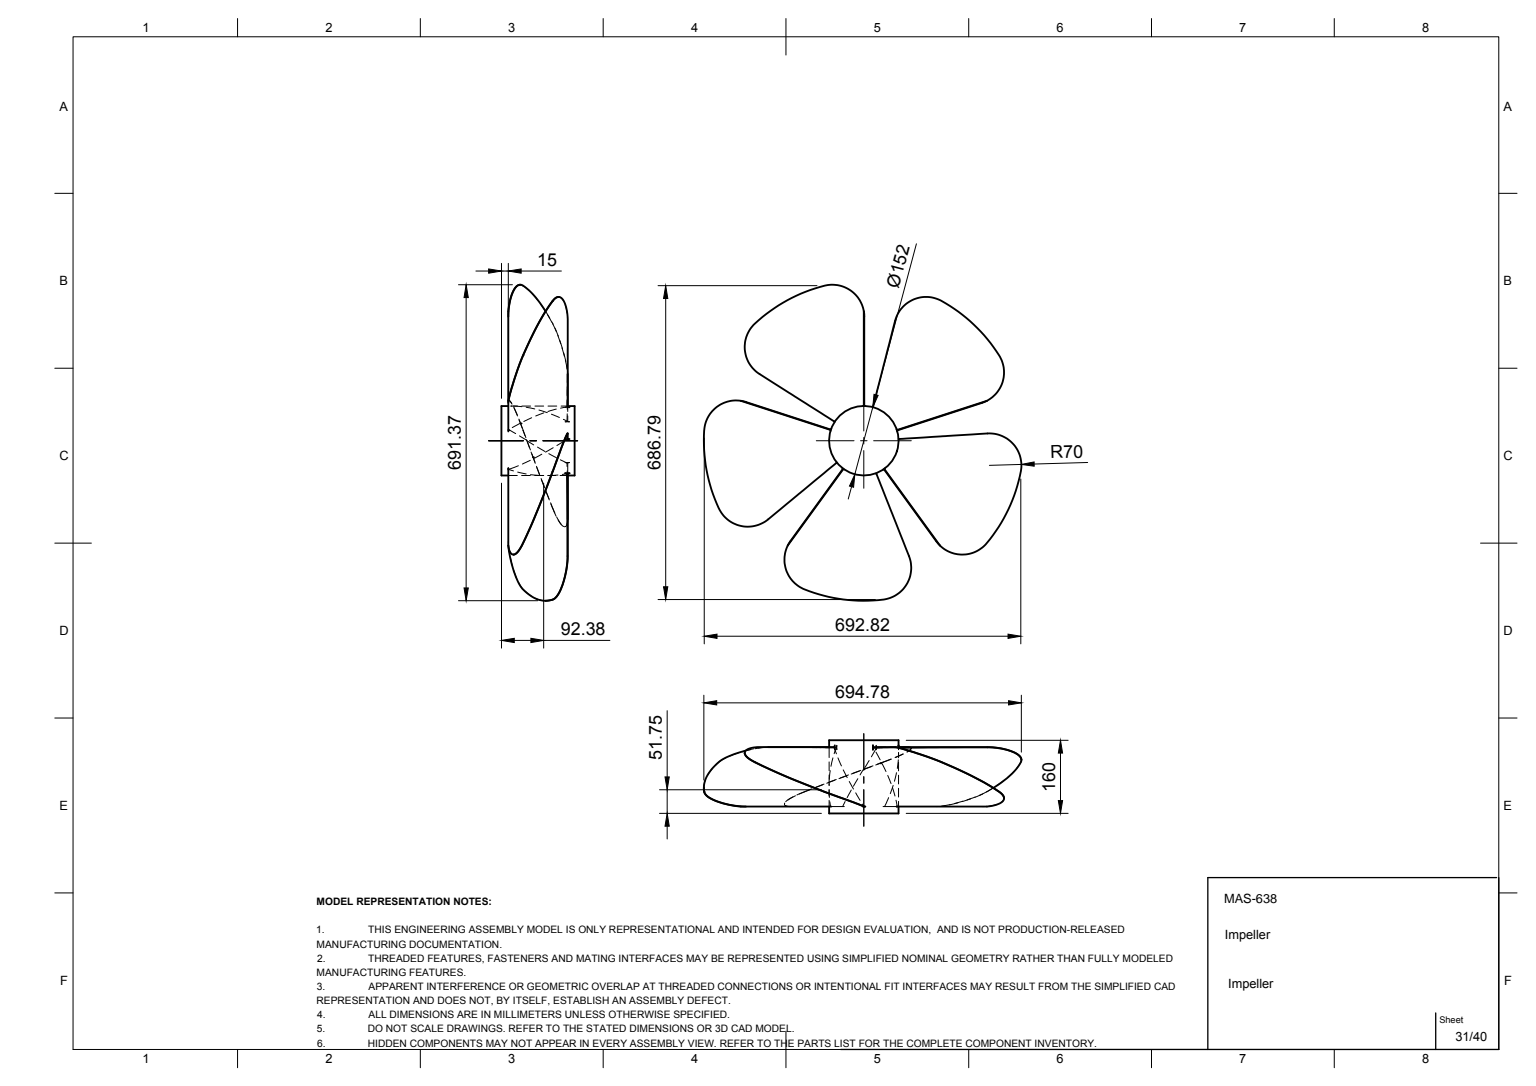
ISO-10303-21;
HEADER;
FILE_DESCRIPTION((''),'2;1');
FILE_NAME('Impeller.step','2026-10-09T12:00:21-07:00',(''),(''),'','','');
FILE_SCHEMA (('AUTOMOTIVE_DESIGN { 1 0 10303 214 3 1 1 }'));
ENDSEC;
DATA;
#10=MECHANICAL_DESIGN_GEOMETRIC_PRESENTATION_REPRESENTATION('',(#428),#10334);
#11=(
BOUNDED_CURVE()
B_SPLINE_CURVE(2,(#6661,#6662,#6663,#6664,#6665,#6666,#6667,#6668,#6669,
#6670,#6671,#6672,#6673,#6674,#6675),.UNSPECIFIED.,.F.,.F.)
B_SPLINE_CURVE_WITH_KNOTS((3,2,2,2,2,2,2,3),(0.24767599272402,0.275737101138962,
0.367649468185283,0.459561835231604,0.551474202277924,0.643386569324245,
0.735298936370566,0.744991303101576),.UNSPECIFIED.)
CURVE()
GEOMETRIC_REPRESENTATION_ITEM()
RATIONAL_B_SPLINE_CURVE((0.999547382800022,0.999674234156792,1.,0.998932974802372,
1.,0.998932974802372,1.,0.998932974802372,1.,0.998932974802372,1.,0.998932974802372,
1.,0.999887479782547,0.999798690587312))
REPRESENTATION_ITEM('')
) ;
#12=(
BOUNDED_CURVE()
B_SPLINE_CURVE(2,(#6842,#6843,#6844,#6845,#6846,#6847,#6848,#6849,#6850,
#6851,#6852,#6853,#6854,#6855,#6856),.UNSPECIFIED.,.F.,.F.)
B_SPLINE_CURVE_WITH_KNOTS((3,2,2,2,2,2,2,3),(0.0400825883740044,0.0441176470588235,
0.0588235294117647,0.0735294117647059,0.0882352941176471,0.102941176470588,
0.117647058823529,0.119652613204452),.UNSPECIFIED.)
CURVE()
GEOMETRIC_REPRESENTATION_ITEM()
RATIONAL_B_SPLINE_CURVE((0.999575116080077,0.999707225368239,1.,0.998932974802372,
1.,0.998932974802372,1.,0.998932974802372,1.,0.998932974802372,1.,0.998932974802372,
1.,0.999854481559943,0.999748654059601))
REPRESENTATION_ITEM('')
) ;
#13=(
BOUNDED_CURVE()
B_SPLINE_CURVE(2,(#7299,#7300,#7301,#7302,#7303,#7304,#7305,#7306,#7307,
#7308,#7309,#7310,#7311,#7312,#7313),.UNSPECIFIED.,.F.,.F.)
B_SPLINE_CURVE_WITH_KNOTS((3,2,2,2,2,2,2,3),(0.24767599272402,0.275737101138962,
0.367649468185283,0.459561835231604,0.551474202277924,0.643386569324245,
0.735298936370566,0.744991303101576),.UNSPECIFIED.)
CURVE()
GEOMETRIC_REPRESENTATION_ITEM()
RATIONAL_B_SPLINE_CURVE((0.999547382800022,0.999674234156792,1.,0.998932974802372,
1.,0.998932974802372,1.,0.998932974802372,1.,0.998932974802372,1.,0.998932974802372,
1.,0.999887479782547,0.999798690587312))
REPRESENTATION_ITEM('')
) ;
#14=(
BOUNDED_CURVE()
B_SPLINE_CURVE(2,(#7480,#7481,#7482,#7483,#7484,#7485,#7486,#7487,#7488,
#7489,#7490,#7491,#7492,#7493,#7494),.UNSPECIFIED.,.F.,.F.)
B_SPLINE_CURVE_WITH_KNOTS((3,2,2,2,2,2,2,3),(0.0400825883740044,0.0441176470588235,
0.0588235294117647,0.0735294117647059,0.0882352941176471,0.102941176470588,
0.117647058823529,0.119652613204452),.UNSPECIFIED.)
CURVE()
GEOMETRIC_REPRESENTATION_ITEM()
RATIONAL_B_SPLINE_CURVE((0.999575116080077,0.999707225368239,1.,0.998932974802372,
1.,0.998932974802372,1.,0.998932974802372,1.,0.998932974802372,1.,0.998932974802372,
1.,0.999854481559943,0.999748654059601))
REPRESENTATION_ITEM('')
) ;
#15=(
BOUNDED_CURVE()
B_SPLINE_CURVE(2,(#7937,#7938,#7939,#7940,#7941,#7942,#7943,#7944,#7945,
#7946,#7947,#7948,#7949,#7950,#7951),.UNSPECIFIED.,.F.,.F.)
B_SPLINE_CURVE_WITH_KNOTS((3,2,2,2,2,2,2,3),(0.24767599272402,0.275737101138962,
0.367649468185283,0.459561835231604,0.551474202277924,0.643386569324245,
0.735298936370566,0.744991303101576),.UNSPECIFIED.)
CURVE()
GEOMETRIC_REPRESENTATION_ITEM()
RATIONAL_B_SPLINE_CURVE((0.999547382800022,0.999674234156792,1.,0.998932974802372,
1.,0.998932974802372,1.,0.998932974802372,1.,0.998932974802372,1.,0.998932974802372,
1.,0.999887479782547,0.999798690587312))
REPRESENTATION_ITEM('')
) ;
#16=(
BOUNDED_CURVE()
B_SPLINE_CURVE(2,(#8118,#8119,#8120,#8121,#8122,#8123,#8124,#8125,#8126,
#8127,#8128,#8129,#8130,#8131,#8132),.UNSPECIFIED.,.F.,.F.)
B_SPLINE_CURVE_WITH_KNOTS((3,2,2,2,2,2,2,3),(0.0400825883740044,0.0441176470588235,
0.0588235294117647,0.0735294117647059,0.0882352941176471,0.102941176470588,
0.117647058823529,0.119652613204452),.UNSPECIFIED.)
CURVE()
GEOMETRIC_REPRESENTATION_ITEM()
RATIONAL_B_SPLINE_CURVE((0.999575116080077,0.999707225368239,1.,0.998932974802372,
1.,0.998932974802372,1.,0.998932974802372,1.,0.998932974802372,1.,0.998932974802372,
1.,0.999854481559943,0.999748654059601))
REPRESENTATION_ITEM('')
) ;
#17=(
BOUNDED_CURVE()
B_SPLINE_CURVE(2,(#8574,#8575,#8576,#8577,#8578,#8579,#8580,#8581,#8582,
#8583,#8584,#8585,#8586,#8587,#8588),.UNSPECIFIED.,.F.,.F.)
B_SPLINE_CURVE_WITH_KNOTS((3,2,2,2,2,2,2,3),(0.24767599272402,0.275737101138962,
0.367649468185283,0.459561835231603,0.551474202277924,0.643386569324245,
0.735298936370566,0.744991303101576),.UNSPECIFIED.)
CURVE()
GEOMETRIC_REPRESENTATION_ITEM()
RATIONAL_B_SPLINE_CURVE((0.999547382800022,0.999674234156792,1.,0.998932974802372,
1.,0.998932974802372,1.,0.998932974802372,1.,0.998932974802372,1.,0.998932974802372,
1.,0.999887479782547,0.999798690587312))
REPRESENTATION_ITEM('')
) ;
#18=(
BOUNDED_CURVE()
B_SPLINE_CURVE(2,(#8755,#8756,#8757,#8758,#8759,#8760,#8761,#8762,#8763,
#8764,#8765,#8766,#8767,#8768,#8769),.UNSPECIFIED.,.F.,.F.)
B_SPLINE_CURVE_WITH_KNOTS((3,2,2,2,2,2,2,3),(0.0400825883740044,0.0441176470588235,
0.0588235294117647,0.0735294117647059,0.0882352941176471,0.102941176470588,
0.117647058823529,0.119652613204452),.UNSPECIFIED.)
CURVE()
GEOMETRIC_REPRESENTATION_ITEM()
RATIONAL_B_SPLINE_CURVE((0.999575116080077,0.999707225368239,1.,0.998932974802372,
1.,0.998932974802372,1.,0.998932974802372,1.,0.998932974802372,1.,0.998932974802372,
1.,0.999854481559943,0.999748654059601))
REPRESENTATION_ITEM('')
) ;
#19=(
BOUNDED_CURVE()
B_SPLINE_CURVE(2,(#9211,#9212,#9213,#9214,#9215,#9216,#9217,#9218,#9219,
#9220,#9221,#9222,#9223,#9224,#9225),.UNSPECIFIED.,.F.,.F.)
B_SPLINE_CURVE_WITH_KNOTS((3,2,2,2,2,2,2,3),(0.24767599272402,0.275737101138962,
0.367649468185283,0.459561835231604,0.551474202277924,0.643386569324245,
0.735298936370566,0.744991303101576),.UNSPECIFIED.)
CURVE()
GEOMETRIC_REPRESENTATION_ITEM()
RATIONAL_B_SPLINE_CURVE((0.999547382800022,0.999674234156792,1.,0.998932974802372,
1.,0.998932974802372,1.,0.998932974802372,1.,0.998932974802372,1.,0.998932974802372,
1.,0.999887479782547,0.999798690587312))
REPRESENTATION_ITEM('')
) ;
#20=(
BOUNDED_CURVE()
B_SPLINE_CURVE(2,(#9392,#9393,#9394,#9395,#9396,#9397,#9398,#9399,#9400,
#9401,#9402,#9403,#9404,#9405,#9406),.UNSPECIFIED.,.F.,.F.)
B_SPLINE_CURVE_WITH_KNOTS((3,2,2,2,2,2,2,3),(0.0400825883740044,0.0441176470588235,
0.0588235294117647,0.0735294117647059,0.0882352941176471,0.102941176470588,
0.117647058823529,0.119652613204452),.UNSPECIFIED.)
CURVE()
GEOMETRIC_REPRESENTATION_ITEM()
RATIONAL_B_SPLINE_CURVE((0.999575116080077,0.999707225368239,1.,0.998932974802372,
1.,0.998932974802372,1.,0.998932974802372,1.,0.998932974802372,1.,0.998932974802372,
1.,0.999854481559943,0.999748654059601))
REPRESENTATION_ITEM('')
) ;
#21=ELLIPSE('',#4098,37.7772650531372,35.8772408571367) ;
#22=ELLIPSE('',#4099,37.8497403828003,36.0198777791808) ;
#23=ELLIPSE('',#4107,36.8921420435166,34.215760038751) ;
#24=ELLIPSE('',#4108,36.1551251123153,32.8675469297647) ;
#25=ELLIPSE('',#4116,37.0958421669686,34.5946418749128) ;
#26=ELLIPSE('',#4117,37.8806839269163,36.0787426019938) ;
#27=ELLIPSE('',#4124,37.6579384286729,35.6509558139733) ;
#28=ELLIPSE('',#4125,37.3365253827658,35.0500856310496) ;
#29=ELLIPSE('',#4132,38.4895046711754,37.2427567220046) ;
#30=ELLIPSE('',#4133,37.7160972861981,35.7660825268951) ;
#31=(
BOUNDED_SURFACE()
B_SPLINE_SURFACE(1,2,((#6503,#6504,#6505,#6506,#6507,#6508,#6509,#6510,
#6511,#6512,#6513,#6514,#6515,#6516,#6517,#6518,#6519,#6520,#6521,#6522,
#6523,#6524,#6525),(#6526,#6527,#6528,#6529,#6530,#6531,#6532,#6533,#6534,
#6535,#6536,#6537,#6538,#6539,#6540,#6541,#6542,#6543,#6544,#6545,#6546,
#6547,#6548)),.UNSPECIFIED.,.F.,.F.,.F.)
B_SPLINE_SURFACE_WITH_KNOTS((2,2),(3,2,2,2,2,2,2,2,2,2,2,3),(0.,1.),(-1.033109709591E-7,
0.0147058823529412,0.0294117647058824,0.0441176470588235,0.0588235294117647,
0.0735294117647059,0.0882352941176471,0.102941176470588,0.117647058823529,
0.132352941176471,0.147058823529412,0.159998951452637),.UNSPECIFIED.)
GEOMETRIC_REPRESENTATION_ITEM()
RATIONAL_B_SPLINE_SURFACE(((1.00000001499212,0.998932967306364,1.,0.998932974802372,
1.,0.998932974802372,1.,0.998932974802372,1.,0.998932974802372,1.,0.998932974802372,
1.,0.998932974802372,1.,0.998932974802372,1.,0.998932974802372,1.,0.998932974802372,
1.,0.999061093906287,0.999774528647208),(1.00000001499212,0.998932967306364,
1.,0.998932974802372,1.,0.998932974802372,1.,0.998932974802372,1.,0.998932974802372,
1.,0.998932974802372,1.,0.998932974802372,1.,0.998932974802372,1.,0.998932974802372,
1.,0.998932974802372,1.,0.999061093906287,0.999774528647208)))
REPRESENTATION_ITEM('')
SURFACE()
) ;
#32=(
BOUNDED_SURFACE()
B_SPLINE_SURFACE(1,2,((#6692,#6693,#6694,#6695,#6696,#6697,#6698,#6699,
#6700,#6701,#6702,#6703,#6704,#6705,#6706,#6707,#6708,#6709,#6710,#6711,
#6712,#6713,#6714),(#6715,#6716,#6717,#6718,#6719,#6720,#6721,#6722,#6723,
#6724,#6725,#6726,#6727,#6728,#6729,#6730,#6731,#6732,#6733,#6734,#6735,
#6736,#6737)),.UNSPECIFIED.,.F.,.F.,.F.)
B_SPLINE_SURFACE_WITH_KNOTS((2,2),(3,2,2,2,2,2,2,2,2,2,2,3),(-2.12079707674176E-9,
1.),(-4.92610673029739E-10,0.0147058823529412,0.0294117647058824,0.0441176470588235,
0.0588235294117647,0.0735294117647059,0.0882352941176471,0.102941176470588,
0.117647058823529,0.132352941176471,0.147058823529412,0.159999479208712),
 .UNSPECIFIED.)
GEOMETRIC_REPRESENTATION_ITEM()
RATIONAL_B_SPLINE_SURFACE(((1.00000000007149,0.99893297476663,1.,0.998932974802372,
1.,0.998932974802372,1.,0.998932974802372,1.,0.998932974802372,1.,0.998932974802372,
1.,0.998932974802372,1.,0.998932974802372,1.,0.998932974802372,1.,0.998932974802372,
1.,0.999061055613513,0.999774586844051),(1.00000000007149,0.99893297476663,
1.,0.998932974802372,1.,0.998932974802372,1.,0.998932974802372,1.,0.998932974802372,
1.,0.998932974802372,1.,0.998932974802372,1.,0.998932974802372,1.,0.998932974802372,
1.,0.998932974802372,1.,0.999061055613513,0.999774586844051)))
REPRESENTATION_ITEM('')
SURFACE()
) ;
#33=(
BOUNDED_SURFACE()
B_SPLINE_SURFACE(3,2,((#6905,#6906,#6907),(#6908,#6909,#6910),(#6911,#6912,
#6913),(#6914,#6915,#6916),(#6917,#6918,#6919),(#6920,#6921,#6922),(#6923,
#6924,#6925),(#6926,#6927,#6928),(#6929,#6930,#6931),(#6932,#6933,#6934),
(#6935,#6936,#6937),(#6938,#6939,#6940),(#6941,#6942,#6943),(#6944,#6945,
#6946),(#6947,#6948,#6949),(#6950,#6951,#6952),(#6953,#6954,#6955),(#6956,
#6957,#6958),(#6959,#6960,#6961),(#6962,#6963,#6964),(#6965,#6966,#6967),
(#6968,#6969,#6970),(#6971,#6972,#6973),(#6974,#6975,#6976),(#6977,#6978,
#6979),(#6980,#6981,#6982),(#6983,#6984,#6985),(#6986,#6987,#6988),(#6989,
#6990,#6991),(#6992,#6993,#6994),(#6995,#6996,#6997),(#6998,#6999,#7000)),
 .UNSPECIFIED.,.F.,.F.,.F.)
B_SPLINE_SURFACE_WITH_KNOTS((4,2,2,2,2,2,2,2,2,2,2,2,2,2,2,4),(3,3),(0.0363322941033848,
0.0552795959345893,0.0647532468501916,0.0742268977657938,0.0837005486813961,
0.0931741995969984,0.102647850512601,0.112121501428203,0.121595152343805,
0.131068803259407,0.14054245417501,0.150016105090612,0.159489756006214,
0.168963406921816,0.178437057837419,0.187910708753021),(0.,1.),
 .UNSPECIFIED.)
GEOMETRIC_REPRESENTATION_ITEM()
RATIONAL_B_SPLINE_SURFACE(((1.,0.713723577868364,1.),(1.,0.713722445293404,
1.),(1.,0.713725662281373,1.),(1.,0.713724573699931,1.),(1.,0.71372208949302,
1.),(1.,0.713725723145716,1.),(1.,0.713725237219869,1.),(1.,0.713719633392001,
1.),(1.,0.713725477091233,1.),(1.,0.713724228403321,1.),(1.,0.713722641415878,
1.),(1.,0.713725747691194,1.),(1.,0.713724999814938,1.),(1.,0.713718882742839,
1.),(1.,0.713725607158444,1.),(1.,0.713723850204247,1.),(1.,0.713723140250565,
1.),(1.,0.713725729945787,1.),(1.,0.713724718679381,1.),(1.,0.713718072353828,
1.),(1.,0.713725695695606,1.),(1.,0.713723420086558,1.),(1.,0.713723588770072,
1.),(1.,0.71372566780113,1.),(1.,0.713718399163855,1.),(1.,0.713724843902384,
1.),(1.,0.713725741663279,1.),(1.,0.71372293985685,1.),(1.,0.713724004994082,
1.),(1.,0.713725560151496,1.),(1.,0.713723126093937,1.),(1.,0.713721352883454,
1.)))
REPRESENTATION_ITEM('')
SURFACE()
) ;
#34=(
BOUNDED_SURFACE()
B_SPLINE_SURFACE(3,2,((#7001,#7002,#7003),(#7004,#7005,#7006),(#7007,#7008,
#7009),(#7010,#7011,#7012),(#7013,#7014,#7015),(#7016,#7017,#7018),(#7019,
#7020,#7021),(#7022,#7023,#7024),(#7025,#7026,#7027),(#7028,#7029,#7030),
(#7031,#7032,#7033),(#7034,#7035,#7036),(#7037,#7038,#7039),(#7040,#7041,
#7042),(#7043,#7044,#7045),(#7046,#7047,#7048),(#7049,#7050,#7051),(#7052,
#7053,#7054),(#7055,#7056,#7057),(#7058,#7059,#7060),(#7061,#7062,#7063),
(#7064,#7065,#7066),(#7067,#7068,#7069),(#7070,#7071,#7072),(#7073,#7074,
#7075),(#7076,#7077,#7078),(#7079,#7080,#7081),(#7082,#7083,#7084),(#7085,
#7086,#7087),(#7088,#7089,#7090),(#7091,#7092,#7093),(#7094,#7095,#7096),
(#7097,#7098,#7099),(#7100,#7101,#7102),(#7103,#7104,#7105),(#7106,#7107,
#7108)),.UNSPECIFIED.,.F.,.F.,.F.)
B_SPLINE_SURFACE_WITH_KNOTS((4,2,2,2,2,2,2,2,2,2,2,2,2,2,2,2,2,4),(3,3),
(0.110192674671804,0.119968567976379,0.129744461280954,0.139520354585529,
0.149296247890104,0.159072141194679,0.168848034499254,0.178623927803829,
0.183511874456117,0.188399821108404,0.198175714412979,0.207951607717554,
0.217727501022129,0.227503394326704,0.23727928763128,0.247055180935855,
0.25683107424043,0.266606967545005),(0.,1.),.UNSPECIFIED.)
GEOMETRIC_REPRESENTATION_ITEM()
RATIONAL_B_SPLINE_SURFACE(((1.,0.717557917014249,1.),(1.,0.717557424551413,
1.),(1.,0.717562701205404,1.),(1.,0.717561702803317,1.),(1.,0.717559005659748,
1.),(1.,0.717563327413176,1.),(1.,0.71756229100789,1.),(1.,0.717553816681041,
1.),(1.,0.717563248342644,1.),(1.,0.717560128438615,1.),(1.,0.717560865936392,
1.),(1.,0.717563079897794,1.),(1.,0.717555152418623,1.),(1.,0.717562714682237,
1.),(1.,0.717563278057682,1.),(1.,0.717559267705998,1.),(1.,0.717558273919951,
1.),(1.,0.717561484503512,1.),(1.,0.717562276054518,1.),(1.,0.717562227727252,
1.),(1.,0.717558058641825,1.),(1.,0.717563288924202,1.),(1.,0.717562675856868,
1.),(1.,0.717554973696268,1.),(1.,0.717563128955385,1.),(1.,0.717560719068534,
1.),(1.,0.717560347129028,1.),(1.,0.717563217875631,1.),(1.,0.717554301335648,
1.),(1.,0.717562479166741,1.),(1.,0.717563325990987,1.),(1.,0.717558566722815,
1.),(1.,0.717561980919154,1.),(1.,0.717562507369476,1.),(1.,0.717555378743213,
1.),(1.,0.717566078456111,1.)))
REPRESENTATION_ITEM('')
SURFACE()
) ;
#35=(
BOUNDED_SURFACE()
B_SPLINE_SURFACE(1,2,((#7141,#7142,#7143,#7144,#7145,#7146,#7147,#7148,
#7149,#7150,#7151,#7152,#7153,#7154,#7155,#7156,#7157,#7158,#7159,#7160,
#7161,#7162,#7163),(#7164,#7165,#7166,#7167,#7168,#7169,#7170,#7171,#7172,
#7173,#7174,#7175,#7176,#7177,#7178,#7179,#7180,#7181,#7182,#7183,#7184,
#7185,#7186)),.UNSPECIFIED.,.F.,.F.,.F.)
B_SPLINE_SURFACE_WITH_KNOTS((2,2),(3,2,2,2,2,2,2,2,2,2,2,3),(0.,1.),(-1.03310890689824E-7,
0.0147058823529412,0.0294117647058824,0.0441176470588235,0.0588235294117647,
0.0735294117647059,0.0882352941176471,0.102941176470588,0.117647058823529,
0.132352941176471,0.147058823529412,0.159998951452637),.UNSPECIFIED.)
GEOMETRIC_REPRESENTATION_ITEM()
RATIONAL_B_SPLINE_SURFACE(((1.00000001499211,0.99893296730637,1.,0.998932974802372,
1.,0.998932974802372,1.,0.998932974802372,1.,0.998932974802372,1.,0.998932974802372,
1.,0.998932974802372,1.,0.998932974802372,1.,0.998932974802372,1.,0.998932974802372,
1.,0.999061093906287,0.999774528647208),(1.00000001499211,0.99893296730637,
1.,0.998932974802372,1.,0.998932974802372,1.,0.998932974802372,1.,0.998932974802372,
1.,0.998932974802372,1.,0.998932974802372,1.,0.998932974802372,1.,0.998932974802372,
1.,0.998932974802372,1.,0.999061093906287,0.999774528647208)))
REPRESENTATION_ITEM('')
SURFACE()
) ;
#36=(
BOUNDED_SURFACE()
B_SPLINE_SURFACE(1,2,((#7330,#7331,#7332,#7333,#7334,#7335,#7336,#7337,
#7338,#7339,#7340,#7341,#7342,#7343,#7344,#7345,#7346,#7347,#7348,#7349,
#7350,#7351,#7352),(#7353,#7354,#7355,#7356,#7357,#7358,#7359,#7360,#7361,
#7362,#7363,#7364,#7365,#7366,#7367,#7368,#7369,#7370,#7371,#7372,#7373,
#7374,#7375)),.UNSPECIFIED.,.F.,.F.,.F.)
B_SPLINE_SURFACE_WITH_KNOTS((2,2),(3,2,2,2,2,2,2,2,2,2,2,3),(-2.12079713977352E-9,
1.),(-4.92610737156842E-10,0.0147058823529412,0.0294117647058824,0.0441176470588235,
0.0588235294117647,0.0735294117647059,0.0882352941176471,0.102941176470588,
0.117647058823529,0.132352941176471,0.147058823529412,0.159999479208712),
 .UNSPECIFIED.)
GEOMETRIC_REPRESENTATION_ITEM()
RATIONAL_B_SPLINE_SURFACE(((1.00000000007149,0.99893297476663,1.,0.998932974802372,
1.,0.998932974802372,1.,0.998932974802372,1.,0.998932974802372,1.,0.998932974802372,
1.,0.998932974802372,1.,0.998932974802372,1.,0.998932974802372,1.,0.998932974802372,
1.,0.999061055613513,0.999774586844051),(1.00000000007149,0.99893297476663,
1.,0.998932974802372,1.,0.998932974802372,1.,0.998932974802372,1.,0.998932974802372,
1.,0.998932974802372,1.,0.998932974802372,1.,0.998932974802372,1.,0.998932974802372,
1.,0.998932974802372,1.,0.999061055613513,0.999774586844051)))
REPRESENTATION_ITEM('')
SURFACE()
) ;
#37=(
BOUNDED_SURFACE()
B_SPLINE_SURFACE(3,2,((#7542,#7543,#7544),(#7545,#7546,#7547),(#7548,#7549,
#7550),(#7551,#7552,#7553),(#7554,#7555,#7556),(#7557,#7558,#7559),(#7560,
#7561,#7562),(#7563,#7564,#7565),(#7566,#7567,#7568),(#7569,#7570,#7571),
(#7572,#7573,#7574),(#7575,#7576,#7577),(#7578,#7579,#7580),(#7581,#7582,
#7583),(#7584,#7585,#7586),(#7587,#7588,#7589),(#7590,#7591,#7592),(#7593,
#7594,#7595),(#7596,#7597,#7598),(#7599,#7600,#7601),(#7602,#7603,#7604),
(#7605,#7606,#7607),(#7608,#7609,#7610),(#7611,#7612,#7613),(#7614,#7615,
#7616),(#7617,#7618,#7619),(#7620,#7621,#7622),(#7623,#7624,#7625),(#7626,
#7627,#7628),(#7629,#7630,#7631),(#7632,#7633,#7634),(#7635,#7636,#7637)),
 .UNSPECIFIED.,.F.,.F.,.F.)
B_SPLINE_SURFACE_WITH_KNOTS((4,2,2,2,2,2,2,2,2,2,2,2,2,2,2,4),(3,3),(0.0363322941033848,
0.0552795959345893,0.0647532468501916,0.0742268977657939,0.0837005486813961,
0.0931741995969984,0.102647850512601,0.112121501428203,0.121595152343805,
0.131068803259407,0.14054245417501,0.150016105090612,0.159489756006214,
0.168963406921816,0.178437057837419,0.187910708753021),(0.,1.),
 .UNSPECIFIED.)
GEOMETRIC_REPRESENTATION_ITEM()
RATIONAL_B_SPLINE_SURFACE(((1.,0.713723577868379,1.),(1.,0.71372244527551,
1.),(1.,0.713725662305176,1.),(1.,0.713724573687971,1.),(1.,0.713722089554594,
1.),(1.,0.713725723084203,1.),(1.,0.713725237316385,1.),(1.,0.71371963329541,
1.),(1.,0.713725477094868,1.),(1.,0.713724228399586,1.),(1.,0.713722641372577,
1.),(1.,0.713725747734493,1.),(1.,0.713724999822108,1.),(1.,0.713718882735633,
1.),(1.,0.713725607168583,1.),(1.,0.713723850194029,1.),(1.,0.713723140179135,
1.),(1.,0.713725730017236,1.),(1.,0.713724718641669,1.),(1.,0.713718072391505,
1.),(1.,0.713725695688412,1.),(1.,0.713723420093739,1.),(1.,0.713723588714817,
1.),(1.,0.71372566785642,1.),(1.,0.713718399180568,1.),(1.,0.713724843885739,
1.),(1.,0.713725741676244,1.),(1.,0.713722939843865,1.),(1.,0.71372400500128,
1.),(1.,0.71372556014432,1.),(1.,0.713723126099315,1.),(1.,0.713721352883477,
1.)))
REPRESENTATION_ITEM('')
SURFACE()
) ;
#38=(
BOUNDED_SURFACE()
B_SPLINE_SURFACE(3,2,((#7638,#7639,#7640),(#7641,#7642,#7643),(#7644,#7645,
#7646),(#7647,#7648,#7649),(#7650,#7651,#7652),(#7653,#7654,#7655),(#7656,
#7657,#7658),(#7659,#7660,#7661),(#7662,#7663,#7664),(#7665,#7666,#7667),
(#7668,#7669,#7670),(#7671,#7672,#7673),(#7674,#7675,#7676),(#7677,#7678,
#7679),(#7680,#7681,#7682),(#7683,#7684,#7685),(#7686,#7687,#7688),(#7689,
#7690,#7691),(#7692,#7693,#7694),(#7695,#7696,#7697),(#7698,#7699,#7700),
(#7701,#7702,#7703),(#7704,#7705,#7706),(#7707,#7708,#7709),(#7710,#7711,
#7712),(#7713,#7714,#7715),(#7716,#7717,#7718),(#7719,#7720,#7721),(#7722,
#7723,#7724),(#7725,#7726,#7727),(#7728,#7729,#7730),(#7731,#7732,#7733),
(#7734,#7735,#7736),(#7737,#7738,#7739),(#7740,#7741,#7742),(#7743,#7744,
#7745)),.UNSPECIFIED.,.F.,.F.,.F.)
B_SPLINE_SURFACE_WITH_KNOTS((4,2,2,2,2,2,2,2,2,2,2,2,2,2,2,2,2,4),(3,3),
(0.110192674671804,0.119968567976379,0.129744461280954,0.139520354585529,
0.149296247890104,0.159072141194679,0.168848034499254,0.178623927803829,
0.183511874456117,0.188399821108404,0.198175714412979,0.207951607717554,
0.21772750102213,0.227503394326705,0.23727928763128,0.247055180935855,0.25683107424043,
0.266606967545005),(0.,1.),.UNSPECIFIED.)
GEOMETRIC_REPRESENTATION_ITEM()
RATIONAL_B_SPLINE_SURFACE(((1.,0.717557917014237,1.),(1.,0.717557424537029,
1.),(1.,0.717562701224584,1.),(1.,0.717561702784131,1.),(1.,0.717559005677598,
1.),(1.,0.717563327395298,1.),(1.,0.71756229102355,1.),(1.,0.717553816665384,
1.),(1.,0.717563248345556,1.),(1.,0.717560128435701,1.),(1.,0.717560865922022,
1.),(1.,0.717563079912224,1.),(1.,0.717555152410577,1.),(1.,0.717562714690268,
1.),(1.,0.71756327807233,1.),(1.,0.717559267698649,1.),(1.,0.71755827388903,
1.),(1.,0.717561484534412,1.),(1.,0.717562276061397,1.),(1.,0.717562227713511,
1.),(1.,0.717558058653909,1.),(1.,0.717563288912114,1.),(1.,0.717562675824823,
1.),(1.,0.717554973728334,1.),(1.,0.717563128966192,1.),(1.,0.717560719057696,
1.),(1.,0.717560347146644,1.),(1.,0.71756321785806,1.),(1.,0.717554301337103,
1.),(1.,0.717562479165266,1.),(1.,0.717563326012811,1.),(1.,0.717558566701041,
1.),(1.,0.717561980953627,1.),(1.,0.717562507334971,1.),(1.,0.717555378769111,
1.),(1.,0.717566078456109,1.)))
REPRESENTATION_ITEM('')
SURFACE()
) ;
#39=(
BOUNDED_SURFACE()
B_SPLINE_SURFACE(1,2,((#7779,#7780,#7781,#7782,#7783,#7784,#7785,#7786,
#7787,#7788,#7789,#7790,#7791,#7792,#7793,#7794,#7795,#7796,#7797,#7798,
#7799,#7800,#7801),(#7802,#7803,#7804,#7805,#7806,#7807,#7808,#7809,#7810,
#7811,#7812,#7813,#7814,#7815,#7816,#7817,#7818,#7819,#7820,#7821,#7822,
#7823,#7824)),.UNSPECIFIED.,.F.,.F.,.F.)
B_SPLINE_SURFACE_WITH_KNOTS((2,2),(3,2,2,2,2,2,2,2,2,2,2,3),(0.,1.),(-1.03311088010868E-7,
0.0147058823529412,0.0294117647058824,0.0441176470588235,0.0588235294117647,
0.0735294117647059,0.0882352941176471,0.102941176470588,0.117647058823529,
0.132352941176471,0.147058823529412,0.159998951452637),.UNSPECIFIED.)
GEOMETRIC_REPRESENTATION_ITEM()
RATIONAL_B_SPLINE_SURFACE(((1.00000001499214,0.998932967306356,1.,0.998932974802372,
1.,0.998932974802372,1.,0.998932974802372,1.,0.998932974802372,1.,0.998932974802372,
1.,0.998932974802372,1.,0.998932974802372,1.,0.998932974802372,1.,0.998932974802372,
1.,0.999061093906287,0.999774528647208),(1.00000001499214,0.998932967306356,
1.,0.998932974802372,1.,0.998932974802372,1.,0.998932974802372,1.,0.998932974802372,
1.,0.998932974802372,1.,0.998932974802372,1.,0.998932974802372,1.,0.998932974802372,
1.,0.998932974802372,1.,0.999061093906287,0.999774528647208)))
REPRESENTATION_ITEM('')
SURFACE()
) ;
#40=(
BOUNDED_SURFACE()
B_SPLINE_SURFACE(1,2,((#7968,#7969,#7970,#7971,#7972,#7973,#7974,#7975,
#7976,#7977,#7978,#7979,#7980,#7981,#7982,#7983,#7984,#7985,#7986,#7987,
#7988,#7989,#7990),(#7991,#7992,#7993,#7994,#7995,#7996,#7997,#7998,#7999,
#8000,#8001,#8002,#8003,#8004,#8005,#8006,#8007,#8008,#8009,#8010,#8011,
#8012,#8013)),.UNSPECIFIED.,.F.,.F.,.F.)
B_SPLINE_SURFACE_WITH_KNOTS((2,2),(3,2,2,2,2,2,2,2,2,2,2,3),(-2.12079722094204E-9,
1.),(-4.92610683626735E-10,0.0147058823529412,0.0294117647058824,0.0441176470588235,
0.0588235294117647,0.0735294117647059,0.0882352941176471,0.102941176470588,
0.117647058823529,0.132352941176471,0.147058823529412,0.159999479208712),
 .UNSPECIFIED.)
GEOMETRIC_REPRESENTATION_ITEM()
RATIONAL_B_SPLINE_SURFACE(((1.00000000007149,0.99893297476663,1.,0.998932974802373,
1.,0.998932974802373,1.,0.998932974802373,1.,0.998932974802373,1.,0.998932974802373,
1.,0.998932974802373,1.,0.998932974802373,1.,0.998932974802373,1.,0.998932974802373,
1.,0.999061055613513,0.999774586844051),(1.00000000007149,0.99893297476663,
1.,0.998932974802372,1.,0.998932974802372,1.,0.998932974802372,1.,0.998932974802372,
1.,0.998932974802372,1.,0.998932974802372,1.,0.998932974802372,1.,0.998932974802372,
1.,0.998932974802372,1.,0.999061055613513,0.999774586844051)))
REPRESENTATION_ITEM('')
SURFACE()
) ;
#41=(
BOUNDED_SURFACE()
B_SPLINE_SURFACE(3,2,((#8180,#8181,#8182),(#8183,#8184,#8185),(#8186,#8187,
#8188),(#8189,#8190,#8191),(#8192,#8193,#8194),(#8195,#8196,#8197),(#8198,
#8199,#8200),(#8201,#8202,#8203),(#8204,#8205,#8206),(#8207,#8208,#8209),
(#8210,#8211,#8212),(#8213,#8214,#8215),(#8216,#8217,#8218),(#8219,#8220,
#8221),(#8222,#8223,#8224),(#8225,#8226,#8227),(#8228,#8229,#8230),(#8231,
#8232,#8233),(#8234,#8235,#8236),(#8237,#8238,#8239),(#8240,#8241,#8242),
(#8243,#8244,#8245),(#8246,#8247,#8248),(#8249,#8250,#8251),(#8252,#8253,
#8254),(#8255,#8256,#8257),(#8258,#8259,#8260),(#8261,#8262,#8263),(#8264,
#8265,#8266),(#8267,#8268,#8269),(#8270,#8271,#8272),(#8273,#8274,#8275)),
 .UNSPECIFIED.,.F.,.F.,.F.)
B_SPLINE_SURFACE_WITH_KNOTS((4,2,2,2,2,2,2,2,2,2,2,2,2,2,2,4),(3,3),(0.0363322941033848,
0.0552795959345893,0.0647532468501916,0.0742268977657939,0.0837005486813961,
0.0931741995969984,0.102647850512601,0.112121501428203,0.121595152343805,
0.131068803259407,0.14054245417501,0.150016105090612,0.159489756006214,
0.168963406921816,0.178437057837419,0.187910708753021),(0.,1.),
 .UNSPECIFIED.)
GEOMETRIC_REPRESENTATION_ITEM()
RATIONAL_B_SPLINE_SURFACE(((1.,0.713723577868358,1.),(1.,0.713722445286561,
1.),(1.,0.713725662290464,1.),(1.,0.713724573695348,1.),(1.,0.713722089511115,
1.),(1.,0.713725723127692,1.),(1.,0.713725237333952,1.),(1.,0.713719633277867,
1.),(1.,0.713725477122433,1.),(1.,0.713724228372051,1.),(1.,0.713722641353114,
1.),(1.,0.713725747753947,1.),(1.,0.713724999842608,1.),(1.,0.713718882715111,
1.),(1.,0.713725607168934,1.),(1.,0.713723850193677,1.),(1.,0.713723140210728,
1.),(1.,0.71372572998564,1.),(1.,0.713724718629055,1.),(1.,0.713718072404138,
1.),(1.,0.713725695723828,1.),(1.,0.713723420058332,1.),(1.,0.713723588633586,
1.),(1.,0.713725667937673,1.),(1.,0.713718399179848,1.),(1.,0.713724843886423,
1.),(1.,0.713725741689566,1.),(1.,0.713722939830535,1.),(1.,0.713724005000408,
1.),(1.,0.713725560145201,1.),(1.,0.71372312609865,1.),(1.,0.713721352883471,
1.)))
REPRESENTATION_ITEM('')
SURFACE()
) ;
#42=(
BOUNDED_SURFACE()
B_SPLINE_SURFACE(3,2,((#8276,#8277,#8278),(#8279,#8280,#8281),(#8282,#8283,
#8284),(#8285,#8286,#8287),(#8288,#8289,#8290),(#8291,#8292,#8293),(#8294,
#8295,#8296),(#8297,#8298,#8299),(#8300,#8301,#8302),(#8303,#8304,#8305),
(#8306,#8307,#8308),(#8309,#8310,#8311),(#8312,#8313,#8314),(#8315,#8316,
#8317),(#8318,#8319,#8320),(#8321,#8322,#8323),(#8324,#8325,#8326),(#8327,
#8328,#8329),(#8330,#8331,#8332),(#8333,#8334,#8335),(#8336,#8337,#8338),
(#8339,#8340,#8341),(#8342,#8343,#8344),(#8345,#8346,#8347),(#8348,#8349,
#8350),(#8351,#8352,#8353),(#8354,#8355,#8356),(#8357,#8358,#8359),(#8360,
#8361,#8362),(#8363,#8364,#8365),(#8366,#8367,#8368),(#8369,#8370,#8371),
(#8372,#8373,#8374),(#8375,#8376,#8377),(#8378,#8379,#8380),(#8381,#8382,
#8383)),.UNSPECIFIED.,.F.,.F.,.F.)
B_SPLINE_SURFACE_WITH_KNOTS((4,2,2,2,2,2,2,2,2,2,2,2,2,2,2,2,2,4),(3,3),
(0.110192674671804,0.119968567976379,0.129744461280954,0.139520354585529,
0.149296247890104,0.159072141194679,0.168848034499254,0.178623927803829,
0.183511874456117,0.188399821108404,0.198175714412979,0.207951607717554,
0.21772750102213,0.227503394326705,0.23727928763128,0.247055180935855,0.25683107424043,
0.266606967545005),(0.,1.),.UNSPECIFIED.)
GEOMETRIC_REPRESENTATION_ITEM()
RATIONAL_B_SPLINE_SURFACE(((1.,0.717557917014254,1.),(1.,0.717557424547014,
1.),(1.,0.717562701211253,1.),(1.,0.717561702797474,1.),(1.,0.717559005695462,
1.),(1.,0.717563327377434,1.),(1.,0.71756229099605,1.),(1.,0.717553816692872,
1.),(1.,0.71756324839199,1.),(1.,0.717560128389276,1.),(1.,0.717560865954089,
1.),(1.,0.717563079880128,1.),(1.,0.717555152412765,1.),(1.,0.717562714688071,
1.),(1.,0.717563278030574,1.),(1.,0.717559267719585,1.),(1.,0.717558273903889,
1.),(1.,0.717561484519553,1.),(1.,0.717562276060567,1.),(1.,0.717562227715156,
1.),(1.,0.717558058640351,1.),(1.,0.717563288925658,1.),(1.,0.717562675824091,
1.),(1.,0.717554973729067,1.),(1.,0.717563128925084,1.),(1.,0.717560719098766,
1.),(1.,0.717560347141852,1.),(1.,0.717563217862797,1.),(1.,0.71755430134791,
1.),(1.,0.717562479154465,1.),(1.,0.717563326066472,1.),(1.,0.717558566647358,
1.),(1.,0.717561980967755,1.),(1.,0.717562507320847,1.),(1.,0.717555378779752,
1.),(1.,0.7175660784561,1.)))
REPRESENTATION_ITEM('')
SURFACE()
) ;
#43=(
BOUNDED_SURFACE()
B_SPLINE_SURFACE(1,2,((#8416,#8417,#8418,#8419,#8420,#8421,#8422,#8423,
#8424,#8425,#8426,#8427,#8428,#8429,#8430,#8431,#8432,#8433,#8434,#8435,
#8436,#8437,#8438),(#8439,#8440,#8441,#8442,#8443,#8444,#8445,#8446,#8447,
#8448,#8449,#8450,#8451,#8452,#8453,#8454,#8455,#8456,#8457,#8458,#8459,
#8460,#8461)),.UNSPECIFIED.,.F.,.F.,.F.)
B_SPLINE_SURFACE_WITH_KNOTS((2,2),(3,2,2,2,2,2,2,2,2,2,2,3),(0.,1.),(-1.03311007440564E-7,
0.0147058823529412,0.0294117647058824,0.0441176470588235,0.0588235294117647,
0.0735294117647059,0.0882352941176471,0.102941176470588,0.117647058823529,
0.132352941176471,0.147058823529412,0.159998951452637),.UNSPECIFIED.)
GEOMETRIC_REPRESENTATION_ITEM()
RATIONAL_B_SPLINE_SURFACE(((1.00000001499213,0.998932967306362,1.,0.998932974802372,
1.,0.998932974802372,1.,0.998932974802372,1.,0.998932974802372,1.,0.998932974802372,
1.,0.998932974802372,1.,0.998932974802372,1.,0.998932974802372,1.,0.998932974802372,
1.,0.999061093906287,0.999774528647208),(1.00000001499213,0.998932967306362,
1.,0.998932974802372,1.,0.998932974802372,1.,0.998932974802372,1.,0.998932974802372,
1.,0.998932974802372,1.,0.998932974802372,1.,0.998932974802372,1.,0.998932974802372,
1.,0.998932974802372,1.,0.999061093906287,0.999774528647208)))
REPRESENTATION_ITEM('')
SURFACE()
) ;
#44=(
BOUNDED_SURFACE()
B_SPLINE_SURFACE(1,2,((#8605,#8606,#8607,#8608,#8609,#8610,#8611,#8612,
#8613,#8614,#8615,#8616,#8617,#8618,#8619,#8620,#8621,#8622,#8623,#8624,
#8625,#8626,#8627),(#8628,#8629,#8630,#8631,#8632,#8633,#8634,#8635,#8636,
#8637,#8638,#8639,#8640,#8641,#8642,#8643,#8644,#8645,#8646,#8647,#8648,
#8649,#8650)),.UNSPECIFIED.,.F.,.F.,.F.)
B_SPLINE_SURFACE_WITH_KNOTS((2,2),(3,2,2,2,2,2,2,2,2,2,2,3),(-2.12079720203126E-9,
1.),(-4.92610607495987E-10,0.0147058823529412,0.0294117647058824,0.0441176470588235,
0.0588235294117647,0.0735294117647059,0.0882352941176471,0.102941176470588,
0.117647058823529,0.132352941176471,0.147058823529412,0.159999479208712),
 .UNSPECIFIED.)
GEOMETRIC_REPRESENTATION_ITEM()
RATIONAL_B_SPLINE_SURFACE(((1.00000000007148,0.998932974766629,1.,0.998932974802372,
1.,0.998932974802372,1.,0.998932974802372,1.,0.998932974802372,1.,0.998932974802372,
1.,0.998932974802372,1.,0.998932974802372,1.,0.998932974802372,1.,0.998932974802372,
1.,0.999061055613513,0.999774586844051),(1.00000000007149,0.99893297476663,
1.,0.998932974802372,1.,0.998932974802372,1.,0.998932974802372,1.,0.998932974802372,
1.,0.998932974802372,1.,0.998932974802372,1.,0.998932974802372,1.,0.998932974802372,
1.,0.998932974802372,1.,0.999061055613513,0.999774586844051)))
REPRESENTATION_ITEM('')
SURFACE()
) ;
#45=(
BOUNDED_SURFACE()
B_SPLINE_SURFACE(3,2,((#8817,#8818,#8819),(#8820,#8821,#8822),(#8823,#8824,
#8825),(#8826,#8827,#8828),(#8829,#8830,#8831),(#8832,#8833,#8834),(#8835,
#8836,#8837),(#8838,#8839,#8840),(#8841,#8842,#8843),(#8844,#8845,#8846),
(#8847,#8848,#8849),(#8850,#8851,#8852),(#8853,#8854,#8855),(#8856,#8857,
#8858),(#8859,#8860,#8861),(#8862,#8863,#8864),(#8865,#8866,#8867),(#8868,
#8869,#8870),(#8871,#8872,#8873),(#8874,#8875,#8876),(#8877,#8878,#8879),
(#8880,#8881,#8882),(#8883,#8884,#8885),(#8886,#8887,#8888),(#8889,#8890,
#8891),(#8892,#8893,#8894),(#8895,#8896,#8897),(#8898,#8899,#8900),(#8901,
#8902,#8903),(#8904,#8905,#8906),(#8907,#8908,#8909),(#8910,#8911,#8912)),
 .UNSPECIFIED.,.F.,.F.,.F.)
B_SPLINE_SURFACE_WITH_KNOTS((4,2,2,2,2,2,2,2,2,2,2,2,2,2,2,4),(3,3),(0.0363322941033848,
0.0552795959345893,0.0647532468501916,0.0742268977657938,0.0837005486813961,
0.0931741995969983,0.102647850512601,0.112121501428203,0.121595152343805,
0.131068803259407,0.14054245417501,0.150016105090612,0.159489756006214,
0.168963406921816,0.178437057837419,0.187910708753021),(0.,1.),
 .UNSPECIFIED.)
GEOMETRIC_REPRESENTATION_ITEM()
RATIONAL_B_SPLINE_SURFACE(((1.,0.713723577868383,1.),(1.,0.713722445236779,
1.),(1.,0.713725662356741,1.),(1.,0.713724573662225,1.),(1.,0.713722089533019,
1.),(1.,0.713725723105761,1.),(1.,0.713725237328151,1.),(1.,0.713719633283652,
1.),(1.,0.713725477073128,1.),(1.,0.713724228421365,1.),(1.,0.713722641394657,
1.),(1.,0.713725747712396,1.),(1.,0.713724999816327,1.),(1.,0.713718882741423,
1.),(1.,0.713725607146823,1.),(1.,0.713723850215792,1.),(1.,0.713723140163847,
1.),(1.,0.71372573003249,1.),(1.,0.713724718644484,1.),(1.,0.71371807238871,
1.),(1.,0.713725695693675,1.),(1.,0.713723420088484,1.),(1.,0.713723588715348,
1.),(1.,0.713725667855899,1.),(1.,0.713718399201785,1.),(1.,0.713724843864469,
1.),(1.,0.71372574166801,1.),(1.,0.713722939852113,1.),(1.,0.71372400503284,
1.),(1.,0.713725560112773,1.),(1.,0.713723126123005,1.),(1.,0.713721352883481,
1.)))
REPRESENTATION_ITEM('')
SURFACE()
) ;
#46=(
BOUNDED_SURFACE()
B_SPLINE_SURFACE(3,2,((#8913,#8914,#8915),(#8916,#8917,#8918),(#8919,#8920,
#8921),(#8922,#8923,#8924),(#8925,#8926,#8927),(#8928,#8929,#8930),(#8931,
#8932,#8933),(#8934,#8935,#8936),(#8937,#8938,#8939),(#8940,#8941,#8942),
(#8943,#8944,#8945),(#8946,#8947,#8948),(#8949,#8950,#8951),(#8952,#8953,
#8954),(#8955,#8956,#8957),(#8958,#8959,#8960),(#8961,#8962,#8963),(#8964,
#8965,#8966),(#8967,#8968,#8969),(#8970,#8971,#8972),(#8973,#8974,#8975),
(#8976,#8977,#8978),(#8979,#8980,#8981),(#8982,#8983,#8984),(#8985,#8986,
#8987),(#8988,#8989,#8990),(#8991,#8992,#8993),(#8994,#8995,#8996),(#8997,
#8998,#8999),(#9000,#9001,#9002),(#9003,#9004,#9005),(#9006,#9007,#9008),
(#9009,#9010,#9011),(#9012,#9013,#9014),(#9015,#9016,#9017),(#9018,#9019,
#9020)),.UNSPECIFIED.,.F.,.F.,.F.)
B_SPLINE_SURFACE_WITH_KNOTS((4,2,2,2,2,2,2,2,2,2,2,2,2,2,2,2,2,4),(3,3),
(0.110192674671804,0.119968567976379,0.129744461280954,0.139520354585529,
0.149296247890104,0.159072141194679,0.168848034499254,0.178623927803829,
0.183511874456117,0.188399821108404,0.198175714412979,0.207951607717554,
0.217727501022129,0.227503394326704,0.23727928763128,0.247055180935855,
0.25683107424043,0.266606967545005),(0.,1.00023388176495),.UNSPECIFIED.)
GEOMETRIC_REPRESENTATION_ITEM()
RATIONAL_B_SPLINE_SURFACE(((1.,0.717491858961397,1.00013214700528),(1.,
0.717491366381689,1.00013214723569),(1.,0.717496644273678,1.00013214476688),
(1.,0.717495645633698,1.00013214523401),(1.,0.717492947926026,1.0001321464959),
(1.,0.717497270561146,1.00013214447393),(1.,0.717496233954528,1.00013214495881),
(1.,0.717487757692677,1.0001321489237),(1.,0.717497191556528,1.00013214451089),
(1.,0.717494070883108,1.00013214597062),(1.,0.717494808582735,1.00013214562555),
(1.,0.71749702304298,1.0001321445897),(1.,0.717489093728662,1.00013214829875),
(1.,0.717496657741948,1.00013214476058),(1.,0.717497221266918,1.00013214449699),
(1.,0.71749320996491,1.00013214637333),(1.,0.717492215950634,1.00013214683829),
(1.,0.71749542728491,1.00013214533615),(1.,0.717496219027939,1.0001321449658),
(1.,0.717496170669021,1.00013214498842),(1.,0.717492000648466,1.000132146939),
(1.,0.717497232101359,1.00013214449192),(1.,0.717496618895965,1.00013214477875),
(1.,0.717488914976109,1.00013214838237),(1.,0.717497072114508,1.00013214456675),
(1.,0.717494661677973,1.00013214569427),(1.,0.717494289673323,1.00013214586828),
(1.,0.717497161033782,1.00013214452516),(1.,0.717488242471211,1.00013214869694),
(1.,0.717496422146812,1.00013214487079),(1.,0.717497269224653,1.00013214447455),
(1.,0.7174925088005,1.00013214670131),(1.,0.7174959238285,1.00013214510388),
(1.,0.717496450378461,1.00013214485758),(1.,0.717489320105511,1.00013214819286),
(1.,0.717500022312063,1.00013214318676)))
REPRESENTATION_ITEM('')
SURFACE()
) ;
#47=(
BOUNDED_SURFACE()
B_SPLINE_SURFACE(1,2,((#9053,#9054,#9055,#9056,#9057,#9058,#9059,#9060,
#9061,#9062,#9063,#9064,#9065,#9066,#9067,#9068,#9069,#9070,#9071,#9072,
#9073,#9074,#9075),(#9076,#9077,#9078,#9079,#9080,#9081,#9082,#9083,#9084,
#9085,#9086,#9087,#9088,#9089,#9090,#9091,#9092,#9093,#9094,#9095,#9096,
#9097,#9098)),.UNSPECIFIED.,.F.,.F.,.F.)
B_SPLINE_SURFACE_WITH_KNOTS((2,2),(3,2,2,2,2,2,2,2,2,2,2,3),(0.,1.),(-1.0331090323905E-7,
0.0147058823529412,0.0294117647058824,0.0441176470588235,0.0588235294117647,
0.0735294117647059,0.0882352941176471,0.102941176470588,0.117647058823529,
0.132352941176471,0.147058823529412,0.159998951452637),.UNSPECIFIED.)
GEOMETRIC_REPRESENTATION_ITEM()
RATIONAL_B_SPLINE_SURFACE(((1.00000001499211,0.998932967306369,1.,0.998932974802372,
1.,0.998932974802372,1.,0.998932974802372,1.,0.998932974802372,1.,0.998932974802372,
1.,0.998932974802372,1.,0.998932974802372,1.,0.998932974802372,1.,0.998932974802372,
1.,0.999061093906287,0.999774528647208),(1.00000001499211,0.998932967306369,
1.,0.998932974802372,1.,0.998932974802372,1.,0.998932974802372,1.,0.998932974802372,
1.,0.998932974802372,1.,0.998932974802372,1.,0.998932974802372,1.,0.998932974802372,
1.,0.998932974802372,1.,0.999061093906287,0.999774528647208)))
REPRESENTATION_ITEM('')
SURFACE()
) ;
#48=(
BOUNDED_SURFACE()
B_SPLINE_SURFACE(1,2,((#9242,#9243,#9244,#9245,#9246,#9247,#9248,#9249,
#9250,#9251,#9252,#9253,#9254,#9255,#9256,#9257,#9258,#9259,#9260,#9261,
#9262,#9263,#9264),(#9265,#9266,#9267,#9268,#9269,#9270,#9271,#9272,#9273,
#9274,#9275,#9276,#9277,#9278,#9279,#9280,#9281,#9282,#9283,#9284,#9285,
#9286,#9287)),.UNSPECIFIED.,.F.,.F.,.F.)
B_SPLINE_SURFACE_WITH_KNOTS((2,2),(3,2,2,2,2,2,2,2,2,2,2,3),(-2.12079799133641E-9,
1.),(-4.92610666765903E-10,0.0147058823529412,0.0294117647058824,0.0441176470588235,
0.0588235294117647,0.0735294117647059,0.0882352941176471,0.102941176470588,
0.117647058823529,0.132352941176471,0.147058823529412,0.159999479208712),
 .UNSPECIFIED.)
GEOMETRIC_REPRESENTATION_ITEM()
RATIONAL_B_SPLINE_SURFACE(((1.00000000007149,0.99893297476663,1.,0.998932974802372,
1.,0.998932974802372,1.,0.998932974802372,1.,0.998932974802372,1.,0.998932974802372,
1.,0.998932974802372,1.,0.998932974802372,1.,0.998932974802372,1.,0.998932974802372,
1.,0.999061055613513,0.999774586844051),(1.00000000007149,0.99893297476663,
1.,0.998932974802372,1.,0.998932974802372,1.,0.998932974802372,1.,0.998932974802372,
1.,0.998932974802372,1.,0.998932974802372,1.,0.998932974802372,1.,0.998932974802372,
1.,0.998932974802372,1.,0.999061055613513,0.999774586844051)))
REPRESENTATION_ITEM('')
SURFACE()
) ;
#49=(
BOUNDED_SURFACE()
B_SPLINE_SURFACE(3,2,((#9454,#9455,#9456),(#9457,#9458,#9459),(#9460,#9461,
#9462),(#9463,#9464,#9465),(#9466,#9467,#9468),(#9469,#9470,#9471),(#9472,
#9473,#9474),(#9475,#9476,#9477),(#9478,#9479,#9480),(#9481,#9482,#9483),
(#9484,#9485,#9486),(#9487,#9488,#9489),(#9490,#9491,#9492),(#9493,#9494,
#9495),(#9496,#9497,#9498),(#9499,#9500,#9501),(#9502,#9503,#9504),(#9505,
#9506,#9507),(#9508,#9509,#9510),(#9511,#9512,#9513),(#9514,#9515,#9516),
(#9517,#9518,#9519),(#9520,#9521,#9522),(#9523,#9524,#9525),(#9526,#9527,
#9528),(#9529,#9530,#9531),(#9532,#9533,#9534),(#9535,#9536,#9537),(#9538,
#9539,#9540),(#9541,#9542,#9543),(#9544,#9545,#9546),(#9547,#9548,#9549)),
 .UNSPECIFIED.,.F.,.F.,.F.)
B_SPLINE_SURFACE_WITH_KNOTS((4,2,2,2,2,2,2,2,2,2,2,2,2,2,2,4),(3,3),(0.0363322941033848,
0.0552795959345893,0.0647532468501916,0.0742268977657939,0.0837005486813961,
0.0931741995969984,0.102647850512601,0.112121501428203,0.121595152343805,
0.131068803259407,0.14054245417501,0.150016105090612,0.159489756006214,
0.168963406921816,0.178437057837419,0.187910708753021),(0.,1.),
 .UNSPECIFIED.)
GEOMETRIC_REPRESENTATION_ITEM()
RATIONAL_B_SPLINE_SURFACE(((1.,0.713723577868383,1.),(1.,0.71372244524152,
1.),(1.,0.71372566235043,1.),(1.,0.713724573665381,1.),(1.,0.713722089517223,
1.),(1.,0.713725723121526,1.),(1.,0.713725237291428,1.),(1.,0.71371963332031,
1.),(1.,0.713725477049126,1.),(1.,0.713724228445444,1.),(1.,0.713722641365561,
1.),(1.,0.713725747741501,1.),(1.,0.713724999819642,1.),(1.,0.713718882738076,
1.),(1.,0.71372560714099,1.),(1.,0.713723850221543,1.),(1.,0.713723140170877,
1.),(1.,0.713725730025478,1.),(1.,0.713724718581176,1.),(1.,0.713718072451985,
1.),(1.,0.713725695588659,1.),(1.,0.713723420193482,1.),(1.,0.713723588743928,
1.),(1.,0.713725667827276,1.),(1.,0.713718399166187,1.),(1.,0.71372484390015,
1.),(1.,0.71372574176479,1.),(1.,0.713722939755319,1.),(1.,0.713724005027918,
1.),(1.,0.713725560117667,1.),(1.,0.713723126119328,1.),(1.,0.713721352883472,
1.)))
REPRESENTATION_ITEM('')
SURFACE()
) ;
#50=(
BOUNDED_SURFACE()
B_SPLINE_SURFACE(3,2,((#9550,#9551,#9552),(#9553,#9554,#9555),(#9556,#9557,
#9558),(#9559,#9560,#9561),(#9562,#9563,#9564),(#9565,#9566,#9567),(#9568,
#9569,#9570),(#9571,#9572,#9573),(#9574,#9575,#9576),(#9577,#9578,#9579),
(#9580,#9581,#9582),(#9583,#9584,#9585),(#9586,#9587,#9588),(#9589,#9590,
#9591),(#9592,#9593,#9594),(#9595,#9596,#9597),(#9598,#9599,#9600),(#9601,
#9602,#9603),(#9604,#9605,#9606),(#9607,#9608,#9609),(#9610,#9611,#9612),
(#9613,#9614,#9615),(#9616,#9617,#9618),(#9619,#9620,#9621),(#9622,#9623,
#9624),(#9625,#9626,#9627),(#9628,#9629,#9630),(#9631,#9632,#9633),(#9634,
#9635,#9636),(#9637,#9638,#9639),(#9640,#9641,#9642),(#9643,#9644,#9645),
(#9646,#9647,#9648),(#9649,#9650,#9651),(#9652,#9653,#9654),(#9655,#9656,
#9657)),.UNSPECIFIED.,.F.,.F.,.F.)
B_SPLINE_SURFACE_WITH_KNOTS((4,2,2,2,2,2,2,2,2,2,2,2,2,2,2,2,2,4),(3,3),
(0.110192674671804,0.119968567976379,0.129744461280954,0.139520354585529,
0.149296247890104,0.159072141194679,0.168848034499254,0.178623927803829,
0.183511874456117,0.188399821108404,0.198175714412979,0.207951607717554,
0.217727501022129,0.227503394326705,0.23727928763128,0.247055180935855,
0.25683107424043,0.266606967545005),(0.,1.),.UNSPECIFIED.)
GEOMETRIC_REPRESENTATION_ITEM()
RATIONAL_B_SPLINE_SURFACE(((1.,0.717557917014258,1.),(1.,0.717557424560011,
1.),(1.,0.717562701193914,1.),(1.,0.717561702814847,1.),(1.,0.71755900564737,
1.),(1.,0.717563327425588,1.),(1.,0.717562291025758,1.),(1.,0.717553816663223,
1.),(1.,0.717563248329896,1.),(1.,0.717560128451358,1.),(1.,0.717560865886123,
1.),(1.,0.717563079948143,1.),(1.,0.717555152391406,1.),(1.,0.717562714709462,
1.),(1.,0.717563278031631,1.),(1.,0.717559267718992,1.),(1.,0.71755827387268,
1.),(1.,0.717561484550715,1.),(1.,0.717562276065883,1.),(1.,0.717562227704526,
1.),(1.,0.71755805869716,1.),(1.,0.71756328886893,1.),(1.,0.717562675764556,
1.),(1.,0.717554973788595,1.),(1.,0.717563128952974,1.),(1.,0.717560719070892,
1.),(1.,0.717560347081223,1.),(1.,0.717563217923494,1.),(1.,0.71755430141606,
1.),(1.,0.717562479086372,1.),(1.,0.717563326002921,1.),(1.,0.717558566710936,
1.),(1.,0.71756198091345,1.),(1.,0.717562507375146,1.),(1.,0.717555378738943,
1.),(1.,0.717566078456158,1.)))
REPRESENTATION_ITEM('')
SURFACE()
) ;
#51=B_SPLINE_CURVE_WITH_KNOTS('',3,(#5793,#5794,#5795,#5796),
 .UNSPECIFIED.,.F.,.F.,(4,4),(0.149240959230156,0.155663525084362),
 .UNSPECIFIED.) ;
#52=B_SPLINE_CURVE_WITH_KNOTS('',3,(#5805,#5806,#5807,#5808,#5809,#5810,
#5811,#5812,#5813,#5814,#5815,#5816,#5817,#5818,#5819,#5820,#5821,#5822,
#5823,#5824,#5825,#5826,#5827,#5828,#5829,#5830,#5831,#5832,#5833,#5834,
#5835,#5836,#5837,#5838,#5839,#5840,#5841,#5842,#5843,#5844,#5845,#5846,
#5847,#5848,#5849,#5850,#5851,#5852,#5853,#5854,#5855,#5856,#5857,#5858,
#5859,#5860),.UNSPECIFIED.,.F.,.F.,(4,2,2,2,2,2,2,2,2,2,2,2,2,2,2,2,2,2,
2,2,2,2,2,2,2,2,2,4),(0.,0.00731512878245589,0.00902075833180565,0.0167240727068727,
0.0180415166636113,0.0261381508744796,0.027062274995417,0.0355562466737043,
0.0360830333272226,0.0449741716251418,0.0451037916590283,0.0541245499908339,
0.0543919669055456,0.0631453083226396,0.0638099851771147,0.0721660666544452,
0.0732283939342589,0.0826464947664068,0.0902075833180562,0.0920641197300344,
0.0992283416498616,0.101482130305131,0.108249099981667,0.110900185947423,
0.120317603377353,0.126290616645278,0.129734235290266,0.14433212758977),
 .UNSPECIFIED.) ;
#53=B_SPLINE_CURVE_WITH_KNOTS('',3,(#5862,#5863,#5864,#5865),
 .UNSPECIFIED.,.F.,.F.,(4,4),(-0.00866851853360736,0.),.UNSPECIFIED.) ;
#54=B_SPLINE_CURVE_WITH_KNOTS('',3,(#5868,#5869,#5870,#5871,#5872,#5873,
#5874,#5875,#5876,#5877,#5878,#5879,#5880,#5881,#5882,#5883,#5884,#5885,
#5886,#5887,#5888,#5889,#5890,#5891,#5892,#5893,#5894,#5895,#5896,#5897,
#5898,#5899,#5900,#5901,#5902,#5903,#5904,#5905,#5906,#5907,#5908,#5909,
#5910,#5911,#5912,#5913,#5914,#5915,#5916,#5917,#5918,#5919,#5920,#5921,
#5922,#5923,#5924,#5925,#5926,#5927,#5928,#5929),.UNSPECIFIED.,.F.,.F.,
(4,2,2,2,2,2,2,2,2,2,2,2,2,2,2,2,2,2,2,2,2,2,2,2,2,2,2,2,2,2,4),(3.94956318998463E-8,
0.00891142814756958,0.00932755995188492,0.0186551199037698,0.0187613828160708,
0.0286110142999948,0.0373102398075393,0.0384607884393804,0.046637799759424,
0.0483108212289063,0.0559653597113087,0.0581608694451579,0.0652929196631934,
0.0680105025743505,0.0746204796150781,0.0778602470751006,0.0827853130796942,
0.0839480395669628,0.0877102729721427,0.0932755995188474,0.0975581095945039,
0.102603159470732,0.107402909010666,0.111930719422617,0.117245126652995,
0.121258279374501,0.127085194433039,0.130585839326386,0.136923514137084,
0.146760505439294,0.149240959230156),.UNSPECIFIED.) ;
#55=B_SPLINE_CURVE_WITH_KNOTS('',3,(#5932,#5933,#5934,#5935,#5936,#5937,
#5938,#5939,#5940,#5941,#5942,#5943,#5944,#5945,#5946,#5947,#5948,#5949,
#5950,#5951),.UNSPECIFIED.,.F.,.F.,(4,2,2,2,2,2,2,2,2,4),(0.0897547274400454,
0.0920640826369811,0.101482011794833,0.103399078907256,0.110221254640862,
0.110900374996111,0.117043430374467,0.12031784279818,0.12973472062429,0.144332127589771),
 .UNSPECIFIED.) ;
#56=B_SPLINE_CURVE_WITH_KNOTS('',3,(#5953,#5954,#5955,#5956),
 .UNSPECIFIED.,.F.,.F.,(4,4),(-0.0147595409796903,0.),.UNSPECIFIED.) ;
#57=B_SPLINE_CURVE_WITH_KNOTS('',3,(#5960,#5961,#5962,#5963,#5964,#5965,
#5966,#5967,#5968,#5969,#5970,#5971,#5972,#5973,#5974,#5975,#5976,#5977),
 .UNSPECIFIED.,.F.,.F.,(4,2,2,2,2,2,2,2,4),(3.23478334301053E-8,0.00950796128231213,
0.0136581275144307,0.0258902720983011,0.0273162550288615,0.0409743825432922,
0.0474513189825906,0.0478034463005076,0.0546325100577231),.UNSPECIFIED.) ;
#58=B_SPLINE_CURVE_WITH_KNOTS('',3,(#5979,#5980,#5981,#5982,#5983,#5984,
#5985,#5986,#5987,#5988,#5989,#5990,#5991,#5992,#5993,#5994,#5995,#5996,
#5997,#5998,#5999,#6000,#6001,#6002,#6003,#6004,#6005,#6006,#6007,#6008,
#6009,#6010,#6011,#6012,#6013,#6014,#6015,#6016,#6017,#6018,#6019,#6020,
#6021,#6022,#6023,#6024,#6025,#6026,#6027,#6028,#6029,#6030,#6031,#6032,
#6033,#6034,#6035,#6036,#6037,#6038,#6039),.UNSPECIFIED.,.F.,.F.,(4,3,3,
3,3,3,3,3,3,3,3,3,3,3,3,3,3,3,3,3,4),(0.0546325100577231,0.058160873912377,
0.067357759257812,0.0680104909370463,0.0778602344007145,0.0798902638143831,
0.0827851932736896,0.086204702253548,0.0877102855556224,0.0925191406927129,
0.0975581115684209,0.105148017571043,0.107402908109119,0.116343229848907,
0.117245131820784,0.127085188202925,0.130405771327702,0.136923515438958,
0.143034648206032,0.146760502503953,0.155663525084362),.UNSPECIFIED.) ;
#59=B_SPLINE_CURVE_WITH_KNOTS('',3,(#6042,#6043,#6044,#6045,#6046,#6047,
#6048,#6049,#6050,#6051,#6052,#6053,#6054,#6055,#6056,#6057,#6058,#6059,
#6060,#6061,#6062,#6063,#6064,#6065,#6066,#6067,#6068,#6069,#6070,#6071,
#6072,#6073,#6074,#6075,#6076,#6077,#6078),.UNSPECIFIED.,.F.,.F.,(4,2,2,
2,2,2,2,2,2,3,2,2,2,2,2,2,2,4),(0.,0.00731512646279782,0.0112193409300058,
0.016724079282874,0.0224386818600116,0.0261380306119276,0.0336580227900174,
0.0355562890153248,0.0448773637200232,0.0449741716018943,0.0543919626298755,
0.0560967046500289,0.0638102284561295,0.0673160455800344,0.0732282109179109,
0.0785353865100399,0.0826463437232967,0.0897547274400454),.UNSPECIFIED.) ;
#60=B_SPLINE_CURVE_WITH_KNOTS('',3,(#6081,#6082,#6083,#6084,#6085,#6086,
#6087,#6088,#6089,#6090,#6091,#6092,#6093,#6094,#6095,#6096,#6097,#6098,
#6099,#6100,#6101,#6102,#6103,#6104,#6105,#6106,#6107,#6108,#6109,#6110,
#6111,#6112,#6113,#6114,#6115,#6116,#6117,#6118,#6119,#6120,#6121,#6122,
#6123,#6124,#6125,#6126,#6127,#6128,#6129,#6130,#6131,#6132,#6133,#6134,
#6135,#6136),.UNSPECIFIED.,.F.,.F.,(4,2,2,2,2,2,2,2,2,2,2,2,2,2,2,2,2,2,
2,2,2,2,2,2,2,2,2,4),(0.,0.00731512878238814,0.00902075833180564,0.0167240727068785,
0.0180415166636113,0.0261381508744852,0.0270622749954169,0.0355562466737161,
0.0360830333272226,0.0449741716251424,0.0451037916590282,0.0541245499908339,
0.0543919669055449,0.0631453083226395,0.0638099851771106,0.0721660666544451,
0.0732283939342739,0.0826464947663908,0.0902075833180561,0.0920641197300239,
0.0992283416498616,0.101482130305075,0.108249099981667,0.110900185947284,
0.120317603377234,0.126290616645278,0.129734235290253,0.144332127589754),
 .UNSPECIFIED.) ;
#61=B_SPLINE_CURVE_WITH_KNOTS('',3,(#6138,#6139,#6140,#6141),
 .UNSPECIFIED.,.F.,.F.,(4,4),(-0.0147606579860161,0.),.UNSPECIFIED.) ;
#62=B_SPLINE_CURVE_WITH_KNOTS('',3,(#6145,#6146,#6147,#6148,#6149,#6150,
#6151,#6152,#6153,#6154,#6155,#6156,#6157,#6158,#6159,#6160,#6161,#6162,
#6163,#6164,#6165,#6166,#6167,#6168,#6169,#6170,#6171,#6172,#6173,#6174,
#6175,#6176,#6177,#6178,#6179,#6180,#6181,#6182,#6183,#6184,#6185,#6186,
#6187,#6188,#6189,#6190,#6191,#6192,#6193,#6194,#6195,#6196,#6197,#6198,
#6199,#6200,#6201,#6202,#6203,#6204,#6205,#6206,#6207,#6208),
 .UNSPECIFIED.,.F.,.F.,(4,2,2,2,2,2,2,2,2,2,2,2,2,3,2,3,2,2,2,2,2,2,2,2,
2,2,2,2,2,2,4),(3.94954787930727E-8,0.00891142512110372,0.00972897031777275,
0.0187613829416187,0.0194579406355455,0.028610894536375,0.0384607392810885,
0.0389158812710911,0.0483109273475211,0.0486448515888637,0.0581608647626506,
0.0583738219066363,0.0680105056195261,0.068102792224409,0.0778317625421816,
0.0778602325221652,0.0827853055179139,0.0875607328599542,0.0877103163614879,
0.0972897031777268,0.0975581136408448,0.107018673495499,0.107402909551261,
0.116747643813272,0.117245122911299,0.127085197251929,0.136205584448817,
0.136923529027027,0.14593455476659,0.146760502952475,0.155663525084362),
 .UNSPECIFIED.) ;
#63=B_SPLINE_CURVE_WITH_KNOTS('',3,(#6212,#6213,#6214,#6215,#6216,#6217,
#6218,#6219,#6220,#6221,#6222,#6223,#6224,#6225,#6226,#6227,#6228,#6229,
#6230,#6231,#6232,#6233,#6234,#6235,#6236,#6237,#6238,#6239,#6240,#6241,
#6242,#6243,#6244,#6245,#6246,#6247,#6248,#6249,#6250,#6251,#6252,#6253,
#6254,#6255,#6256,#6257,#6258,#6259,#6260,#6261,#6262,#6263,#6264,#6265,
#6266,#6267,#6268),.UNSPECIFIED.,.F.,.F.,(4,2,2,2,2,2,2,2,2,2,3,2,2,2,2,
2,2,2,2,2,2,2,2,2,2,2,2,4),(0.,0.00731512878242812,0.00902075833180566,
0.016724072706909,0.0180415166636113,0.0261381508744844,0.027062274995417,
0.0355562466737159,0.0360830333272226,0.0449741716251424,0.0451037916590283,
0.054124549990834,0.0543919669055458,0.0631453083226396,0.0638099851771047,
0.0721660666544453,0.0732283939342734,0.0826464947662712,0.0902075833180563,
0.0920641197300701,0.0992283416498616,0.101482130305197,0.108249099981667,
0.110900185947437,0.120317603377343,0.126290616645278,0.129734235290238,
0.144332127589761),.UNSPECIFIED.) ;
#64=B_SPLINE_CURVE_WITH_KNOTS('',3,(#6270,#6271,#6272,#6273),
 .UNSPECIFIED.,.F.,.F.,(4,4),(-0.0147606630153147,0.),.UNSPECIFIED.) ;
#65=B_SPLINE_CURVE_WITH_KNOTS('',3,(#6277,#6278,#6279,#6280,#6281,#6282,
#6283,#6284,#6285,#6286,#6287,#6288,#6289,#6290,#6291,#6292,#6293,#6294,
#6295,#6296,#6297,#6298,#6299,#6300,#6301,#6302,#6303,#6304,#6305,#6306,
#6307,#6308,#6309,#6310,#6311,#6312,#6313,#6314,#6315,#6316,#6317,#6318,
#6319,#6320,#6321,#6322,#6323,#6324,#6325,#6326,#6327,#6328,#6329,#6330,
#6331,#6332,#6333,#6334,#6335,#6336,#6337,#6338,#6339),.UNSPECIFIED.,.F.,
 .F.,(4,2,2,2,2,2,2,2,2,2,2,2,2,2,2,3,2,2,2,2,2,2,2,2,2,2,2,2,2,2,4),(3.9495430696627E-8,
0.00891142512111904,0.00972897031777276,0.0187613829416347,0.0194579406355455,
0.028610894536505,0.0384607392810928,0.038915881271091,0.0483109273475251,
0.0486448515888636,0.0581608647626519,0.0583738219066362,0.0680105056195256,
0.0681027922244088,0.0778317625421815,0.0778602325221654,0.0827853055178527,
0.0875607328599541,0.0877103163614874,0.0972897031777267,0.0975581136408476,
0.107018673495499,0.107402909551269,0.116747643813272,0.117245122911301,
0.127085197251926,0.136205584448817,0.136923529027022,0.14593455476659,
0.146760502952473,0.155663525084362),.UNSPECIFIED.) ;
#66=B_SPLINE_CURVE_WITH_KNOTS('',3,(#6343,#6344,#6345,#6346,#6347,#6348,
#6349,#6350,#6351,#6352,#6353,#6354,#6355,#6356,#6357,#6358,#6359,#6360,
#6361,#6362,#6363,#6364,#6365,#6366,#6367,#6368,#6369,#6370,#6371,#6372,
#6373,#6374,#6375,#6376,#6377,#6378,#6379,#6380,#6381,#6382,#6383,#6384,
#6385,#6386,#6387,#6388,#6389,#6390,#6391,#6392,#6393,#6394,#6395,#6396,
#6397,#6398),.UNSPECIFIED.,.F.,.F.,(4,2,2,2,2,2,2,2,2,2,2,2,2,2,2,2,2,2,
2,2,2,2,2,2,2,2,2,4),(0.,0.00731512878240043,0.00902075833180559,0.0167240727069339,
0.0180415166636112,0.0261381508744801,0.0270622749954168,0.0355562466737007,
0.0360830333272225,0.0449741716251419,0.0451037916590281,0.0541245499908337,
0.0543919669055447,0.0631453083226394,0.0638099851770966,0.072166066654445,
0.0732283939342627,0.0826464947664404,0.090207583318056,0.0920641197300776,
0.0992283416498613,0.101482130305149,0.108249099981667,0.110900185947403,
0.120317603377446,0.126290616645278,0.12973423529026,0.144332127589769),
 .UNSPECIFIED.) ;
#67=B_SPLINE_CURVE_WITH_KNOTS('',3,(#6400,#6401,#6402,#6403),
 .UNSPECIFIED.,.F.,.F.,(4,4),(-0.00866852031690021,0.),.UNSPECIFIED.) ;
#68=B_SPLINE_CURVE_WITH_KNOTS('',3,(#6407,#6408,#6409,#6410,#6411,#6412,
#6413,#6414,#6415,#6416,#6417,#6418,#6419,#6420,#6421,#6422,#6423,#6424,
#6425,#6426,#6427,#6428,#6429,#6430,#6431,#6432,#6433,#6434,#6435,#6436,
#6437,#6438,#6439,#6440,#6441,#6442,#6443,#6444,#6445,#6446,#6447,#6448,
#6449,#6450,#6451,#6452,#6453,#6454,#6455,#6456,#6457,#6458,#6459,#6460,
#6461,#6462,#6463,#6464,#6465,#6466,#6467,#6468,#6469),.UNSPECIFIED.,.F.,
 .F.,(4,2,2,2,2,2,2,2,2,2,2,2,2,2,2,3,2,2,2,2,2,2,2,2,2,2,2,2,2,2,4),(3.94954778143609E-8,
0.00891142512111536,0.00972897031777272,0.0187613829416454,0.0194579406355454,
0.0286108945365536,0.038460739281093,0.0389158812710909,0.0483109273475189,
0.0486448515888637,0.058160864762651,0.0583738219066364,0.068010505619526,
0.0681027922244092,0.077831762542182,0.0778602325221656,0.0827853055180071,
0.0875607328599548,0.0877103163614895,0.0972897031777276,0.0975581136408469,
0.1070186734955,0.107402909551265,0.116747643813273,0.1172451229113,0.127085197251908,
0.136205584448817,0.136923529027016,0.14593455476659,0.146760502952471,
0.155663525084362),.UNSPECIFIED.) ;
#69=B_SPLINE_CURVE_WITH_KNOTS('',3,(#6475,#6476,#6477,#6478,#6479,#6480,
#6481,#6482,#6483,#6484,#6485,#6486),.UNSPECIFIED.,.F.,.F.,(4,2,2,2,2,4),
(-0.337170890175032,-0.295474578031491,-0.250449400518782,-0.168586531681465,
-0.0800191535060179,0.),.UNSPECIFIED.) ;
#70=B_SPLINE_CURVE_WITH_KNOTS('',3,(#6488,#6489,#6490,#6491,#6492,#6493,
#6494,#6495,#6496,#6497,#6498,#6499),.UNSPECIFIED.,.F.,.F.,(4,2,2,2,2,4),
(-0.333222107964713,-0.254909679222191,-0.166608972895279,-0.0849984861950195,
-0.0408878594142492,0.),.UNSPECIFIED.) ;
#71=B_SPLINE_CURVE_WITH_KNOTS('',3,(#6551,#6552,#6553,#6554,#6555,#6556),
 .UNSPECIFIED.,.F.,.F.,(4,2,4),(9.99999864681522E-7,7.73756153016491,14.6500515074066),
 .UNSPECIFIED.) ;
#72=B_SPLINE_CURVE_WITH_KNOTS('',3,(#6557,#6558,#6559,#6560,#6561,#6562,
#6563,#6564,#6565,#6566,#6567,#6568,#6569,#6570,#6571,#6572,#6573,#6574,
#6575,#6576,#6577,#6578,#6579,#6580,#6581,#6582,#6583,#6584,#6585,#6586,
#6587,#6588,#6589,#6590,#6591,#6592,#6593,#6594,#6595,#6596,#6597,#6598,
#6599,#6600,#6601,#6602,#6603,#6604,#6605,#6606,#6607,#6608,#6609,#6610,
#6611,#6612,#6613,#6614,#6615,#6616,#6617,#6618,#6619,#6620,#6621,#6622,
#6623,#6624,#6625,#6626,#6627,#6628,#6629,#6630,#6631,#6632,#6633,#6634,
#6635,#6636,#6637,#6638,#6639,#6640,#6641,#6642,#6643,#6644),
 .UNSPECIFIED.,.F.,.F.,(4,3,3,3,3,3,3,3,3,3,3,3,3,3,3,3,3,3,3,3,3,3,3,3,
3,3,3,3,3,4),(0.,0.00937963669820284,0.0180867052587593,0.0187592733964057,
0.0275801848733995,0.0281389100946085,0.0370735108965404,0.0375185467928114,
0.0465678590763149,0.0468981834910142,0.0560614220554019,0.056277820189217,
0.0655556527434089,0.0750370935856226,0.0750489969011788,0.0844167302838255,
0.0845426524492584,0.0937963669820284,0.0940356196999413,0.103176003680231,
0.103530146128526,0.112555640378434,0.113023868907298,0.121935277076637,
0.122516583962713,0.13131491377484,0.132007368634961,0.140694550473043,
0.141493081370673,0.150074187171246),.UNSPECIFIED.) ;
#73=B_SPLINE_CURVE_WITH_KNOTS('',3,(#6646,#6647,#6648,#6649,#6650,#6651,
#6652,#6653,#6654,#6655,#6656,#6657),.UNSPECIFIED.,.F.,.F.,(4,2,2,2,2,4),
(1.000000006113E-6,1.57108044003981,3.17385828869477,5.99475389679247,9.05882226516005,
11.9895252463837),.UNSPECIFIED.) ;
#74=B_SPLINE_CURVE_WITH_KNOTS('',3,(#6678,#6679,#6680,#6681,#6682,#6683,
#6684,#6685,#6686,#6687,#6688,#6689,#6690,#6691),.UNSPECIFIED.,.F.,.F.,
(4,2,2,2,2,2,4),(3.16384028085258E-15,1.73074433286408,3.58539416576252,
6.63006684161914,9.43481733805421,11.4958871896749,13.2600099107559),
 .UNSPECIFIED.) ;
#75=B_SPLINE_CURVE_WITH_KNOTS('',3,(#6739,#6740,#6741,#6742,#6743,#6744,
#6745,#6746,#6747,#6748,#6749,#6750,#6751,#6752,#6753,#6754,#6755,#6756,
#6757,#6758,#6759,#6760,#6761,#6762,#6763,#6764,#6765,#6766,#6767,#6768,
#6769,#6770,#6771,#6772,#6773,#6774,#6775,#6776,#6777,#6778,#6779,#6780,
#6781,#6782,#6783,#6784,#6785,#6786,#6787,#6788,#6789,#6790,#6791,#6792,
#6793,#6794,#6795,#6796,#6797,#6798,#6799,#6800,#6801,#6802,#6803,#6804,
#6805,#6806,#6807,#6808,#6809,#6810,#6811,#6812,#6813,#6814,#6815,#6816,
#6817,#6818),.UNSPECIFIED.,.F.,.F.,(4,2,2,2,2,2,2,2,2,2,2,2,2,2,2,2,2,2,
2,2,2,2,2,2,2,2,2,2,2,2,2,2,2,2,2,2,2,2,2,4),(-5.99999999998624E-8,0.000590526800461016,
0.00118111360092203,0.00236228720184421,0.00472463440368856,0.00769960210153364,
0.00944932880737708,0.0175309308941166,0.0188987176147543,0.0273655127101969,
0.0372020310641398,0.0377974952295087,0.0470416860700581,0.0472468840368859,
0.056696272844263,0.0568833874626172,0.0661456616516403,0.0667287422857246,
0.0716522046058592,0.0755950504590174,0.0765761128198491,0.086423531293351,
0.0944938280737717,0.0962698644460277,0.103943216881149,0.106117401685429,
0.113392605688526,0.115965067364374,0.122841994495903,0.125814419594229,
0.13229138330328,0.135667192159133,0.141740772110657,0.145521654063409,
0.146465466514346,0.14882781371619,0.150008786432466,0.150599272790603,
0.150760142698118,0.151189743027088),.UNSPECIFIED.) ;
#76=B_SPLINE_CURVE_WITH_KNOTS('',3,(#6820,#6821,#6822,#6823,#6824,#6825),
 .UNSPECIFIED.,.F.,.F.,(4,2,4),(3.60319835854062E-5,9.64490115774811,19.2897662777575),
 .UNSPECIFIED.) ;
#77=B_SPLINE_CURVE_WITH_KNOTS('',3,(#6827,#6828,#6829,#6830,#6831,#6832,
#6833,#6834,#6835,#6836,#6837,#6838,#6839,#6840),.UNSPECIFIED.,.F.,.F.,
(4,2,2,2,2,2,4),(1.00000002995617E-6,1.7692530094857,3.83875002010364,6.637598522414,
9.67546927736373,11.5382441958309,13.275259829094),.UNSPECIFIED.) ;
#78=B_SPLINE_CURVE_WITH_KNOTS('',3,(#6857,#6858,#6859,#6860,#6861,#6862,
#6863,#6864,#6865,#6866,#6867,#6868,#6869,#6870),.UNSPECIFIED.,.F.,.F.,
(4,2,2,2,2,2,4),(9.99999993593914E-7,1.73146252564964,3.58437512441185,
6.6300673358595,9.43722227701482,11.4955951658395,13.2600876660263),
 .UNSPECIFIED.) ;
#79=B_SPLINE_CURVE_WITH_KNOTS('',3,(#6878,#6879,#6880,#6881,#6882,#6883,
#6884,#6885,#6886,#6887,#6888,#6889),.UNSPECIFIED.,.F.,.F.,(4,2,2,2,2,4),
(1.45423920475118E-6,0.136695796634482,0.26996812895029,0.393732693444733,
0.460063012688564,0.516324865534141),.UNSPECIFIED.) ;
#80=B_SPLINE_CURVE_WITH_KNOTS('',3,(#6890,#6891,#6892,#6893,#6894,#6895,
#6896,#6897,#6898,#6899,#6900,#6901,#6902,#6903),.UNSPECIFIED.,.F.,.F.,
(4,2,2,2,2,2,4),(0.,0.0210914408170582,0.0435982414579784,0.0952050288075531,
0.187105593312812,0.287813738176817,0.391818327243934),.UNSPECIFIED.) ;
#81=B_SPLINE_CURVE_WITH_KNOTS('',3,(#7113,#7114,#7115,#7116,#7117,#7118,
#7119,#7120,#7121,#7122,#7123,#7124),.UNSPECIFIED.,.F.,.F.,(4,2,2,2,2,4),
(-0.337170890197259,-0.295474578044017,-0.250449400521991,-0.168586531692847,
-0.0800191535398783,0.),.UNSPECIFIED.) ;
#82=B_SPLINE_CURVE_WITH_KNOTS('',3,(#7126,#7127,#7128,#7129,#7130,#7131,
#7132,#7133,#7134,#7135,#7136,#7137),.UNSPECIFIED.,.F.,.F.,(4,2,2,2,2,4),
(-0.333222107966658,-0.254909679269947,-0.166608972896623,-0.084998486132098,
-0.0408878593827511,0.),.UNSPECIFIED.) ;
#83=B_SPLINE_CURVE_WITH_KNOTS('',3,(#7189,#7190,#7191,#7192,#7193,#7194),
 .UNSPECIFIED.,.F.,.F.,(4,2,4),(9.99999998905569E-7,7.73756066856093,14.6500505460067),
 .UNSPECIFIED.) ;
#84=B_SPLINE_CURVE_WITH_KNOTS('',3,(#7195,#7196,#7197,#7198,#7199,#7200,
#7201,#7202,#7203,#7204,#7205,#7206,#7207,#7208,#7209,#7210,#7211,#7212,
#7213,#7214,#7215,#7216,#7217,#7218,#7219,#7220,#7221,#7222,#7223,#7224,
#7225,#7226,#7227,#7228,#7229,#7230,#7231,#7232,#7233,#7234,#7235,#7236,
#7237,#7238,#7239,#7240,#7241,#7242,#7243,#7244,#7245,#7246,#7247,#7248,
#7249,#7250,#7251,#7252,#7253,#7254,#7255,#7256,#7257,#7258,#7259,#7260,
#7261,#7262,#7263,#7264,#7265,#7266,#7267,#7268,#7269,#7270,#7271,#7272,
#7273,#7274,#7275,#7276,#7277,#7278,#7279,#7280,#7281,#7282),
 .UNSPECIFIED.,.F.,.F.,(4,3,3,3,3,3,3,3,3,3,3,3,3,3,3,3,3,3,3,3,3,3,3,3,
3,3,3,3,3,4),(0.,0.00937963669820301,0.0180867052587536,0.018759273396406,
0.0275801848734017,0.028138910094609,0.0370735108965484,0.037518546792812,
0.0465678590763189,0.046898183491015,0.0560614220554027,0.0562778201892181,
0.0655556527434121,0.0750370935856239,0.0750489969011802,0.0844167302838267,
0.0845426524492591,0.0937963669820294,0.0940356196999414,0.103176003680232,
0.103530146128525,0.112555640378435,0.113023868907291,0.121935277076638,
0.122516583962711,0.13131491377484,0.132007368634953,0.140694550473043,
0.141493081370687,0.150074187171246),.UNSPECIFIED.) ;
#85=B_SPLINE_CURVE_WITH_KNOTS('',3,(#7284,#7285,#7286,#7287,#7288,#7289,
#7290,#7291,#7292,#7293,#7294,#7295),.UNSPECIFIED.,.F.,.F.,(4,2,2,2,2,4),
(1.00000001060884E-6,1.5710804400398,3.17385828869448,5.99475389679188,
9.05882226515939,11.9895252463828),.UNSPECIFIED.) ;
#86=B_SPLINE_CURVE_WITH_KNOTS('',3,(#7316,#7317,#7318,#7319,#7320,#7321,
#7322,#7323,#7324,#7325,#7326,#7327,#7328,#7329),.UNSPECIFIED.,.F.,.F.,
(4,2,2,2,2,2,4),(4.9472447807214E-14,1.73074409285085,3.58539363528042,
6.630066337806,9.43481685331838,11.4958869837882,13.2600099122335),
 .UNSPECIFIED.) ;
#87=B_SPLINE_CURVE_WITH_KNOTS('',3,(#7377,#7378,#7379,#7380,#7381,#7382,
#7383,#7384,#7385,#7386,#7387,#7388,#7389,#7390,#7391,#7392,#7393,#7394,
#7395,#7396,#7397,#7398,#7399,#7400,#7401,#7402,#7403,#7404,#7405,#7406,
#7407,#7408,#7409,#7410,#7411,#7412,#7413,#7414,#7415,#7416,#7417,#7418,
#7419,#7420,#7421,#7422,#7423,#7424,#7425,#7426,#7427,#7428,#7429,#7430,
#7431,#7432,#7433,#7434,#7435,#7436,#7437,#7438,#7439,#7440,#7441,#7442,
#7443,#7444,#7445,#7446,#7447,#7448,#7449,#7450,#7451,#7452,#7453,#7454,
#7455,#7456),.UNSPECIFIED.,.F.,.F.,(4,2,2,2,2,2,2,2,2,2,2,2,2,2,2,2,2,2,
2,2,2,2,2,2,2,2,2,2,2,2,2,2,2,2,2,2,2,2,2,4),(-5.99999999998624E-8,0.000590526800461144,
0.00118111360092229,0.00236228720184452,0.00472463440368883,0.0076996021015449,
0.00944932880737732,0.0175309308941572,0.0188987176147545,0.0273655127104135,
0.0372020310641432,0.0377974952295087,0.0470416860700603,0.0472468840368859,
0.056696272844263,0.0568833874626158,0.0661456616516401,0.0667287422857208,
0.071652204605778,0.0755950504590172,0.0765761128198549,0.0864235312935481,
0.0944938280737713,0.0962698644460535,0.103943216881148,0.106117401685444,
0.113392605688525,0.115965067364384,0.122841994495902,0.125814419594311,
0.132291383303279,0.135667192159198,0.141740772110656,0.145521654063392,
0.146465466514345,0.148827813716189,0.150008786432462,0.150599272790598,
0.150760142698139,0.151189743027081),.UNSPECIFIED.) ;
#88=B_SPLINE_CURVE_WITH_KNOTS('',3,(#7458,#7459,#7460,#7461,#7462,#7463),
 .UNSPECIFIED.,.F.,.F.,(4,2,4),(3.60319838392225E-5,9.64490115776298,19.2897662777871),
 .UNSPECIFIED.) ;
#89=B_SPLINE_CURVE_WITH_KNOTS('',3,(#7465,#7466,#7467,#7468,#7469,#7470,
#7471,#7472,#7473,#7474,#7475,#7476,#7477,#7478),.UNSPECIFIED.,.F.,.F.,
(4,2,2,2,2,2,4),(9.99999994089207E-7,1.76925387621149,3.83875073093921,
6.63759902241896,9.67546954853305,11.5382443266811,13.2752598290988),
 .UNSPECIFIED.) ;
#90=B_SPLINE_CURVE_WITH_KNOTS('',3,(#7495,#7496,#7497,#7498,#7499,#7500,
#7501,#7502,#7503,#7504,#7505,#7506,#7507,#7508),.UNSPECIFIED.,.F.,.F.,
(4,2,2,2,2,2,4),(1.00000001476021E-6,1.73146252564982,3.58437512441194,
6.63006733585989,9.43722227701539,11.4955951658406,13.260087666028),
 .UNSPECIFIED.) ;
#91=B_SPLINE_CURVE_WITH_KNOTS('',3,(#7516,#7517,#7518,#7519,#7520,#7521,
#7522,#7523,#7524,#7525,#7526,#7527),.UNSPECIFIED.,.F.,.F.,(4,2,2,2,2,4),
(9.99999888340319E-7,0.136552307695273,0.269611694582245,0.393232608950036,
0.459467944573314,0.515661056622118),.UNSPECIFIED.) ;
#92=B_SPLINE_CURVE_WITH_KNOTS('',3,(#7528,#7529,#7530,#7531,#7532,#7533,
#7534,#7535,#7536,#7537,#7538,#7539,#7540,#7541),.UNSPECIFIED.,.F.,.F.,
(4,2,2,2,2,2,4),(0.,0.0210914408174009,0.0435982414581033,0.095205028809359,
0.187105593316175,0.287813738154874,0.391818327188839),.UNSPECIFIED.) ;
#93=B_SPLINE_CURVE_WITH_KNOTS('',3,(#7751,#7752,#7753,#7754,#7755,#7756,
#7757,#7758,#7759,#7760,#7761,#7762),.UNSPECIFIED.,.F.,.F.,(4,2,2,2,2,4),
(-0.337170890186573,-0.295474578033596,-0.25044940051207,-0.168586531687245,
-0.08001915354066,0.),.UNSPECIFIED.) ;
#94=B_SPLINE_CURVE_WITH_KNOTS('',3,(#7764,#7765,#7766,#7767,#7768,#7769,
#7770,#7771,#7772,#7773,#7774,#7775),.UNSPECIFIED.,.F.,.F.,(4,2,2,2,2,4),
(-0.333222107963772,-0.254909679273463,-0.166608972895298,-0.0849984861465236,
-0.0408878593888914,0.),.UNSPECIFIED.) ;
#95=B_SPLINE_CURVE_WITH_KNOTS('',3,(#7827,#7828,#7829,#7830,#7831,#7832),
 .UNSPECIFIED.,.F.,.F.,(4,2,4),(9.99999977697379E-7,7.73756153014981,14.6500515071856),
 .UNSPECIFIED.) ;
#96=B_SPLINE_CURVE_WITH_KNOTS('',3,(#7833,#7834,#7835,#7836,#7837,#7838,
#7839,#7840,#7841,#7842,#7843,#7844,#7845,#7846,#7847,#7848,#7849,#7850,
#7851,#7852,#7853,#7854,#7855,#7856,#7857,#7858,#7859,#7860,#7861,#7862,
#7863,#7864,#7865,#7866,#7867,#7868,#7869,#7870,#7871,#7872,#7873,#7874,
#7875,#7876,#7877,#7878,#7879,#7880,#7881,#7882,#7883,#7884,#7885,#7886,
#7887,#7888,#7889,#7890,#7891,#7892,#7893,#7894,#7895,#7896,#7897,#7898,
#7899,#7900,#7901,#7902,#7903,#7904,#7905,#7906,#7907,#7908,#7909,#7910,
#7911,#7912,#7913,#7914,#7915,#7916,#7917,#7918,#7919,#7920),
 .UNSPECIFIED.,.F.,.F.,(4,3,3,3,3,3,3,3,3,3,3,3,3,3,3,3,3,3,3,3,3,3,3,3,
3,3,3,3,3,4),(0.,0.00937963669820279,0.0180867052587558,0.0187592733964056,
0.0275801848734022,0.0281389100946084,0.0370735108965382,0.0375185467928111,
0.0465678590763102,0.0468981834910139,0.0560614220554001,0.0562778201892167,
0.0655556527434759,0.0750370935856223,0.0750489969011782,0.0844167302838252,
0.0845426524492568,0.0937963669820282,0.0940356196999407,0.103176003680231,
0.103530146128523,0.112555640378434,0.113023868907291,0.121935277076637,
0.122516583962714,0.13131491377484,0.132007368634949,0.140694550473043,
0.141493081370678,0.150074187171246),.UNSPECIFIED.) ;
#97=B_SPLINE_CURVE_WITH_KNOTS('',3,(#7922,#7923,#7924,#7925,#7926,#7927,
#7928,#7929,#7930,#7931,#7932,#7933),.UNSPECIFIED.,.F.,.F.,(4,2,2,2,2,4),
(1.00000000092516E-6,1.57108130900177,3.17385902397466,5.99475439679111,
9.05882250959543,11.9895252463797),.UNSPECIFIED.) ;
#98=B_SPLINE_CURVE_WITH_KNOTS('',3,(#7954,#7955,#7956,#7957,#7958,#7959,
#7960,#7961,#7962,#7963,#7964,#7965,#7966,#7967),.UNSPECIFIED.,.F.,.F.,
(4,2,2,2,2,2,4),(0.,1.73074422377745,3.58539390650711,6.63006683935466,
9.43481756703878,11.4958878534228,13.2600099122431),.UNSPECIFIED.) ;
#99=B_SPLINE_CURVE_WITH_KNOTS('',3,(#8015,#8016,#8017,#8018,#8019,#8020,
#8021,#8022,#8023,#8024,#8025,#8026,#8027,#8028,#8029,#8030,#8031,#8032,
#8033,#8034,#8035,#8036,#8037,#8038,#8039,#8040,#8041,#8042,#8043,#8044,
#8045,#8046,#8047,#8048,#8049,#8050,#8051,#8052,#8053,#8054,#8055,#8056,
#8057,#8058,#8059,#8060,#8061,#8062,#8063,#8064,#8065,#8066,#8067,#8068,
#8069,#8070,#8071,#8072,#8073,#8074,#8075,#8076,#8077,#8078,#8079,#8080,
#8081,#8082,#8083,#8084,#8085,#8086,#8087,#8088,#8089,#8090,#8091,#8092,
#8093,#8094),.UNSPECIFIED.,.F.,.F.,(4,2,2,2,2,2,2,2,2,2,2,2,2,2,2,2,2,2,
2,2,2,2,2,2,2,2,2,2,2,2,2,2,2,2,2,2,2,2,2,4),(-5.99999999998624E-8,0.000590526800460891,
0.00118111360092178,0.00236228720184384,0.00472463440368797,0.00769960210153734,
0.0094493288073765,0.0175309308941643,0.0188987176147537,0.0273655127104343,
0.0372020310641408,0.037797495229508,0.0470416860700575,0.0472468840368852,
0.0566962728442623,0.0568833874626166,0.0661456616516395,0.0667287422857187,
0.0716522046058725,0.0755950504590167,0.0765761128198469,0.0864235312933632,
0.0944938280737709,0.0962698644460282,0.103943216881148,0.106117401685392,
0.113392605688525,0.11596506736434,0.122841994495902,0.125814419594224,
0.132291383303279,0.135667192159144,0.141740772110656,0.145521654063402,
0.146465466514345,0.148827813716189,0.150008786432464,0.150599272790601,
0.1507601426981,0.151189743027067),.UNSPECIFIED.) ;
#100=B_SPLINE_CURVE_WITH_KNOTS('',3,(#8096,#8097,#8098,#8099,#8100,#8101),
 .UNSPECIFIED.,.F.,.F.,(4,2,4),(3.60319807248407E-5,9.64490115778259,19.2897662778294),
 .UNSPECIFIED.) ;
#101=B_SPLINE_CURVE_WITH_KNOTS('',3,(#8103,#8104,#8105,#8106,#8107,#8108,
#8109,#8110,#8111,#8112,#8113,#8114,#8115,#8116),.UNSPECIFIED.,.F.,.F.,
(4,2,2,2,2,2,4),(1.0000000090877E-6,1.76925287661113,3.83874973180625,6.63759802391772,
9.67546855071821,11.5382433292875,13.2752598290998),.UNSPECIFIED.) ;
#102=B_SPLINE_CURVE_WITH_KNOTS('',3,(#8133,#8134,#8135,#8136,#8137,#8138,
#8139,#8140,#8141,#8142,#8143,#8144,#8145,#8146),.UNSPECIFIED.,.F.,.F.,
(4,2,2,2,2,2,4),(1.00000000764925E-6,1.73146141725425,3.58437386659369,
6.63006633376183,9.43722150469471,11.4955948249276,13.2600876640189),
 .UNSPECIFIED.) ;
#103=B_SPLINE_CURVE_WITH_KNOTS('',3,(#8154,#8155,#8156,#8157,#8158,#8159,
#8160,#8161,#8162,#8163,#8164,#8165),.UNSPECIFIED.,.F.,.F.,(4,2,2,2,2,4),
(9.99999885547778E-7,0.136552307551045,0.269611694272923,0.393232608587996,
0.459467944103502,0.515661056065258),.UNSPECIFIED.) ;
#104=B_SPLINE_CURVE_WITH_KNOTS('',3,(#8166,#8167,#8168,#8169,#8170,#8171,
#8172,#8173,#8174,#8175,#8176,#8177,#8178,#8179),.UNSPECIFIED.,.F.,.F.,
(4,2,2,2,2,2,4),(0.,0.0210914408273525,0.0435982414795198,0.0952050288578533,
0.187105593300968,0.287813738141156,0.391818327182591),.UNSPECIFIED.) ;
#105=B_SPLINE_CURVE_WITH_KNOTS('',3,(#8388,#8389,#8390,#8391,#8392,#8393,
#8394,#8395,#8396,#8397,#8398,#8399),.UNSPECIFIED.,.F.,.F.,(4,2,2,2,2,4),
(-0.337170890224052,-0.295474578066957,-0.250449400540881,-0.168586531705906,
-0.080019153547782,0.),.UNSPECIFIED.) ;
#106=B_SPLINE_CURVE_WITH_KNOTS('',3,(#8401,#8402,#8403,#8404,#8405,#8406,
#8407,#8408,#8409,#8410,#8411,#8412),.UNSPECIFIED.,.F.,.F.,(4,2,2,2,2,4),
(-0.333222107941406,-0.254909678914244,-0.166608972882872,-0.0849984861480893,
-0.0408878594487005,0.),.UNSPECIFIED.) ;
#107=B_SPLINE_CURVE_WITH_KNOTS('',3,(#8464,#8465,#8466,#8467,#8468,#8469),
 .UNSPECIFIED.,.F.,.F.,(4,2,4),(9.99999983881963E-7,7.73756066850657,14.6500505458332),
 .UNSPECIFIED.) ;
#108=B_SPLINE_CURVE_WITH_KNOTS('',3,(#8470,#8471,#8472,#8473,#8474,#8475,
#8476,#8477,#8478,#8479,#8480,#8481,#8482,#8483,#8484,#8485,#8486,#8487,
#8488,#8489,#8490,#8491,#8492,#8493,#8494,#8495,#8496,#8497,#8498,#8499,
#8500,#8501,#8502,#8503,#8504,#8505,#8506,#8507,#8508,#8509,#8510,#8511,
#8512,#8513,#8514,#8515,#8516,#8517,#8518,#8519,#8520,#8521,#8522,#8523,
#8524,#8525,#8526,#8527,#8528,#8529,#8530,#8531,#8532,#8533,#8534,#8535,
#8536,#8537,#8538,#8539,#8540,#8541,#8542,#8543,#8544,#8545,#8546,#8547,
#8548,#8549,#8550,#8551,#8552,#8553,#8554,#8555,#8556,#8557),
 .UNSPECIFIED.,.F.,.F.,(4,3,3,3,3,3,3,3,3,3,3,3,3,3,3,3,3,3,3,3,3,3,3,3,
3,3,3,3,3,4),(0.,0.00937963669820289,0.0180867052587603,0.0187592733964058,
0.0275801848734026,0.0281389100946087,0.0370735108965375,0.0375185467928116,
0.0465678590763162,0.0468981834910144,0.0560614220554024,0.0562778201892173,
0.0655556527434056,0.0750370935856231,0.075048996901179,0.0844167302838259,
0.0845426524492572,0.0937963669820288,0.094035619699941,0.103176003680232,
0.103530146128528,0.112555640378434,0.113023868907299,0.121935277076637,
0.122516583962717,0.13131491377484,0.132007368634945,0.140694550473043,
0.141493081370679,0.150074187171246),.UNSPECIFIED.) ;
#109=B_SPLINE_CURVE_WITH_KNOTS('',3,(#8559,#8560,#8561,#8562,#8563,#8564,
#8565,#8566,#8567,#8568,#8569,#8570),.UNSPECIFIED.,.F.,.F.,(4,2,2,2,2,4),
(9.99999976105999E-7,1.57108130900231,3.1738590239761,5.99475439679353,
9.05882250959927,11.9895252463846),.UNSPECIFIED.) ;
#110=B_SPLINE_CURVE_WITH_KNOTS('',3,(#8591,#8592,#8593,#8594,#8595,#8596,
#8597,#8598,#8599,#8600,#8601,#8602,#8603,#8604),.UNSPECIFIED.,.F.,.F.,
(4,2,2,2,2,2,4),(0.,1.73074433286595,3.58539416576586,6.63006684162357,
9.43481733805997,11.4958871896815,13.2600099107624),.UNSPECIFIED.) ;
#111=B_SPLINE_CURVE_WITH_KNOTS('',3,(#8652,#8653,#8654,#8655,#8656,#8657,
#8658,#8659,#8660,#8661,#8662,#8663,#8664,#8665,#8666,#8667,#8668,#8669,
#8670,#8671,#8672,#8673,#8674,#8675,#8676,#8677,#8678,#8679,#8680,#8681,
#8682,#8683,#8684,#8685,#8686,#8687,#8688,#8689,#8690,#8691,#8692,#8693,
#8694,#8695,#8696,#8697,#8698,#8699,#8700,#8701,#8702,#8703,#8704,#8705,
#8706,#8707,#8708,#8709,#8710,#8711,#8712,#8713,#8714,#8715,#8716,#8717,
#8718,#8719,#8720,#8721,#8722,#8723,#8724,#8725,#8726,#8727,#8728,#8729,
#8730,#8731),.UNSPECIFIED.,.F.,.F.,(4,2,2,2,2,2,2,2,2,2,2,2,2,2,2,2,2,2,
2,2,2,2,2,2,2,2,2,2,2,2,2,2,2,2,2,2,2,2,2,4),(-5.99999999998624E-8,0.000590526800461057,
0.00118111360092211,0.00236228720184423,0.00472463440368849,0.00769960210152361,
0.00944932880737713,0.0175309308941517,0.0188987176147546,0.0273655127104255,
0.0372020310641476,0.0377974952295093,0.0470416860700614,0.0472468840368866,
0.056696272844264,0.0568833874626169,0.0661456616516411,0.0667287422857187,
0.0716522046058997,0.0755950504590182,0.0765761128198413,0.0864235312933135,
0.0944938280737723,0.0962698644460061,0.103943216881149,0.106117401685439,
0.113392605688526,0.115965067364374,0.122841994495903,0.125814419594223,
0.13229138330328,0.135667192159117,0.141740772110657,0.14552165406341,0.146465466514345,
0.14882781371619,0.150008786432463,0.1505992727906,0.150760142698144,0.151189743027089),
 .UNSPECIFIED.) ;
#112=B_SPLINE_CURVE_WITH_KNOTS('',3,(#8733,#8734,#8735,#8736,#8737,#8738),
 .UNSPECIFIED.,.F.,.F.,(4,2,4),(3.60319843423254E-5,9.64490065775652,19.2897662777735),
 .UNSPECIFIED.) ;
#113=B_SPLINE_CURVE_WITH_KNOTS('',3,(#8740,#8741,#8742,#8743,#8744,#8745,
#8746,#8747,#8748,#8749,#8750,#8751,#8752,#8753),.UNSPECIFIED.,.F.,.F.,
(4,2,2,2,2,2,4),(1.00000000329695E-6,1.76925353789123,3.83874996049991,
6.63759802407595,9.67546829683264,11.5382432249431,13.2752598328519),
 .UNSPECIFIED.) ;
#114=B_SPLINE_CURVE_WITH_KNOTS('',3,(#8770,#8771,#8772,#8773,#8774,#8775,
#8776,#8777,#8778,#8779,#8780,#8781,#8782,#8783),.UNSPECIFIED.,.F.,.F.,
(4,2,2,2,2,2,4),(9.99999971167725E-7,1.73146228667713,3.58437459628016,
6.63006683375916,9.43722179299249,11.4955949579948,13.2600876640179),
 .UNSPECIFIED.) ;
#115=B_SPLINE_CURVE_WITH_KNOTS('',3,(#8791,#8792,#8793,#8794,#8795,#8796,
#8797,#8798,#8799,#8800,#8801,#8802),.UNSPECIFIED.,.F.,.F.,(4,2,2,2,2,4),
(9.99999764585794E-7,0.136553042381969,0.269612170499918,0.393232844695364,
0.459468051520106,0.515661054333012),.UNSPECIFIED.) ;
#116=B_SPLINE_CURVE_WITH_KNOTS('',3,(#8803,#8804,#8805,#8806,#8807,#8808,
#8809,#8810,#8811,#8812,#8813,#8814,#8815,#8816),.UNSPECIFIED.,.F.,.F.,
(4,2,2,2,2,2,4),(0.,0.0210914409585585,0.0435982416633199,0.0952050281507284,
0.187105593156084,0.28781486856457,0.391819686950129),.UNSPECIFIED.) ;
#117=B_SPLINE_CURVE_WITH_KNOTS('',3,(#9025,#9026,#9027,#9028,#9029,#9030,
#9031,#9032,#9033,#9034,#9035,#9036),.UNSPECIFIED.,.F.,.F.,(4,2,2,2,2,4),
(-0.337170890167228,-0.295474578027858,-0.250449400520224,-0.16858653167804,
-0.080019153500057,0.),.UNSPECIFIED.) ;
#118=B_SPLINE_CURVE_WITH_KNOTS('',3,(#9038,#9039,#9040,#9041,#9042,#9043,
#9044,#9045,#9046,#9047,#9048,#9049),.UNSPECIFIED.,.F.,.F.,(4,2,2,2,2,4),
(-0.333222107943548,-0.254909679200476,-0.166608972885045,-0.084998486181255,
-0.0408878594089353,0.),.UNSPECIFIED.) ;
#119=B_SPLINE_CURVE_WITH_KNOTS('',3,(#9101,#9102,#9103,#9104,#9105,#9106),
 .UNSPECIFIED.,.F.,.F.,(4,2,4),(9.99999993528995E-7,7.73756066846338,14.6500505457511),
 .UNSPECIFIED.) ;
#120=B_SPLINE_CURVE_WITH_KNOTS('',3,(#9107,#9108,#9109,#9110,#9111,#9112,
#9113,#9114,#9115,#9116,#9117,#9118,#9119,#9120,#9121,#9122,#9123,#9124,
#9125,#9126,#9127,#9128,#9129,#9130,#9131,#9132,#9133,#9134,#9135,#9136,
#9137,#9138,#9139,#9140,#9141,#9142,#9143,#9144,#9145,#9146,#9147,#9148,
#9149,#9150,#9151,#9152,#9153,#9154,#9155,#9156,#9157,#9158,#9159,#9160,
#9161,#9162,#9163,#9164,#9165,#9166,#9167,#9168,#9169,#9170,#9171,#9172,
#9173,#9174,#9175,#9176,#9177,#9178,#9179,#9180,#9181,#9182,#9183,#9184,
#9185,#9186,#9187,#9188,#9189,#9190,#9191,#9192,#9193,#9194),
 .UNSPECIFIED.,.F.,.F.,(4,3,3,3,3,3,3,3,3,3,3,3,3,3,3,3,3,3,3,3,3,3,3,3,
3,3,3,3,3,4),(0.,0.00937963669820283,0.0180867052587627,0.0187592733964057,
0.0275801848734053,0.0281389100946085,0.0370735108965416,0.0375185467928113,
0.0465678590763129,0.0468981834910141,0.0560614220553998,0.056277820189217,
0.0655556527432504,0.0750370935856224,0.0750489969011785,0.0844167302838252,
0.0845426524492565,0.093796366982028,0.0940356196999399,0.103176003680231,
0.103530146128525,0.112555640378434,0.113023868907302,0.121935277076637,
0.122516583962714,0.13131491377484,0.132007368634939,0.140694550473043,
0.14149308137069,0.150074187171246),.UNSPECIFIED.) ;
#121=B_SPLINE_CURVE_WITH_KNOTS('',3,(#9196,#9197,#9198,#9199,#9200,#9201,
#9202,#9203,#9204,#9205,#9206,#9207),.UNSPECIFIED.,.F.,.F.,(4,2,2,2,2,4),
(9.99999992923776E-7,1.57108130900183,3.17385902397465,5.99475439679217,
9.05882250959655,11.9895252463801),.UNSPECIFIED.) ;
#122=B_SPLINE_CURVE_WITH_KNOTS('',3,(#9228,#9229,#9230,#9231,#9232,#9233,
#9234,#9235,#9236,#9237,#9238,#9239,#9240,#9241),.UNSPECIFIED.,.F.,.F.,
(4,2,2,2,2,2,4),(0.,1.7307444637883,3.58539443698107,6.63006734314984,9.43481805174913,
11.4958880592783,13.2600099107283),.UNSPECIFIED.) ;
#123=B_SPLINE_CURVE_WITH_KNOTS('',3,(#9289,#9290,#9291,#9292,#9293,#9294,
#9295,#9296,#9297,#9298,#9299,#9300,#9301,#9302,#9303,#9304,#9305,#9306,
#9307,#9308,#9309,#9310,#9311,#9312,#9313,#9314,#9315,#9316,#9317,#9318,
#9319,#9320,#9321,#9322,#9323,#9324,#9325,#9326,#9327,#9328,#9329,#9330,
#9331,#9332,#9333,#9334,#9335,#9336,#9337,#9338,#9339,#9340,#9341,#9342,
#9343,#9344,#9345,#9346,#9347,#9348,#9349,#9350,#9351,#9352,#9353,#9354,
#9355,#9356,#9357,#9358,#9359,#9360,#9361,#9362,#9363,#9364,#9365,#9366,
#9367,#9368),.UNSPECIFIED.,.F.,.F.,(4,2,2,2,2,2,2,2,2,2,2,2,2,2,2,2,2,2,
2,2,2,2,2,2,2,2,2,2,2,2,2,2,2,2,2,2,2,2,2,4),(-5.99999999998624E-8,0.000590526800460957,
0.00118111360092191,0.00236228720184402,0.00472463440368833,0.00769960210154686,
0.0094493288073769,0.0175309308941876,0.0188987176147541,0.0273655127104106,
0.037202031064141,0.0377974952295082,0.0470416860700587,0.0472468840368852,
0.0566962728442623,0.0568833874626161,0.0661456616516395,0.0667287422857284,
0.0716522046057163,0.0755950504590167,0.0765761128198456,0.0864235312934359,
0.0944938280737711,0.0962698644460588,0.103943216881148,0.106117401685479,
0.113392605688525,0.115965067364307,0.122841994495902,0.125814419594179,
0.132291383303279,0.135667192159113,0.141740772110656,0.145521654063399,
0.146465466514345,0.148827813716189,0.150008786432465,0.150599272790602,
0.150760142698105,0.151189743027079),.UNSPECIFIED.) ;
#124=B_SPLINE_CURVE_WITH_KNOTS('',3,(#9370,#9371,#9372,#9373,#9374,#9375),
 .UNSPECIFIED.,.F.,.F.,(4,2,4),(3.60319821137706E-5,9.64490115776887,19.2897662778005),
 .UNSPECIFIED.) ;
#125=B_SPLINE_CURVE_WITH_KNOTS('',3,(#9377,#9378,#9379,#9380,#9381,#9382,
#9383,#9384,#9385,#9386,#9387,#9388,#9389,#9390),.UNSPECIFIED.,.F.,.F.,
(4,2,2,2,2,2,4),(9.99999999267761E-7,1.76925387621167,3.83875073094035,
6.63759902242126,9.67546954853661,11.5382443266855,13.2752598291039),
 .UNSPECIFIED.) ;
#126=B_SPLINE_CURVE_WITH_KNOTS('',3,(#9407,#9408,#9409,#9410,#9411,#9412,
#9413,#9414,#9415,#9416,#9417,#9418,#9419,#9420),.UNSPECIFIED.,.F.,.F.,
(4,2,2,2,2,2,4),(1.00000000421862E-6,1.7314614172568,3.58437386659518,6.63006633376352,
9.43722150469613,11.4955948249291,13.2600876640204),.UNSPECIFIED.) ;
#127=B_SPLINE_CURVE_WITH_KNOTS('',3,(#9428,#9429,#9430,#9431,#9432,#9433,
#9434,#9435,#9436,#9437,#9438,#9439),.UNSPECIFIED.,.F.,.F.,(4,2,2,2,2,4),
(1.45423872814327E-6,0.13669579668315,0.269968128958899,0.393732693269049,
0.460063012540498,0.516324865414279),.UNSPECIFIED.) ;
#128=B_SPLINE_CURVE_WITH_KNOTS('',3,(#9440,#9441,#9442,#9443,#9444,#9445,
#9446,#9447,#9448,#9449,#9450,#9451,#9452,#9453),.UNSPECIFIED.,.F.,.F.,
(4,2,2,2,2,2,4),(0.,0.0210914408313759,0.0435982414838107,0.0952050288584094,
0.187105593266359,0.287813738105342,0.391818327152263),.UNSPECIFIED.) ;
#129=CYLINDRICAL_SURFACE('',#4087,7.6) ;
#130=CYLINDRICAL_SURFACE('',#4100,7.) ;
#131=CYLINDRICAL_SURFACE('',#4101,35.0001428568513) ;
#132=CYLINDRICAL_SURFACE('',#4102,7.) ;
#133=CYLINDRICAL_SURFACE('',#4109,7.00000000000001) ;
#134=CYLINDRICAL_SURFACE('',#4110,35.0001428568513) ;
#135=CYLINDRICAL_SURFACE('',#4111,6.99999999999999) ;
#136=CYLINDRICAL_SURFACE('',#4118,7.) ;
#137=CYLINDRICAL_SURFACE('',#4119,35.0001428568513) ;
#138=CYLINDRICAL_SURFACE('',#4120,7.) ;
#139=CYLINDRICAL_SURFACE('',#4126,7.) ;
#140=CYLINDRICAL_SURFACE('',#4127,35.0001428568513) ;
#141=CYLINDRICAL_SURFACE('',#4128,7.) ;
#142=CYLINDRICAL_SURFACE('',#4134,7.) ;
#143=CYLINDRICAL_SURFACE('',#4135,35.0001428568513) ;
#144=CYLINDRICAL_SURFACE('',#4136,6.99999999999999) ;
#356=SHAPE_REPRESENTATION_RELATIONSHIP('SRR','None',#10473,#388) ;
#388=ADVANCED_BREP_SHAPE_REPRESENTATION('',(#460),#10325) ;
#428=STYLED_ITEM('',(#10633),#460) ;
#460=MANIFOLD_SOLID_BREP('Body1',#3582) ;
#469=FACE_BOUND('',#1082,.T.) ;
#470=FACE_BOUND('',#1083,.T.) ;
#471=FACE_BOUND('',#1084,.T.) ;
#472=FACE_BOUND('',#1085,.T.) ;
#478=PLANE('',#4096) ;
#479=PLANE('',#4103) ;
#480=PLANE('',#4104) ;
#481=PLANE('',#4105) ;
#482=PLANE('',#4112) ;
#483=PLANE('',#4113) ;
#484=PLANE('',#4114) ;
#485=PLANE('',#4121) ;
#486=PLANE('',#4122) ;
#487=PLANE('',#4129) ;
#488=PLANE('',#4130) ;
#489=PLANE('',#4137) ;
#535=LINE('',#5791,#693) ;
#536=LINE('',#5800,#694) ;
#537=LINE('',#5867,#695) ;
#538=LINE('',#5958,#696) ;
#539=LINE('',#6143,#697) ;
#540=LINE('',#6275,#698) ;
#541=LINE('',#6405,#699) ;
#542=LINE('',#6474,#700) ;
#543=LINE('',#6501,#701) ;
#544=LINE('',#6872,#702) ;
#545=LINE('',#6874,#703) ;
#546=LINE('',#6876,#704) ;
#547=LINE('',#7112,#705) ;
#548=LINE('',#7139,#706) ;
#549=LINE('',#7510,#707) ;
#550=LINE('',#7512,#708) ;
#551=LINE('',#7514,#709) ;
#552=LINE('',#7750,#710) ;
#553=LINE('',#7777,#711) ;
#554=LINE('',#8148,#712) ;
#555=LINE('',#8150,#713) ;
#556=LINE('',#8152,#714) ;
#557=LINE('',#8387,#715) ;
#558=LINE('',#8414,#716) ;
#559=LINE('',#8785,#717) ;
#560=LINE('',#8787,#718) ;
#561=LINE('',#8789,#719) ;
#562=LINE('',#9024,#720) ;
#563=LINE('',#9051,#721) ;
#564=LINE('',#9422,#722) ;
#565=LINE('',#9424,#723) ;
#566=LINE('',#9426,#724) ;
#693=VECTOR('',#4739,7.6) ;
#694=VECTOR('',#4742,7.6) ;
#695=VECTOR('',#4747,100.) ;
#696=VECTOR('',#4748,100.) ;
#697=VECTOR('',#4751,100.) ;
#698=VECTOR('',#4754,100.) ;
#699=VECTOR('',#4757,100.) ;
#700=VECTOR('',#4762,1.) ;
#701=VECTOR('',#4763,1.) ;
#702=VECTOR('',#4772,100.) ;
#703=VECTOR('',#4775,100.) ;
#704=VECTOR('',#4778,100.) ;
#705=VECTOR('',#4785,1.) ;
#706=VECTOR('',#4786,1.) ;
#707=VECTOR('',#4795,100.) ;
#708=VECTOR('',#4798,100.) ;
#709=VECTOR('',#4801,100.) ;
#710=VECTOR('',#4808,1.) ;
#711=VECTOR('',#4809,1.) ;
#712=VECTOR('',#4818,100.) ;
#713=VECTOR('',#4821,100.) ;
#714=VECTOR('',#4824,100.) ;
#715=VECTOR('',#4829,1.) ;
#716=VECTOR('',#4830,1.) ;
#717=VECTOR('',#4839,100.) ;
#718=VECTOR('',#4842,100.) ;
#719=VECTOR('',#4845,100.) ;
#720=VECTOR('',#4850,1.) ;
#721=VECTOR('',#4851,1.) ;
#722=VECTOR('',#4860,100.) ;
#723=VECTOR('',#4863,100.) ;
#724=VECTOR('',#4866,100.) ;
#881=FACE_OUTER_BOUND('',#1081,.T.) ;
#882=FACE_OUTER_BOUND('',#1086,.T.) ;
#883=FACE_OUTER_BOUND('',#1087,.T.) ;
#884=FACE_OUTER_BOUND('',#1088,.T.) ;
#885=FACE_OUTER_BOUND('',#1089,.T.) ;
#886=FACE_OUTER_BOUND('',#1090,.T.) ;
#887=FACE_OUTER_BOUND('',#1091,.T.) ;
#888=FACE_OUTER_BOUND('',#1092,.T.) ;
#889=FACE_OUTER_BOUND('',#1093,.T.) ;
#890=FACE_OUTER_BOUND('',#1094,.T.) ;
#891=FACE_OUTER_BOUND('',#1095,.T.) ;
#892=FACE_OUTER_BOUND('',#1096,.T.) ;
#893=FACE_OUTER_BOUND('',#1097,.T.) ;
#894=FACE_OUTER_BOUND('',#1098,.T.) ;
#895=FACE_OUTER_BOUND('',#1099,.T.) ;
#896=FACE_OUTER_BOUND('',#1100,.T.) ;
#897=FACE_OUTER_BOUND('',#1101,.T.) ;
#898=FACE_OUTER_BOUND('',#1102,.T.) ;
#899=FACE_OUTER_BOUND('',#1103,.T.) ;
#900=FACE_OUTER_BOUND('',#1104,.T.) ;
#901=FACE_OUTER_BOUND('',#1105,.T.) ;
#902=FACE_OUTER_BOUND('',#1106,.T.) ;
#903=FACE_OUTER_BOUND('',#1107,.T.) ;
#904=FACE_OUTER_BOUND('',#1108,.T.) ;
#905=FACE_OUTER_BOUND('',#1109,.T.) ;
#906=FACE_OUTER_BOUND('',#1110,.T.) ;
#907=FACE_OUTER_BOUND('',#1111,.T.) ;
#908=FACE_OUTER_BOUND('',#1112,.T.) ;
#909=FACE_OUTER_BOUND('',#1113,.T.) ;
#910=FACE_OUTER_BOUND('',#1114,.T.) ;
#911=FACE_OUTER_BOUND('',#1115,.T.) ;
#912=FACE_OUTER_BOUND('',#1116,.T.) ;
#913=FACE_OUTER_BOUND('',#1117,.T.) ;
#914=FACE_OUTER_BOUND('',#1118,.T.) ;
#915=FACE_OUTER_BOUND('',#1119,.T.) ;
#916=FACE_OUTER_BOUND('',#1120,.T.) ;
#917=FACE_OUTER_BOUND('',#1121,.T.) ;
#918=FACE_OUTER_BOUND('',#1122,.T.) ;
#919=FACE_OUTER_BOUND('',#1123,.T.) ;
#920=FACE_OUTER_BOUND('',#1124,.T.) ;
#921=FACE_OUTER_BOUND('',#1125,.T.) ;
#922=FACE_OUTER_BOUND('',#1126,.T.) ;
#923=FACE_OUTER_BOUND('',#1127,.T.) ;
#924=FACE_OUTER_BOUND('',#1128,.T.) ;
#925=FACE_OUTER_BOUND('',#1129,.T.) ;
#926=FACE_OUTER_BOUND('',#1130,.T.) ;
#927=FACE_OUTER_BOUND('',#1131,.T.) ;
#928=FACE_OUTER_BOUND('',#1132,.T.) ;
#1081=EDGE_LOOP('',(#2437,#2438,#2439,#2440,#2441,#2442,#2443,#2444,#2445,
#2446,#2447,#2448,#2449)) ;
#1082=EDGE_LOOP('',(#2450,#2451,#2452,#2453,#2454,#2455,#2456)) ;
#1083=EDGE_LOOP('',(#2457,#2458,#2459,#2460,#2461)) ;
#1084=EDGE_LOOP('',(#2462,#2463,#2464,#2465,#2466)) ;
#1085=EDGE_LOOP('',(#2467,#2468,#2469,#2470,#2471)) ;
#1086=EDGE_LOOP('',(#2472,#2473,#2474,#2475,#2476,#2477,#2478)) ;
#1087=EDGE_LOOP('',(#2479,#2480,#2481,#2482,#2483,#2484,#2485,#2486)) ;
#1088=EDGE_LOOP('',(#2487,#2488,#2489,#2490,#2491,#2492)) ;
#1089=EDGE_LOOP('',(#2493,#2494,#2495,#2496,#2497)) ;
#1090=EDGE_LOOP('',(#2498,#2499,#2500,#2501)) ;
#1091=EDGE_LOOP('',(#2502,#2503,#2504,#2505,#2506)) ;
#1092=EDGE_LOOP('',(#2507,#2508,#2509,#2510,#2511,#2512)) ;
#1093=EDGE_LOOP('',(#2513)) ;
#1094=EDGE_LOOP('',(#2514,#2515,#2516,#2517,#2518)) ;
#1095=EDGE_LOOP('',(#2519,#2520,#2521,#2522,#2523)) ;
#1096=EDGE_LOOP('',(#2524,#2525,#2526,#2527,#2528,#2529)) ;
#1097=EDGE_LOOP('',(#2530,#2531,#2532,#2533,#2534,#2535,#2536,#2537)) ;
#1098=EDGE_LOOP('',(#2538,#2539,#2540,#2541,#2542,#2543)) ;
#1099=EDGE_LOOP('',(#2544,#2545,#2546,#2547,#2548)) ;
#1100=EDGE_LOOP('',(#2549,#2550,#2551,#2552)) ;
#1101=EDGE_LOOP('',(#2553,#2554,#2555,#2556,#2557)) ;
#1102=EDGE_LOOP('',(#2558,#2559,#2560,#2561,#2562,#2563)) ;
#1103=EDGE_LOOP('',(#2564,#2565,#2566,#2567,#2568)) ;
#1104=EDGE_LOOP('',(#2569,#2570,#2571,#2572)) ;
#1105=EDGE_LOOP('',(#2573)) ;
#1106=EDGE_LOOP('',(#2574,#2575,#2576,#2577,#2578,#2579)) ;
#1107=EDGE_LOOP('',(#2580,#2581,#2582,#2583,#2584,#2585,#2586,#2587)) ;
#1108=EDGE_LOOP('',(#2588,#2589,#2590,#2591,#2592,#2593)) ;
#1109=EDGE_LOOP('',(#2594,#2595,#2596,#2597,#2598)) ;
#1110=EDGE_LOOP('',(#2599,#2600,#2601,#2602)) ;
#1111=EDGE_LOOP('',(#2603,#2604,#2605,#2606,#2607)) ;
#1112=EDGE_LOOP('',(#2608,#2609,#2610,#2611,#2612,#2613)) ;
#1113=EDGE_LOOP('',(#2614,#2615,#2616,#2617,#2618)) ;
#1114=EDGE_LOOP('',(#2619,#2620,#2621,#2622)) ;
#1115=EDGE_LOOP('',(#2623,#2624,#2625,#2626,#2627,#2628)) ;
#1116=EDGE_LOOP('',(#2629,#2630,#2631,#2632,#2633,#2634,#2635,#2636)) ;
#1117=EDGE_LOOP('',(#2637,#2638,#2639,#2640,#2641,#2642)) ;
#1118=EDGE_LOOP('',(#2643,#2644,#2645,#2646,#2647)) ;
#1119=EDGE_LOOP('',(#2648,#2649,#2650,#2651)) ;
#1120=EDGE_LOOP('',(#2652,#2653,#2654,#2655,#2656)) ;
#1121=EDGE_LOOP('',(#2657,#2658,#2659,#2660,#2661,#2662)) ;
#1122=EDGE_LOOP('',(#2663,#2664,#2665,#2666,#2667,#2668)) ;
#1123=EDGE_LOOP('',(#2669,#2670,#2671,#2672,#2673)) ;
#1124=EDGE_LOOP('',(#2674,#2675,#2676,#2677,#2678,#2679)) ;
#1125=EDGE_LOOP('',(#2680,#2681,#2682,#2683,#2684,#2685,#2686,#2687)) ;
#1126=EDGE_LOOP('',(#2688,#2689,#2690,#2691,#2692,#2693)) ;
#1127=EDGE_LOOP('',(#2694,#2695,#2696,#2697,#2698)) ;
#1128=EDGE_LOOP('',(#2699,#2700,#2701,#2702)) ;
#1129=EDGE_LOOP('',(#2703,#2704,#2705,#2706,#2707)) ;
#1130=EDGE_LOOP('',(#2708,#2709,#2710,#2711,#2712,#2713)) ;
#1131=EDGE_LOOP('',(#2714,#2715,#2716,#2717,#2718)) ;
#1132=EDGE_LOOP('',(#2719,#2720,#2721,#2722)) ;
#1320=CIRCLE('',#4088,7.6) ;
#1321=CIRCLE('',#4089,7.6) ;
#1322=CIRCLE('',#4090,7.6) ;
#1323=CIRCLE('',#4091,7.6) ;
#1324=CIRCLE('',#4092,7.6) ;
#1325=CIRCLE('',#4093,7.6) ;
#1326=CIRCLE('',#4094,7.60000000000001) ;
#1327=CIRCLE('',#4095,7.6) ;
#1328=CIRCLE('',#4097,7.) ;
#1329=CIRCLE('',#4106,7.00000000000001) ;
#1330=CIRCLE('',#4115,7.) ;
#1331=CIRCLE('',#4123,7.) ;
#1332=CIRCLE('',#4131,7.) ;
#1535=VERTEX_POINT('',#5788) ;
#1536=VERTEX_POINT('',#5790) ;
#1537=VERTEX_POINT('',#5792) ;
#1538=VERTEX_POINT('',#5797) ;
#1539=VERTEX_POINT('',#5799) ;
#1540=VERTEX_POINT('',#5802) ;
#1541=VERTEX_POINT('',#5804) ;
#1542=VERTEX_POINT('',#5861) ;
#1543=VERTEX_POINT('',#5866) ;
#1544=VERTEX_POINT('',#5930) ;
#1545=VERTEX_POINT('',#5931) ;
#1546=VERTEX_POINT('',#5952) ;
#1547=VERTEX_POINT('',#5957) ;
#1548=VERTEX_POINT('',#5959) ;
#1549=VERTEX_POINT('',#5978) ;
#1550=VERTEX_POINT('',#6040) ;
#1551=VERTEX_POINT('',#6079) ;
#1552=VERTEX_POINT('',#6080) ;
#1553=VERTEX_POINT('',#6137) ;
#1554=VERTEX_POINT('',#6142) ;
#1555=VERTEX_POINT('',#6144) ;
#1556=VERTEX_POINT('',#6210) ;
#1557=VERTEX_POINT('',#6211) ;
#1558=VERTEX_POINT('',#6269) ;
#1559=VERTEX_POINT('',#6274) ;
#1560=VERTEX_POINT('',#6276) ;
#1561=VERTEX_POINT('',#6341) ;
#1562=VERTEX_POINT('',#6342) ;
#1563=VERTEX_POINT('',#6399) ;
#1564=VERTEX_POINT('',#6404) ;
#1565=VERTEX_POINT('',#6406) ;
#1566=VERTEX_POINT('',#6472) ;
#1567=VERTEX_POINT('',#6473) ;
#1568=VERTEX_POINT('',#6487) ;
#1569=VERTEX_POINT('',#6500) ;
#1570=VERTEX_POINT('',#6549) ;
#1571=VERTEX_POINT('',#6550) ;
#1572=VERTEX_POINT('',#6645) ;
#1573=VERTEX_POINT('',#6658) ;
#1574=VERTEX_POINT('',#6660) ;
#1575=VERTEX_POINT('',#6676) ;
#1576=VERTEX_POINT('',#6738) ;
#1577=VERTEX_POINT('',#6819) ;
#1578=VERTEX_POINT('',#6826) ;
#1579=VERTEX_POINT('',#6841) ;
#1580=VERTEX_POINT('',#7110) ;
#1581=VERTEX_POINT('',#7111) ;
#1582=VERTEX_POINT('',#7125) ;
#1583=VERTEX_POINT('',#7138) ;
#1584=VERTEX_POINT('',#7187) ;
#1585=VERTEX_POINT('',#7188) ;
#1586=VERTEX_POINT('',#7283) ;
#1587=VERTEX_POINT('',#7296) ;
#1588=VERTEX_POINT('',#7298) ;
#1589=VERTEX_POINT('',#7314) ;
#1590=VERTEX_POINT('',#7376) ;
#1591=VERTEX_POINT('',#7457) ;
#1592=VERTEX_POINT('',#7464) ;
#1593=VERTEX_POINT('',#7479) ;
#1594=VERTEX_POINT('',#7748) ;
#1595=VERTEX_POINT('',#7749) ;
#1596=VERTEX_POINT('',#7763) ;
#1597=VERTEX_POINT('',#7776) ;
#1598=VERTEX_POINT('',#7825) ;
#1599=VERTEX_POINT('',#7826) ;
#1600=VERTEX_POINT('',#7921) ;
#1601=VERTEX_POINT('',#7934) ;
#1602=VERTEX_POINT('',#7936) ;
#1603=VERTEX_POINT('',#7952) ;
#1604=VERTEX_POINT('',#8014) ;
#1605=VERTEX_POINT('',#8095) ;
#1606=VERTEX_POINT('',#8102) ;
#1607=VERTEX_POINT('',#8117) ;
#1608=VERTEX_POINT('',#8385) ;
#1609=VERTEX_POINT('',#8386) ;
#1610=VERTEX_POINT('',#8400) ;
#1611=VERTEX_POINT('',#8413) ;
#1612=VERTEX_POINT('',#8462) ;
#1613=VERTEX_POINT('',#8463) ;
#1614=VERTEX_POINT('',#8558) ;
#1615=VERTEX_POINT('',#8571) ;
#1616=VERTEX_POINT('',#8573) ;
#1617=VERTEX_POINT('',#8589) ;
#1618=VERTEX_POINT('',#8651) ;
#1619=VERTEX_POINT('',#8732) ;
#1620=VERTEX_POINT('',#8739) ;
#1621=VERTEX_POINT('',#8754) ;
#1622=VERTEX_POINT('',#9022) ;
#1623=VERTEX_POINT('',#9023) ;
#1624=VERTEX_POINT('',#9037) ;
#1625=VERTEX_POINT('',#9050) ;
#1626=VERTEX_POINT('',#9099) ;
#1627=VERTEX_POINT('',#9100) ;
#1628=VERTEX_POINT('',#9195) ;
#1629=VERTEX_POINT('',#9208) ;
#1630=VERTEX_POINT('',#9210) ;
#1631=VERTEX_POINT('',#9226) ;
#1632=VERTEX_POINT('',#9288) ;
#1633=VERTEX_POINT('',#9369) ;
#1634=VERTEX_POINT('',#9376) ;
#1635=VERTEX_POINT('',#9391) ;
#1875=EDGE_CURVE('',#1535,#1535,#1320,.T.) ;
#1876=EDGE_CURVE('',#1535,#1536,#535,.T.) ;
#1877=EDGE_CURVE('',#1536,#1537,#51,.T.) ;
#1878=EDGE_CURVE('',#1538,#1537,#1321,.T.) ;
#1879=EDGE_CURVE('',#1538,#1539,#536,.T.) ;
#1880=EDGE_CURVE('',#1539,#1539,#1322,.T.) ;
#1881=EDGE_CURVE('',#1540,#1538,#1323,.T.) ;
#1882=EDGE_CURVE('',#1540,#1541,#52,.T.) ;
#1883=EDGE_CURVE('',#1541,#1542,#53,.T.) ;
#1884=EDGE_CURVE('',#1542,#1543,#537,.T.) ;
#1885=EDGE_CURVE('',#1543,#1536,#54,.T.) ;
#1886=EDGE_CURVE('',#1544,#1545,#55,.T.) ;
#1887=EDGE_CURVE('',#1545,#1546,#56,.T.) ;
#1888=EDGE_CURVE('',#1546,#1547,#538,.T.) ;
#1889=EDGE_CURVE('',#1547,#1548,#57,.T.) ;
#1890=EDGE_CURVE('',#1548,#1549,#58,.T.) ;
#1891=EDGE_CURVE('',#1550,#1549,#1324,.T.) ;
#1892=EDGE_CURVE('',#1550,#1544,#59,.T.) ;
#1893=EDGE_CURVE('',#1551,#1552,#60,.T.) ;
#1894=EDGE_CURVE('',#1552,#1553,#61,.T.) ;
#1895=EDGE_CURVE('',#1553,#1554,#539,.T.) ;
#1896=EDGE_CURVE('',#1554,#1555,#62,.T.) ;
#1897=EDGE_CURVE('',#1551,#1555,#1325,.T.) ;
#1898=EDGE_CURVE('',#1556,#1557,#63,.T.) ;
#1899=EDGE_CURVE('',#1557,#1558,#64,.T.) ;
#1900=EDGE_CURVE('',#1558,#1559,#540,.T.) ;
#1901=EDGE_CURVE('',#1559,#1560,#65,.T.) ;
#1902=EDGE_CURVE('',#1556,#1560,#1326,.T.) ;
#1903=EDGE_CURVE('',#1561,#1562,#66,.T.) ;
#1904=EDGE_CURVE('',#1562,#1563,#67,.T.) ;
#1905=EDGE_CURVE('',#1563,#1564,#541,.T.) ;
#1906=EDGE_CURVE('',#1564,#1565,#68,.T.) ;
#1907=EDGE_CURVE('',#1561,#1565,#1327,.T.) ;
#1908=EDGE_CURVE('',#1566,#1567,#542,.T.) ;
#1909=EDGE_CURVE('',#1566,#1540,#69,.T.) ;
#1910=EDGE_CURVE('',#1537,#1568,#70,.T.) ;
#1911=EDGE_CURVE('',#1569,#1568,#543,.T.) ;
#1912=EDGE_CURVE('',#1567,#1569,#1328,.T.) ;
#1913=EDGE_CURVE('',#1570,#1571,#71,.T.) ;
#1914=EDGE_CURVE('',#1571,#1566,#72,.T.) ;
#1915=EDGE_CURVE('',#1567,#1572,#73,.T.) ;
#1916=EDGE_CURVE('',#1572,#1573,#21,.T.) ;
#1917=EDGE_CURVE('',#1573,#1574,#11,.T.) ;
#1918=EDGE_CURVE('',#1574,#1575,#22,.T.) ;
#1919=EDGE_CURVE('',#1575,#1570,#74,.T.) ;
#1920=EDGE_CURVE('',#1568,#1576,#75,.T.) ;
#1921=EDGE_CURVE('',#1576,#1577,#76,.T.) ;
#1922=EDGE_CURVE('',#1577,#1578,#77,.T.) ;
#1923=EDGE_CURVE('',#1579,#1578,#12,.T.) ;
#1924=EDGE_CURVE('',#1579,#1569,#78,.T.) ;
#1925=EDGE_CURVE('',#1573,#1579,#544,.T.) ;
#1926=EDGE_CURVE('',#1574,#1578,#545,.T.) ;
#1927=EDGE_CURVE('',#1570,#1577,#546,.T.) ;
#1928=EDGE_CURVE('',#1542,#1571,#79,.T.) ;
#1929=EDGE_CURVE('',#1576,#1543,#80,.T.) ;
#1930=EDGE_CURVE('',#1580,#1581,#547,.T.) ;
#1931=EDGE_CURVE('',#1580,#1551,#81,.T.) ;
#1932=EDGE_CURVE('',#1555,#1582,#82,.T.) ;
#1933=EDGE_CURVE('',#1583,#1582,#548,.T.) ;
#1934=EDGE_CURVE('',#1581,#1583,#1329,.T.) ;
#1935=EDGE_CURVE('',#1584,#1585,#83,.T.) ;
#1936=EDGE_CURVE('',#1585,#1580,#84,.T.) ;
#1937=EDGE_CURVE('',#1581,#1586,#85,.T.) ;
#1938=EDGE_CURVE('',#1586,#1587,#23,.T.) ;
#1939=EDGE_CURVE('',#1587,#1588,#13,.T.) ;
#1940=EDGE_CURVE('',#1588,#1589,#24,.T.) ;
#1941=EDGE_CURVE('',#1589,#1584,#86,.T.) ;
#1942=EDGE_CURVE('',#1582,#1590,#87,.T.) ;
#1943=EDGE_CURVE('',#1590,#1591,#88,.T.) ;
#1944=EDGE_CURVE('',#1591,#1592,#89,.T.) ;
#1945=EDGE_CURVE('',#1593,#1592,#14,.T.) ;
#1946=EDGE_CURVE('',#1593,#1583,#90,.T.) ;
#1947=EDGE_CURVE('',#1587,#1593,#549,.T.) ;
#1948=EDGE_CURVE('',#1588,#1592,#550,.T.) ;
#1949=EDGE_CURVE('',#1584,#1591,#551,.T.) ;
#1950=EDGE_CURVE('',#1553,#1585,#91,.T.) ;
#1951=EDGE_CURVE('',#1590,#1554,#92,.T.) ;
#1952=EDGE_CURVE('',#1594,#1595,#552,.T.) ;
#1953=EDGE_CURVE('',#1594,#1556,#93,.T.) ;
#1954=EDGE_CURVE('',#1560,#1596,#94,.T.) ;
#1955=EDGE_CURVE('',#1597,#1596,#553,.T.) ;
#1956=EDGE_CURVE('',#1595,#1597,#1330,.T.) ;
#1957=EDGE_CURVE('',#1598,#1599,#95,.T.) ;
#1958=EDGE_CURVE('',#1599,#1594,#96,.T.) ;
#1959=EDGE_CURVE('',#1595,#1600,#97,.T.) ;
#1960=EDGE_CURVE('',#1600,#1601,#25,.T.) ;
#1961=EDGE_CURVE('',#1601,#1602,#15,.T.) ;
#1962=EDGE_CURVE('',#1602,#1603,#26,.T.) ;
#1963=EDGE_CURVE('',#1603,#1598,#98,.T.) ;
#1964=EDGE_CURVE('',#1596,#1604,#99,.T.) ;
#1965=EDGE_CURVE('',#1604,#1605,#100,.T.) ;
#1966=EDGE_CURVE('',#1605,#1606,#101,.T.) ;
#1967=EDGE_CURVE('',#1607,#1606,#16,.T.) ;
#1968=EDGE_CURVE('',#1607,#1597,#102,.T.) ;
#1969=EDGE_CURVE('',#1601,#1607,#554,.T.) ;
#1970=EDGE_CURVE('',#1602,#1606,#555,.T.) ;
#1971=EDGE_CURVE('',#1598,#1605,#556,.T.) ;
#1972=EDGE_CURVE('',#1558,#1599,#103,.T.) ;
#1973=EDGE_CURVE('',#1604,#1559,#104,.T.) ;
#1974=EDGE_CURVE('',#1608,#1609,#557,.T.) ;
#1975=EDGE_CURVE('',#1608,#1550,#105,.T.) ;
#1976=EDGE_CURVE('',#1549,#1610,#106,.T.) ;
#1977=EDGE_CURVE('',#1611,#1610,#558,.T.) ;
#1978=EDGE_CURVE('',#1609,#1611,#1331,.T.) ;
#1979=EDGE_CURVE('',#1612,#1613,#107,.T.) ;
#1980=EDGE_CURVE('',#1613,#1608,#108,.T.) ;
#1981=EDGE_CURVE('',#1609,#1614,#109,.T.) ;
#1982=EDGE_CURVE('',#1614,#1615,#27,.T.) ;
#1983=EDGE_CURVE('',#1615,#1616,#17,.T.) ;
#1984=EDGE_CURVE('',#1616,#1617,#28,.T.) ;
#1985=EDGE_CURVE('',#1617,#1612,#110,.T.) ;
#1986=EDGE_CURVE('',#1610,#1618,#111,.T.) ;
#1987=EDGE_CURVE('',#1618,#1619,#112,.T.) ;
#1988=EDGE_CURVE('',#1619,#1620,#113,.T.) ;
#1989=EDGE_CURVE('',#1621,#1620,#18,.T.) ;
#1990=EDGE_CURVE('',#1621,#1611,#114,.T.) ;
#1991=EDGE_CURVE('',#1615,#1621,#559,.T.) ;
#1992=EDGE_CURVE('',#1616,#1620,#560,.T.) ;
#1993=EDGE_CURVE('',#1612,#1619,#561,.T.) ;
#1994=EDGE_CURVE('',#1546,#1613,#115,.T.) ;
#1995=EDGE_CURVE('',#1618,#1547,#116,.T.) ;
#1996=EDGE_CURVE('',#1622,#1623,#562,.T.) ;
#1997=EDGE_CURVE('',#1622,#1561,#117,.T.) ;
#1998=EDGE_CURVE('',#1565,#1624,#118,.T.) ;
#1999=EDGE_CURVE('',#1625,#1624,#563,.T.) ;
#2000=EDGE_CURVE('',#1623,#1625,#1332,.T.) ;
#2001=EDGE_CURVE('',#1626,#1627,#119,.T.) ;
#2002=EDGE_CURVE('',#1627,#1622,#120,.T.) ;
#2003=EDGE_CURVE('',#1623,#1628,#121,.T.) ;
#2004=EDGE_CURVE('',#1628,#1629,#29,.T.) ;
#2005=EDGE_CURVE('',#1629,#1630,#19,.T.) ;
#2006=EDGE_CURVE('',#1630,#1631,#30,.T.) ;
#2007=EDGE_CURVE('',#1631,#1626,#122,.T.) ;
#2008=EDGE_CURVE('',#1624,#1632,#123,.T.) ;
#2009=EDGE_CURVE('',#1632,#1633,#124,.T.) ;
#2010=EDGE_CURVE('',#1633,#1634,#125,.T.) ;
#2011=EDGE_CURVE('',#1635,#1634,#20,.T.) ;
#2012=EDGE_CURVE('',#1635,#1625,#126,.T.) ;
#2013=EDGE_CURVE('',#1629,#1635,#564,.T.) ;
#2014=EDGE_CURVE('',#1630,#1634,#565,.T.) ;
#2015=EDGE_CURVE('',#1626,#1633,#566,.T.) ;
#2016=EDGE_CURVE('',#1563,#1627,#127,.T.) ;
#2017=EDGE_CURVE('',#1632,#1564,#128,.T.) ;
#2437=ORIENTED_EDGE('',*,*,#1875,.F.) ;
#2438=ORIENTED_EDGE('',*,*,#1876,.T.) ;
#2439=ORIENTED_EDGE('',*,*,#1877,.T.) ;
#2440=ORIENTED_EDGE('',*,*,#1878,.F.) ;
#2441=ORIENTED_EDGE('',*,*,#1879,.T.) ;
#2442=ORIENTED_EDGE('',*,*,#1880,.T.) ;
#2443=ORIENTED_EDGE('',*,*,#1879,.F.) ;
#2444=ORIENTED_EDGE('',*,*,#1881,.F.) ;
#2445=ORIENTED_EDGE('',*,*,#1882,.T.) ;
#2446=ORIENTED_EDGE('',*,*,#1883,.T.) ;
#2447=ORIENTED_EDGE('',*,*,#1884,.T.) ;
#2448=ORIENTED_EDGE('',*,*,#1885,.T.) ;
#2449=ORIENTED_EDGE('',*,*,#1876,.F.) ;
#2450=ORIENTED_EDGE('',*,*,#1886,.T.) ;
#2451=ORIENTED_EDGE('',*,*,#1887,.T.) ;
#2452=ORIENTED_EDGE('',*,*,#1888,.T.) ;
#2453=ORIENTED_EDGE('',*,*,#1889,.T.) ;
#2454=ORIENTED_EDGE('',*,*,#1890,.T.) ;
#2455=ORIENTED_EDGE('',*,*,#1891,.F.) ;
#2456=ORIENTED_EDGE('',*,*,#1892,.T.) ;
#2457=ORIENTED_EDGE('',*,*,#1893,.T.) ;
#2458=ORIENTED_EDGE('',*,*,#1894,.T.) ;
#2459=ORIENTED_EDGE('',*,*,#1895,.T.) ;
#2460=ORIENTED_EDGE('',*,*,#1896,.T.) ;
#2461=ORIENTED_EDGE('',*,*,#1897,.F.) ;
#2462=ORIENTED_EDGE('',*,*,#1898,.T.) ;
#2463=ORIENTED_EDGE('',*,*,#1899,.T.) ;
#2464=ORIENTED_EDGE('',*,*,#1900,.T.) ;
#2465=ORIENTED_EDGE('',*,*,#1901,.T.) ;
#2466=ORIENTED_EDGE('',*,*,#1902,.F.) ;
#2467=ORIENTED_EDGE('',*,*,#1903,.T.) ;
#2468=ORIENTED_EDGE('',*,*,#1904,.T.) ;
#2469=ORIENTED_EDGE('',*,*,#1905,.T.) ;
#2470=ORIENTED_EDGE('',*,*,#1906,.T.) ;
#2471=ORIENTED_EDGE('',*,*,#1907,.F.) ;
#2472=ORIENTED_EDGE('',*,*,#1908,.F.) ;
#2473=ORIENTED_EDGE('',*,*,#1909,.T.) ;
#2474=ORIENTED_EDGE('',*,*,#1881,.T.) ;
#2475=ORIENTED_EDGE('',*,*,#1878,.T.) ;
#2476=ORIENTED_EDGE('',*,*,#1910,.T.) ;
#2477=ORIENTED_EDGE('',*,*,#1911,.F.) ;
#2478=ORIENTED_EDGE('',*,*,#1912,.F.) ;
#2479=ORIENTED_EDGE('',*,*,#1913,.T.) ;
#2480=ORIENTED_EDGE('',*,*,#1914,.T.) ;
#2481=ORIENTED_EDGE('',*,*,#1908,.T.) ;
#2482=ORIENTED_EDGE('',*,*,#1915,.T.) ;
#2483=ORIENTED_EDGE('',*,*,#1916,.T.) ;
#2484=ORIENTED_EDGE('',*,*,#1917,.T.) ;
#2485=ORIENTED_EDGE('',*,*,#1918,.T.) ;
#2486=ORIENTED_EDGE('',*,*,#1919,.T.) ;
#2487=ORIENTED_EDGE('',*,*,#1911,.T.) ;
#2488=ORIENTED_EDGE('',*,*,#1920,.T.) ;
#2489=ORIENTED_EDGE('',*,*,#1921,.T.) ;
#2490=ORIENTED_EDGE('',*,*,#1922,.T.) ;
#2491=ORIENTED_EDGE('',*,*,#1923,.F.) ;
#2492=ORIENTED_EDGE('',*,*,#1924,.T.) ;
#2493=ORIENTED_EDGE('',*,*,#1925,.F.) ;
#2494=ORIENTED_EDGE('',*,*,#1916,.F.) ;
#2495=ORIENTED_EDGE('',*,*,#1915,.F.) ;
#2496=ORIENTED_EDGE('',*,*,#1912,.T.) ;
#2497=ORIENTED_EDGE('',*,*,#1924,.F.) ;
#2498=ORIENTED_EDGE('',*,*,#1925,.T.) ;
#2499=ORIENTED_EDGE('',*,*,#1923,.T.) ;
#2500=ORIENTED_EDGE('',*,*,#1926,.F.) ;
#2501=ORIENTED_EDGE('',*,*,#1917,.F.) ;
#2502=ORIENTED_EDGE('',*,*,#1927,.F.) ;
#2503=ORIENTED_EDGE('',*,*,#1919,.F.) ;
#2504=ORIENTED_EDGE('',*,*,#1918,.F.) ;
#2505=ORIENTED_EDGE('',*,*,#1926,.T.) ;
#2506=ORIENTED_EDGE('',*,*,#1922,.F.) ;
#2507=ORIENTED_EDGE('',*,*,#1884,.F.) ;
#2508=ORIENTED_EDGE('',*,*,#1928,.T.) ;
#2509=ORIENTED_EDGE('',*,*,#1913,.F.) ;
#2510=ORIENTED_EDGE('',*,*,#1927,.T.) ;
#2511=ORIENTED_EDGE('',*,*,#1921,.F.) ;
#2512=ORIENTED_EDGE('',*,*,#1929,.T.) ;
#2513=ORIENTED_EDGE('',*,*,#1880,.F.) ;
#2514=ORIENTED_EDGE('',*,*,#1909,.F.) ;
#2515=ORIENTED_EDGE('',*,*,#1914,.F.) ;
#2516=ORIENTED_EDGE('',*,*,#1928,.F.) ;
#2517=ORIENTED_EDGE('',*,*,#1883,.F.) ;
#2518=ORIENTED_EDGE('',*,*,#1882,.F.) ;
#2519=ORIENTED_EDGE('',*,*,#1929,.F.) ;
#2520=ORIENTED_EDGE('',*,*,#1920,.F.) ;
#2521=ORIENTED_EDGE('',*,*,#1910,.F.) ;
#2522=ORIENTED_EDGE('',*,*,#1877,.F.) ;
#2523=ORIENTED_EDGE('',*,*,#1885,.F.) ;
#2524=ORIENTED_EDGE('',*,*,#1930,.F.) ;
#2525=ORIENTED_EDGE('',*,*,#1931,.T.) ;
#2526=ORIENTED_EDGE('',*,*,#1897,.T.) ;
#2527=ORIENTED_EDGE('',*,*,#1932,.T.) ;
#2528=ORIENTED_EDGE('',*,*,#1933,.F.) ;
#2529=ORIENTED_EDGE('',*,*,#1934,.F.) ;
#2530=ORIENTED_EDGE('',*,*,#1935,.T.) ;
#2531=ORIENTED_EDGE('',*,*,#1936,.T.) ;
#2532=ORIENTED_EDGE('',*,*,#1930,.T.) ;
#2533=ORIENTED_EDGE('',*,*,#1937,.T.) ;
#2534=ORIENTED_EDGE('',*,*,#1938,.T.) ;
#2535=ORIENTED_EDGE('',*,*,#1939,.T.) ;
#2536=ORIENTED_EDGE('',*,*,#1940,.T.) ;
#2537=ORIENTED_EDGE('',*,*,#1941,.T.) ;
#2538=ORIENTED_EDGE('',*,*,#1933,.T.) ;
#2539=ORIENTED_EDGE('',*,*,#1942,.T.) ;
#2540=ORIENTED_EDGE('',*,*,#1943,.T.) ;
#2541=ORIENTED_EDGE('',*,*,#1944,.T.) ;
#2542=ORIENTED_EDGE('',*,*,#1945,.F.) ;
#2543=ORIENTED_EDGE('',*,*,#1946,.T.) ;
#2544=ORIENTED_EDGE('',*,*,#1947,.F.) ;
#2545=ORIENTED_EDGE('',*,*,#1938,.F.) ;
#2546=ORIENTED_EDGE('',*,*,#1937,.F.) ;
#2547=ORIENTED_EDGE('',*,*,#1934,.T.) ;
#2548=ORIENTED_EDGE('',*,*,#1946,.F.) ;
#2549=ORIENTED_EDGE('',*,*,#1947,.T.) ;
#2550=ORIENTED_EDGE('',*,*,#1945,.T.) ;
#2551=ORIENTED_EDGE('',*,*,#1948,.F.) ;
#2552=ORIENTED_EDGE('',*,*,#1939,.F.) ;
#2553=ORIENTED_EDGE('',*,*,#1949,.F.) ;
#2554=ORIENTED_EDGE('',*,*,#1941,.F.) ;
#2555=ORIENTED_EDGE('',*,*,#1940,.F.) ;
#2556=ORIENTED_EDGE('',*,*,#1948,.T.) ;
#2557=ORIENTED_EDGE('',*,*,#1944,.F.) ;
#2558=ORIENTED_EDGE('',*,*,#1895,.F.) ;
#2559=ORIENTED_EDGE('',*,*,#1950,.T.) ;
#2560=ORIENTED_EDGE('',*,*,#1935,.F.) ;
#2561=ORIENTED_EDGE('',*,*,#1949,.T.) ;
#2562=ORIENTED_EDGE('',*,*,#1943,.F.) ;
#2563=ORIENTED_EDGE('',*,*,#1951,.T.) ;
#2564=ORIENTED_EDGE('',*,*,#1931,.F.) ;
#2565=ORIENTED_EDGE('',*,*,#1936,.F.) ;
#2566=ORIENTED_EDGE('',*,*,#1950,.F.) ;
#2567=ORIENTED_EDGE('',*,*,#1894,.F.) ;
#2568=ORIENTED_EDGE('',*,*,#1893,.F.) ;
#2569=ORIENTED_EDGE('',*,*,#1951,.F.) ;
#2570=ORIENTED_EDGE('',*,*,#1942,.F.) ;
#2571=ORIENTED_EDGE('',*,*,#1932,.F.) ;
#2572=ORIENTED_EDGE('',*,*,#1896,.F.) ;
#2573=ORIENTED_EDGE('',*,*,#1875,.T.) ;
#2574=ORIENTED_EDGE('',*,*,#1952,.F.) ;
#2575=ORIENTED_EDGE('',*,*,#1953,.T.) ;
#2576=ORIENTED_EDGE('',*,*,#1902,.T.) ;
#2577=ORIENTED_EDGE('',*,*,#1954,.T.) ;
#2578=ORIENTED_EDGE('',*,*,#1955,.F.) ;
#2579=ORIENTED_EDGE('',*,*,#1956,.F.) ;
#2580=ORIENTED_EDGE('',*,*,#1957,.T.) ;
#2581=ORIENTED_EDGE('',*,*,#1958,.T.) ;
#2582=ORIENTED_EDGE('',*,*,#1952,.T.) ;
#2583=ORIENTED_EDGE('',*,*,#1959,.T.) ;
#2584=ORIENTED_EDGE('',*,*,#1960,.T.) ;
#2585=ORIENTED_EDGE('',*,*,#1961,.T.) ;
#2586=ORIENTED_EDGE('',*,*,#1962,.T.) ;
#2587=ORIENTED_EDGE('',*,*,#1963,.T.) ;
#2588=ORIENTED_EDGE('',*,*,#1955,.T.) ;
#2589=ORIENTED_EDGE('',*,*,#1964,.T.) ;
#2590=ORIENTED_EDGE('',*,*,#1965,.T.) ;
#2591=ORIENTED_EDGE('',*,*,#1966,.T.) ;
#2592=ORIENTED_EDGE('',*,*,#1967,.F.) ;
#2593=ORIENTED_EDGE('',*,*,#1968,.T.) ;
#2594=ORIENTED_EDGE('',*,*,#1969,.F.) ;
#2595=ORIENTED_EDGE('',*,*,#1960,.F.) ;
#2596=ORIENTED_EDGE('',*,*,#1959,.F.) ;
#2597=ORIENTED_EDGE('',*,*,#1956,.T.) ;
#2598=ORIENTED_EDGE('',*,*,#1968,.F.) ;
#2599=ORIENTED_EDGE('',*,*,#1969,.T.) ;
#2600=ORIENTED_EDGE('',*,*,#1967,.T.) ;
#2601=ORIENTED_EDGE('',*,*,#1970,.F.) ;
#2602=ORIENTED_EDGE('',*,*,#1961,.F.) ;
#2603=ORIENTED_EDGE('',*,*,#1971,.F.) ;
#2604=ORIENTED_EDGE('',*,*,#1963,.F.) ;
#2605=ORIENTED_EDGE('',*,*,#1962,.F.) ;
#2606=ORIENTED_EDGE('',*,*,#1970,.T.) ;
#2607=ORIENTED_EDGE('',*,*,#1966,.F.) ;
#2608=ORIENTED_EDGE('',*,*,#1900,.F.) ;
#2609=ORIENTED_EDGE('',*,*,#1972,.T.) ;
#2610=ORIENTED_EDGE('',*,*,#1957,.F.) ;
#2611=ORIENTED_EDGE('',*,*,#1971,.T.) ;
#2612=ORIENTED_EDGE('',*,*,#1965,.F.) ;
#2613=ORIENTED_EDGE('',*,*,#1973,.T.) ;
#2614=ORIENTED_EDGE('',*,*,#1953,.F.) ;
#2615=ORIENTED_EDGE('',*,*,#1958,.F.) ;
#2616=ORIENTED_EDGE('',*,*,#1972,.F.) ;
#2617=ORIENTED_EDGE('',*,*,#1899,.F.) ;
#2618=ORIENTED_EDGE('',*,*,#1898,.F.) ;
#2619=ORIENTED_EDGE('',*,*,#1973,.F.) ;
#2620=ORIENTED_EDGE('',*,*,#1964,.F.) ;
#2621=ORIENTED_EDGE('',*,*,#1954,.F.) ;
#2622=ORIENTED_EDGE('',*,*,#1901,.F.) ;
#2623=ORIENTED_EDGE('',*,*,#1974,.F.) ;
#2624=ORIENTED_EDGE('',*,*,#1975,.T.) ;
#2625=ORIENTED_EDGE('',*,*,#1891,.T.) ;
#2626=ORIENTED_EDGE('',*,*,#1976,.T.) ;
#2627=ORIENTED_EDGE('',*,*,#1977,.F.) ;
#2628=ORIENTED_EDGE('',*,*,#1978,.F.) ;
#2629=ORIENTED_EDGE('',*,*,#1979,.T.) ;
#2630=ORIENTED_EDGE('',*,*,#1980,.T.) ;
#2631=ORIENTED_EDGE('',*,*,#1974,.T.) ;
#2632=ORIENTED_EDGE('',*,*,#1981,.T.) ;
#2633=ORIENTED_EDGE('',*,*,#1982,.T.) ;
#2634=ORIENTED_EDGE('',*,*,#1983,.T.) ;
#2635=ORIENTED_EDGE('',*,*,#1984,.T.) ;
#2636=ORIENTED_EDGE('',*,*,#1985,.T.) ;
#2637=ORIENTED_EDGE('',*,*,#1977,.T.) ;
#2638=ORIENTED_EDGE('',*,*,#1986,.T.) ;
#2639=ORIENTED_EDGE('',*,*,#1987,.T.) ;
#2640=ORIENTED_EDGE('',*,*,#1988,.T.) ;
#2641=ORIENTED_EDGE('',*,*,#1989,.F.) ;
#2642=ORIENTED_EDGE('',*,*,#1990,.T.) ;
#2643=ORIENTED_EDGE('',*,*,#1991,.F.) ;
#2644=ORIENTED_EDGE('',*,*,#1982,.F.) ;
#2645=ORIENTED_EDGE('',*,*,#1981,.F.) ;
#2646=ORIENTED_EDGE('',*,*,#1978,.T.) ;
#2647=ORIENTED_EDGE('',*,*,#1990,.F.) ;
#2648=ORIENTED_EDGE('',*,*,#1991,.T.) ;
#2649=ORIENTED_EDGE('',*,*,#1989,.T.) ;
#2650=ORIENTED_EDGE('',*,*,#1992,.F.) ;
#2651=ORIENTED_EDGE('',*,*,#1983,.F.) ;
#2652=ORIENTED_EDGE('',*,*,#1993,.F.) ;
#2653=ORIENTED_EDGE('',*,*,#1985,.F.) ;
#2654=ORIENTED_EDGE('',*,*,#1984,.F.) ;
#2655=ORIENTED_EDGE('',*,*,#1992,.T.) ;
#2656=ORIENTED_EDGE('',*,*,#1988,.F.) ;
#2657=ORIENTED_EDGE('',*,*,#1888,.F.) ;
#2658=ORIENTED_EDGE('',*,*,#1994,.T.) ;
#2659=ORIENTED_EDGE('',*,*,#1979,.F.) ;
#2660=ORIENTED_EDGE('',*,*,#1993,.T.) ;
#2661=ORIENTED_EDGE('',*,*,#1987,.F.) ;
#2662=ORIENTED_EDGE('',*,*,#1995,.T.) ;
#2663=ORIENTED_EDGE('',*,*,#1975,.F.) ;
#2664=ORIENTED_EDGE('',*,*,#1980,.F.) ;
#2665=ORIENTED_EDGE('',*,*,#1994,.F.) ;
#2666=ORIENTED_EDGE('',*,*,#1887,.F.) ;
#2667=ORIENTED_EDGE('',*,*,#1886,.F.) ;
#2668=ORIENTED_EDGE('',*,*,#1892,.F.) ;
#2669=ORIENTED_EDGE('',*,*,#1995,.F.) ;
#2670=ORIENTED_EDGE('',*,*,#1986,.F.) ;
#2671=ORIENTED_EDGE('',*,*,#1976,.F.) ;
#2672=ORIENTED_EDGE('',*,*,#1890,.F.) ;
#2673=ORIENTED_EDGE('',*,*,#1889,.F.) ;
#2674=ORIENTED_EDGE('',*,*,#1996,.F.) ;
#2675=ORIENTED_EDGE('',*,*,#1997,.T.) ;
#2676=ORIENTED_EDGE('',*,*,#1907,.T.) ;
#2677=ORIENTED_EDGE('',*,*,#1998,.T.) ;
#2678=ORIENTED_EDGE('',*,*,#1999,.F.) ;
#2679=ORIENTED_EDGE('',*,*,#2000,.F.) ;
#2680=ORIENTED_EDGE('',*,*,#2001,.T.) ;
#2681=ORIENTED_EDGE('',*,*,#2002,.T.) ;
#2682=ORIENTED_EDGE('',*,*,#1996,.T.) ;
#2683=ORIENTED_EDGE('',*,*,#2003,.T.) ;
#2684=ORIENTED_EDGE('',*,*,#2004,.T.) ;
#2685=ORIENTED_EDGE('',*,*,#2005,.T.) ;
#2686=ORIENTED_EDGE('',*,*,#2006,.T.) ;
#2687=ORIENTED_EDGE('',*,*,#2007,.T.) ;
#2688=ORIENTED_EDGE('',*,*,#1999,.T.) ;
#2689=ORIENTED_EDGE('',*,*,#2008,.T.) ;
#2690=ORIENTED_EDGE('',*,*,#2009,.T.) ;
#2691=ORIENTED_EDGE('',*,*,#2010,.T.) ;
#2692=ORIENTED_EDGE('',*,*,#2011,.F.) ;
#2693=ORIENTED_EDGE('',*,*,#2012,.T.) ;
#2694=ORIENTED_EDGE('',*,*,#2013,.F.) ;
#2695=ORIENTED_EDGE('',*,*,#2004,.F.) ;
#2696=ORIENTED_EDGE('',*,*,#2003,.F.) ;
#2697=ORIENTED_EDGE('',*,*,#2000,.T.) ;
#2698=ORIENTED_EDGE('',*,*,#2012,.F.) ;
#2699=ORIENTED_EDGE('',*,*,#2013,.T.) ;
#2700=ORIENTED_EDGE('',*,*,#2011,.T.) ;
#2701=ORIENTED_EDGE('',*,*,#2014,.F.) ;
#2702=ORIENTED_EDGE('',*,*,#2005,.F.) ;
#2703=ORIENTED_EDGE('',*,*,#2015,.F.) ;
#2704=ORIENTED_EDGE('',*,*,#2007,.F.) ;
#2705=ORIENTED_EDGE('',*,*,#2006,.F.) ;
#2706=ORIENTED_EDGE('',*,*,#2014,.T.) ;
#2707=ORIENTED_EDGE('',*,*,#2010,.F.) ;
#2708=ORIENTED_EDGE('',*,*,#1905,.F.) ;
#2709=ORIENTED_EDGE('',*,*,#2016,.T.) ;
#2710=ORIENTED_EDGE('',*,*,#2001,.F.) ;
#2711=ORIENTED_EDGE('',*,*,#2015,.T.) ;
#2712=ORIENTED_EDGE('',*,*,#2009,.F.) ;
#2713=ORIENTED_EDGE('',*,*,#2017,.T.) ;
#2714=ORIENTED_EDGE('',*,*,#1997,.F.) ;
#2715=ORIENTED_EDGE('',*,*,#2002,.F.) ;
#2716=ORIENTED_EDGE('',*,*,#2016,.F.) ;
#2717=ORIENTED_EDGE('',*,*,#1904,.F.) ;
#2718=ORIENTED_EDGE('',*,*,#1903,.F.) ;
#2719=ORIENTED_EDGE('',*,*,#2017,.F.) ;
#2720=ORIENTED_EDGE('',*,*,#2008,.F.) ;
#2721=ORIENTED_EDGE('',*,*,#1998,.F.) ;
#2722=ORIENTED_EDGE('',*,*,#1906,.F.) ;
#3389=ADVANCED_FACE('',(#881,#469,#470,#471,#472),#129,.T.) ;
#3390=ADVANCED_FACE('',(#882),#478,.F.) ;
#3391=ADVANCED_FACE('',(#883),#31,.T.) ;
#3392=ADVANCED_FACE('',(#884),#32,.T.) ;
#3393=ADVANCED_FACE('',(#885),#130,.T.) ;
#3394=ADVANCED_FACE('',(#886),#131,.T.) ;
#3395=ADVANCED_FACE('',(#887),#132,.T.) ;
#3396=ADVANCED_FACE('',(#888),#479,.T.) ;
#3397=ADVANCED_FACE('',(#889),#480,.F.) ;
#3398=ADVANCED_FACE('',(#890),#33,.F.) ;
#3399=ADVANCED_FACE('',(#891),#34,.F.) ;
#3400=ADVANCED_FACE('',(#892),#481,.F.) ;
#3401=ADVANCED_FACE('',(#893),#35,.T.) ;
#3402=ADVANCED_FACE('',(#894),#36,.T.) ;
#3403=ADVANCED_FACE('',(#895),#133,.T.) ;
#3404=ADVANCED_FACE('',(#896),#134,.T.) ;
#3405=ADVANCED_FACE('',(#897),#135,.T.) ;
#3406=ADVANCED_FACE('',(#898),#482,.T.) ;
#3407=ADVANCED_FACE('',(#899),#37,.F.) ;
#3408=ADVANCED_FACE('',(#900),#38,.F.) ;
#3409=ADVANCED_FACE('',(#901),#483,.T.) ;
#3410=ADVANCED_FACE('',(#902),#484,.F.) ;
#3411=ADVANCED_FACE('',(#903),#39,.T.) ;
#3412=ADVANCED_FACE('',(#904),#40,.T.) ;
#3413=ADVANCED_FACE('',(#905),#136,.T.) ;
#3414=ADVANCED_FACE('',(#906),#137,.T.) ;
#3415=ADVANCED_FACE('',(#907),#138,.T.) ;
#3416=ADVANCED_FACE('',(#908),#485,.T.) ;
#3417=ADVANCED_FACE('',(#909),#41,.F.) ;
#3418=ADVANCED_FACE('',(#910),#42,.F.) ;
#3419=ADVANCED_FACE('',(#911),#486,.F.) ;
#3420=ADVANCED_FACE('',(#912),#43,.T.) ;
#3421=ADVANCED_FACE('',(#913),#44,.T.) ;
#3422=ADVANCED_FACE('',(#914),#139,.T.) ;
#3423=ADVANCED_FACE('',(#915),#140,.T.) ;
#3424=ADVANCED_FACE('',(#916),#141,.T.) ;
#3425=ADVANCED_FACE('',(#917),#487,.T.) ;
#3426=ADVANCED_FACE('',(#918),#45,.F.) ;
#3427=ADVANCED_FACE('',(#919),#46,.F.) ;
#3428=ADVANCED_FACE('',(#920),#488,.F.) ;
#3429=ADVANCED_FACE('',(#921),#47,.T.) ;
#3430=ADVANCED_FACE('',(#922),#48,.T.) ;
#3431=ADVANCED_FACE('',(#923),#142,.T.) ;
#3432=ADVANCED_FACE('',(#924),#143,.T.) ;
#3433=ADVANCED_FACE('',(#925),#144,.T.) ;
#3434=ADVANCED_FACE('',(#926),#489,.T.) ;
#3435=ADVANCED_FACE('',(#927),#49,.F.) ;
#3436=ADVANCED_FACE('',(#928),#50,.F.) ;
#3582=CLOSED_SHELL('',(#3389,#3390,#3391,#3392,#3393,#3394,#3395,#3396,
#3397,#3398,#3399,#3400,#3401,#3402,#3403,#3404,#3405,#3406,#3407,#3408,
#3409,#3410,#3411,#3412,#3413,#3414,#3415,#3416,#3417,#3418,#3419,#3420,
#3421,#3422,#3423,#3424,#3425,#3426,#3427,#3428,#3429,#3430,#3431,#3432,
#3433,#3434,#3435,#3436)) ;
#4086=AXIS2_PLACEMENT_3D('',#5786,#4733,#4734) ;
#4087=AXIS2_PLACEMENT_3D('',#5787,#4735,#4736) ;
#4088=AXIS2_PLACEMENT_3D('',#5789,#4737,#4738) ;
#4089=AXIS2_PLACEMENT_3D('',#5798,#4740,#4741) ;
#4090=AXIS2_PLACEMENT_3D('',#5801,#4743,#4744) ;
#4091=AXIS2_PLACEMENT_3D('',#5803,#4745,#4746) ;
#4092=AXIS2_PLACEMENT_3D('',#6041,#4749,#4750) ;
#4093=AXIS2_PLACEMENT_3D('',#6209,#4752,#4753) ;
#4094=AXIS2_PLACEMENT_3D('',#6340,#4755,#4756) ;
#4095=AXIS2_PLACEMENT_3D('',#6470,#4758,#4759) ;
#4096=AXIS2_PLACEMENT_3D('',#6471,#4760,#4761) ;
#4097=AXIS2_PLACEMENT_3D('',#6502,#4764,#4765) ;
#4098=AXIS2_PLACEMENT_3D('',#6659,#4766,#4767) ;
#4099=AXIS2_PLACEMENT_3D('',#6677,#4768,#4769) ;
#4100=AXIS2_PLACEMENT_3D('',#6871,#4770,#4771) ;
#4101=AXIS2_PLACEMENT_3D('',#6873,#4773,#4774) ;
#4102=AXIS2_PLACEMENT_3D('',#6875,#4776,#4777) ;
#4103=AXIS2_PLACEMENT_3D('',#6877,#4779,#4780) ;
#4104=AXIS2_PLACEMENT_3D('',#6904,#4781,#4782) ;
#4105=AXIS2_PLACEMENT_3D('',#7109,#4783,#4784) ;
#4106=AXIS2_PLACEMENT_3D('',#7140,#4787,#4788) ;
#4107=AXIS2_PLACEMENT_3D('',#7297,#4789,#4790) ;
#4108=AXIS2_PLACEMENT_3D('',#7315,#4791,#4792) ;
#4109=AXIS2_PLACEMENT_3D('',#7509,#4793,#4794) ;
#4110=AXIS2_PLACEMENT_3D('',#7511,#4796,#4797) ;
#4111=AXIS2_PLACEMENT_3D('',#7513,#4799,#4800) ;
#4112=AXIS2_PLACEMENT_3D('',#7515,#4802,#4803) ;
#4113=AXIS2_PLACEMENT_3D('',#7746,#4804,#4805) ;
#4114=AXIS2_PLACEMENT_3D('',#7747,#4806,#4807) ;
#4115=AXIS2_PLACEMENT_3D('',#7778,#4810,#4811) ;
#4116=AXIS2_PLACEMENT_3D('',#7935,#4812,#4813) ;
#4117=AXIS2_PLACEMENT_3D('',#7953,#4814,#4815) ;
#4118=AXIS2_PLACEMENT_3D('',#8147,#4816,#4817) ;
#4119=AXIS2_PLACEMENT_3D('',#8149,#4819,#4820) ;
#4120=AXIS2_PLACEMENT_3D('',#8151,#4822,#4823) ;
#4121=AXIS2_PLACEMENT_3D('',#8153,#4825,#4826) ;
#4122=AXIS2_PLACEMENT_3D('',#8384,#4827,#4828) ;
#4123=AXIS2_PLACEMENT_3D('',#8415,#4831,#4832) ;
#4124=AXIS2_PLACEMENT_3D('',#8572,#4833,#4834) ;
#4125=AXIS2_PLACEMENT_3D('',#8590,#4835,#4836) ;
#4126=AXIS2_PLACEMENT_3D('',#8784,#4837,#4838) ;
#4127=AXIS2_PLACEMENT_3D('',#8786,#4840,#4841) ;
#4128=AXIS2_PLACEMENT_3D('',#8788,#4843,#4844) ;
#4129=AXIS2_PLACEMENT_3D('',#8790,#4846,#4847) ;
#4130=AXIS2_PLACEMENT_3D('',#9021,#4848,#4849) ;
#4131=AXIS2_PLACEMENT_3D('',#9052,#4852,#4853) ;
#4132=AXIS2_PLACEMENT_3D('',#9209,#4854,#4855) ;
#4133=AXIS2_PLACEMENT_3D('',#9227,#4856,#4857) ;
#4134=AXIS2_PLACEMENT_3D('',#9421,#4858,#4859) ;
#4135=AXIS2_PLACEMENT_3D('',#9423,#4861,#4862) ;
#4136=AXIS2_PLACEMENT_3D('',#9425,#4864,#4865) ;
#4137=AXIS2_PLACEMENT_3D('',#9427,#4867,#4868) ;
#4733=DIRECTION('axis',(0.,0.,1.)) ;
#4734=DIRECTION('refdir',(1.,0.,0.)) ;
#4735=DIRECTION('center_axis',(6.42891162084177E-17,1.,1.01883556321148E-16)) ;
#4736=DIRECTION('ref_axis',(-1.,6.42891162084177E-17,6.55000379205717E-33)) ;
#4737=DIRECTION('center_axis',(6.42891162084177E-17,1.,1.01883556321148E-16)) ;
#4738=DIRECTION('ref_axis',(-0.309016994374945,-7.70305906808054E-17,0.951056516295154)) ;
#4739=DIRECTION('',(-6.42891162084177E-17,-1.,-1.01883556321148E-16)) ;
#4740=DIRECTION('center_axis',(6.42891162084177E-17,1.,1.01883556321148E-16)) ;
#4741=DIRECTION('ref_axis',(-1.,6.42891162084177E-17,6.55000379205717E-33)) ;
#4742=DIRECTION('',(-6.42891162084177E-17,-1.,-1.01883556321148E-16)) ;
#4743=DIRECTION('center_axis',(6.42891162084177E-17,1.,1.01883556321148E-16)) ;
#4744=DIRECTION('ref_axis',(-1.,6.42891162084177E-17,6.55000379205717E-33)) ;
#4745=DIRECTION('center_axis',(6.42891162084177E-17,1.,1.01883556321148E-16)) ;
#4746=DIRECTION('ref_axis',(-1.,6.42891162084177E-17,6.55000379205717E-33)) ;
#4747=DIRECTION('',(6.42891162084177E-17,1.,1.01883556321148E-16)) ;
#4748=DIRECTION('',(6.42891162084177E-17,1.,1.01883556321148E-16)) ;
#4749=DIRECTION('center_axis',(6.42891162084177E-17,1.,1.01883556321148E-16)) ;
#4750=DIRECTION('ref_axis',(0.809016994374942,7.87466429072571E-18,-0.587785252292481)) ;
#4751=DIRECTION('',(6.42891162084177E-17,1.,1.01883556321148E-16)) ;
#4752=DIRECTION('center_axis',(6.42891162084177E-17,1.,1.01883556321148E-16)) ;
#4753=DIRECTION('ref_axis',(-0.309016994374945,-7.70305906808054E-17,0.951056516295154)) ;
#4754=DIRECTION('',(6.42891162084177E-17,1.,1.01883556321148E-16)) ;
#4755=DIRECTION('center_axis',(6.42891162084177E-17,1.,1.01883556321148E-16)) ;
#4756=DIRECTION('ref_axis',(0.809016994374951,-1.11896639422636E-16,0.587785252292469)) ;
#4757=DIRECTION('',(6.42891162084177E-17,1.,1.01883556321148E-16)) ;
#4758=DIRECTION('center_axis',(6.42891162084177E-17,1.,1.01883556321148E-16)) ;
#4759=DIRECTION('ref_axis',(-0.309016994374958,1.16763449604299E-16,-0.95105651629515)) ;
#4760=DIRECTION('center_axis',(6.42891162084176E-17,1.,1.01883556321148E-16)) ;
#4761=DIRECTION('ref_axis',(-1.,6.42891162084176E-17,-1.11022302462516E-16)) ;
#4762=DIRECTION('',(1.,0.,-1.38524120452482E-15)) ;
#4763=DIRECTION('',(-1.,0.,0.)) ;
#4764=DIRECTION('center_axis',(6.42891162084177E-17,1.,1.01883556321148E-16)) ;
#4765=DIRECTION('ref_axis',(-1.,6.42891162084177E-17,6.55000379205717E-33)) ;
#4766=DIRECTION('center_axis',(0.0914655886839077,0.93797861604457,-0.334410170194956)) ;
#4767=DIRECTION('ref_axis',(-0.225030533053291,0.346599923972543,0.910620531229106)) ;
#4768=DIRECTION('center_axis',(0.226649657308027,0.937972680585475,-0.262368411432195)) ;
#4769=DIRECTION('ref_axis',(-0.626757039824253,0.346652443702656,0.697859367140484)) ;
#4770=DIRECTION('center_axis',(6.42891162084177E-17,1.,1.01883556321148E-16)) ;
#4771=DIRECTION('ref_axis',(0.789438824149447,1.17867822247222E-17,-0.613829245739838)) ;
#4772=DIRECTION('',(6.42891162084177E-17,1.,1.01883556321148E-16)) ;
#4773=DIRECTION('center_axis',(6.42891162084177E-17,1.,1.01883556321148E-16)) ;
#4774=DIRECTION('ref_axis',(-1.,6.42891162084177E-17,6.55000379205717E-33)) ;
#4775=DIRECTION('',(6.42891162084177E-17,1.,1.01883556321148E-16)) ;
#4776=DIRECTION('center_axis',(6.42891162084177E-17,1.,1.01883556321148E-16)) ;
#4777=DIRECTION('ref_axis',(-1.,6.42891162084177E-17,6.55000379205717E-33)) ;
#4778=DIRECTION('',(6.42891162084177E-17,1.,1.01883556321148E-16)) ;
#4779=DIRECTION('center_axis',(-0.844327925302384,-3.10843368895129E-19,
0.535826795293564)) ;
#4780=DIRECTION('ref_axis',(0.535826795293564,-1.20470962841276E-16,0.844327925302384)) ;
#4781=DIRECTION('center_axis',(6.42891162084176E-17,1.,1.01883556321148E-16)) ;
#4782=DIRECTION('ref_axis',(-1.,6.42891162084176E-17,-1.11022302462516E-16)) ;
#4783=DIRECTION('center_axis',(6.42891162084177E-17,1.,1.01883556321148E-16)) ;
#4784=DIRECTION('ref_axis',(-0.309016994374945,-7.70305906808054E-17,0.951056516295155)) ;
#4785=DIRECTION('',(0.309016994374943,0.,-0.951056516295155)) ;
#4786=DIRECTION('',(-0.309016994374945,0.,0.951056516295155)) ;
#4787=DIRECTION('center_axis',(6.42891162084177E-17,1.,1.01883556321148E-16)) ;
#4788=DIRECTION('ref_axis',(-0.309016994374945,-7.70305906808054E-17,0.951056516295154)) ;
#4789=DIRECTION('center_axis',(-0.289778550198828,0.937978616044842,-0.190327369779724)) ;
#4790=DIRECTION('ref_axis',(0.795750585755454,0.346611107728181,0.496630391004513)) ;
#4791=DIRECTION('center_axis',(-0.179488590609232,0.937972680597995,-0.296632931908991)) ;
#4792=DIRECTION('ref_axis',(0.462146062282483,0.346581069349003,0.816273593524682)) ;
#4793=DIRECTION('center_axis',(6.42891162084177E-17,1.,1.01883556321148E-16)) ;
#4794=DIRECTION('ref_axis',(-0.339836291371861,1.1766769120353E-16,-0.94048460650168)) ;
#4795=DIRECTION('',(6.42891162084177E-17,1.,1.01883556321148E-16)) ;
#4796=DIRECTION('center_axis',(6.42891162084177E-17,1.,1.01883556321148E-16)) ;
#4797=DIRECTION('ref_axis',(-0.309016994374945,-7.70305906808053E-17,0.951056516295154)) ;
#4798=DIRECTION('',(6.42891162084177E-17,1.,1.01883556321148E-16)) ;
#4799=DIRECTION('center_axis',(6.42891162084177E-17,1.,1.01883556321148E-16)) ;
#4800=DIRECTION('ref_axis',(-0.309016994374945,-7.70305906808054E-17,0.951056516295154)) ;
#4801=DIRECTION('',(6.42891162084177E-17,1.,1.01883556321148E-16)) ;
#4802=DIRECTION('center_axis',(0.248689887525719,-1.14670750118124E-16,
0.968583161035977)) ;
#4803=DIRECTION('ref_axis',(0.968583161035977,-3.69319452351318E-17,-0.248689887525719)) ;
#4804=DIRECTION('center_axis',(6.42891162084176E-17,1.,1.01883556321148E-16)) ;
#4805=DIRECTION('ref_axis',(-1.,6.42891162084176E-17,-1.11022302462516E-16)) ;
#4806=DIRECTION('center_axis',(6.42891162084176E-17,1.,1.01883556321148E-16)) ;
#4807=DIRECTION('ref_axis',(0.809016994374951,-1.11896639422636E-16,0.587785252292469)) ;
#4808=DIRECTION('',(-0.809016994374952,3.46310301131204E-16,-0.587785252292467)) ;
#4809=DIRECTION('',(0.809016994374951,-3.67369352402517E-16,0.587785252292468)) ;
#4810=DIRECTION('center_axis',(6.42891162084177E-17,1.,1.01883556321148E-16)) ;
#4811=DIRECTION('ref_axis',(0.809016994374951,-1.11896639422636E-16,0.587785252292469)) ;
#4812=DIRECTION('center_axis',(-0.270558581956355,0.937978616044069,0.216781386594465)) ;
#4813=DIRECTION('ref_axis',(0.718062367667364,0.346609195532121,-0.603530033811504)) ;
#4814=DIRECTION('center_axis',(-0.337579707503438,0.937972680589643,0.0790391773070337)) ;
#4815=DIRECTION('ref_axis',(0.917158495892678,0.34665508108167,-0.196597426667139)) ;
#4816=DIRECTION('center_axis',(6.42891162084177E-17,1.,1.01883556321148E-16)) ;
#4817=DIRECTION('ref_axis',(-0.999469202827967,6.09358503167855E-17,0.0325777930257363)) ;
#4818=DIRECTION('',(6.42891162084177E-17,1.,1.01883556321148E-16)) ;
#4819=DIRECTION('center_axis',(6.42891162084177E-17,1.,1.01883556321148E-16)) ;
#4820=DIRECTION('ref_axis',(0.809016994374951,-1.11896639422636E-16,0.587785252292469)) ;
#4821=DIRECTION('',(6.42891162084177E-17,1.,1.01883556321148E-16)) ;
#4822=DIRECTION('center_axis',(6.42891162084177E-17,1.,1.01883556321148E-16)) ;
#4823=DIRECTION('ref_axis',(0.809016994374951,-1.11896639422636E-16,0.587785252292469)) ;
#4824=DIRECTION('',(6.42891162084177E-17,1.,1.01883556321148E-16)) ;
#4825=DIRECTION('center_axis',(0.998026728451666,-7.05595777195509E-17,
0.062790519157477)) ;
#4826=DIRECTION('ref_axis',(0.062790519157477,9.76457654153146E-17,-0.998026728451666)) ;
#4827=DIRECTION('center_axis',(6.42891162084176E-17,1.,1.01883556321148E-16)) ;
#4828=DIRECTION('ref_axis',(0.809016994374942,7.8746642907257E-18,-0.58778525229248)) ;
#4829=DIRECTION('',(-0.809016994374941,0.,0.587785252292482)) ;
#4830=DIRECTION('',(0.809016994374942,0.,-0.58778525229248)) ;
#4831=DIRECTION('center_axis',(6.42891162084177E-17,1.,1.01883556321148E-16)) ;
#4832=DIRECTION('ref_axis',(0.809016994374942,7.87466429072562E-18,-0.58778525229248)) ;
#4833=DIRECTION('center_axis',(0.122564151348405,0.937978616049674,0.324305634606899)) ;
#4834=DIRECTION('ref_axis',(0.352942571631502,-0.346602105458515,0.869079122762632)) ;
#4835=DIRECTION('center_axis',(-0.0291471407313505,0.937972680574302,0.345481829744264)) ;
#4836=DIRECTION('ref_axis',(-0.10087517992079,-0.346624346328332,0.932564078553536)) ;
#4837=DIRECTION('center_axis',(6.42891162084177E-17,1.,1.01883556321148E-16)) ;
#4838=DIRECTION('ref_axis',(-0.27786964668458,-8.00072645743807E-17,0.960618789870043)) ;
#4839=DIRECTION('',(6.42891162084177E-17,1.,1.01883556321148E-16)) ;
#4840=DIRECTION('center_axis',(6.42891162084177E-17,1.,1.01883556321148E-16)) ;
#4841=DIRECTION('ref_axis',(0.809016994374942,7.87466429072562E-18,-0.58778525229248)) ;
#4842=DIRECTION('',(6.42891162084177E-17,1.,1.01883556321148E-16)) ;
#4843=DIRECTION('center_axis',(6.42891162084177E-17,1.,1.01883556321148E-16)) ;
#4844=DIRECTION('ref_axis',(0.809016994374942,7.87466429072562E-18,-0.58778525229248)) ;
#4845=DIRECTION('',(6.42891162084177E-17,1.,1.01883556321148E-16)) ;
#4846=DIRECTION('center_axis',(0.368124552338267,7.10625328556022E-17,-0.929776486025405)) ;
#4847=DIRECTION('ref_axis',(-0.929776486025405,9.72803471192948E-17,-0.368124552338267)) ;
#4848=DIRECTION('center_axis',(6.42891162084177E-17,1.,1.01883556321148E-16)) ;
#4849=DIRECTION('ref_axis',(-0.309016994374958,1.16763449604299E-16,-0.95105651629515)) ;
#4850=DIRECTION('',(0.30901699437496,-3.46310301131204E-16,0.95105651629515)) ;
#4851=DIRECTION('',(-0.309016994374958,3.67369352402516E-16,-0.95105651629515)) ;
#4852=DIRECTION('center_axis',(6.42891162084177E-17,1.,1.01883556321148E-16)) ;
#4853=DIRECTION('ref_axis',(-0.309016994374958,1.16763449604299E-16,-0.95105651629515)) ;
#4854=DIRECTION('center_axis',(0.346307392767925,0.93797861604615,-0.016349481778672)) ;
#4855=DIRECTION('ref_axis',(0.935403580710108,-0.346577345830713,-0.0700305972532483)) ;
#4856=DIRECTION('center_axis',(0.319565783679362,0.937972680572322,0.134480334626918)) ;
#4857=DIRECTION('ref_axis',(0.856887437232556,-0.34664450139375,0.381551450746163)) ;
#4858=DIRECTION('center_axis',(6.42891162084177E-17,1.,1.01883556321148E-16)) ;
#4859=DIRECTION('ref_axis',(0.827736316734974,-1.10383059170658E-16,0.561117269345739)) ;
#4860=DIRECTION('',(6.42891162084177E-17,1.,1.01883556321148E-16)) ;
#4861=DIRECTION('center_axis',(6.42891162084177E-17,1.,1.01883556321148E-16)) ;
#4862=DIRECTION('ref_axis',(-0.309016994374958,1.16763449604299E-16,-0.95105651629515)) ;
#4863=DIRECTION('',(6.42891162084177E-17,1.,1.01883556321148E-16)) ;
#4864=DIRECTION('center_axis',(6.42891162084177E-17,1.,1.01883556321148E-16)) ;
#4865=DIRECTION('ref_axis',(-0.309016994374958,1.16763449604299E-16,-0.95105651629515)) ;
#4866=DIRECTION('',(6.42891162084177E-17,1.,1.01883556321148E-16)) ;
#4867=DIRECTION('center_axis',(-0.770513243013279,1.14478638350969E-16,
-0.637423989461614)) ;
#4868=DIRECTION('ref_axis',(-0.637423989461614,-3.75232044582032E-17,0.770513243013279)) ;
#5786=CARTESIAN_POINT('',(0.,0.,0.)) ;
#5787=CARTESIAN_POINT('Origin',(23.47768801576,43.8830586252741,68.2224337400009)) ;
#5788=CARTESIAN_POINT('',(31.07768801576,59.8830586252741,68.2224337400009)) ;
#5789=CARTESIAN_POINT('Origin',(23.47768801576,59.8830586252741,68.2224337400009)) ;
#5790=CARTESIAN_POINT('',(31.0776880612976,45.9361079682058,68.2224337399987)) ;
#5791=CARTESIAN_POINT('',(31.07768801576,43.8830586252741,68.2224337400009)) ;
#5792=CARTESIAN_POINT('',(31.0707352866625,45.3830586252742,67.8974209876918)) ;
#5793=CARTESIAN_POINT('Ctrl Pts',(31.07768801576,45.9361079682046,68.2224337400009)) ;
#5794=CARTESIAN_POINT('Ctrl Pts',(31.07768801576,45.7519411862255,68.1142267889447)) ;
#5795=CARTESIAN_POINT('Ctrl Pts',(31.0753771201502,45.5676059004178,68.0058651472121)) ;
#5796=CARTESIAN_POINT('Ctrl Pts',(31.070735276979,45.3830586252741,67.8974209881066)) ;
#5797=CARTESIAN_POINT('',(31.07768801576,45.3830586252741,68.2224337400009)) ;
#5798=CARTESIAN_POINT('Origin',(23.47768801576,45.3830586252741,68.2224337400009)) ;
#5799=CARTESIAN_POINT('',(31.07768801576,43.8830586252741,68.2224337400009)) ;
#5800=CARTESIAN_POINT('',(31.07768801576,43.8830586252741,68.2224337400009)) ;
#5801=CARTESIAN_POINT('Origin',(23.47768801576,43.8830586252741,68.2224337400009)) ;
#5802=CARTESIAN_POINT('',(31.0742800734864,45.3830634900505,68.4500118893126)) ;
#5803=CARTESIAN_POINT('Origin',(23.47768801576,45.3830586252741,68.2224337400009)) ;
#5804=CARTESIAN_POINT('',(27.6340951062153,57.8256696109516,74.5851579545834)) ;
#5805=CARTESIAN_POINT('Ctrl Pts',(31.0742801230022,45.3830652731003,68.4500124151661)) ;
#5806=CARTESIAN_POINT('Ctrl Pts',(31.0705756008784,45.5935267840764,68.5736831572555)) ;
#5807=CARTESIAN_POINT('Ctrl Pts',(31.0638548672636,45.8038922449875,68.6971313448079)) ;
#5808=CARTESIAN_POINT('Ctrl Pts',(31.0518691119314,46.0632318317031,68.8490202361335)) ;
#5809=CARTESIAN_POINT('Ctrl Pts',(31.0494392191971,46.1122612415161,68.8777284508602)) ;
#5810=CARTESIAN_POINT('Ctrl Pts',(31.0351342059633,46.3827042839367,69.0360189559014)) ;
#5811=CARTESIAN_POINT('Ctrl Pts',(31.020087358527,46.6040125923428,69.1653747748633)) ;
#5812=CARTESIAN_POINT('Ctrl Pts',(30.9986034331019,46.8632622432151,69.3162007814499)) ;
#5813=CARTESIAN_POINT('Ctrl Pts',(30.9953693582315,46.9011261856475,69.3382131230647)) ;
#5814=CARTESIAN_POINT('Ctrl Pts',(30.9715704181779,47.1717033808735,69.495396997657)) ;
#5815=CARTESIAN_POINT('Ctrl Pts',(30.9474582703363,47.4044689603727,69.6300128694532)) ;
#5816=CARTESIAN_POINT('Ctrl Pts',(30.9165145207437,47.663862891896,69.7793873192818)) ;
#5817=CARTESIAN_POINT('Ctrl Pts',(30.9132972664022,47.6904386808295,69.7946800230084)) ;
#5818=CARTESIAN_POINT('Ctrl Pts',(30.8800288137658,47.9612998636033,69.9504289150583)) ;
#5819=CARTESIAN_POINT('Ctrl Pts',(30.8460515474602,48.2057236046572,70.0899969837708)) ;
#5820=CARTESIAN_POINT('Ctrl Pts',(30.8058460215849,48.4649882125099,70.2369260769358)) ;
#5821=CARTESIAN_POINT('Ctrl Pts',(30.8034830172247,48.4801277704431,70.2455023164062)) ;
#5822=CARTESIAN_POINT('Ctrl Pts',(30.7609672635063,48.7507815722807,70.3987560508298)) ;
#5823=CARTESIAN_POINT('Ctrl Pts',(30.7165304066699,49.0060603871242,70.5422753814737)) ;
#5824=CARTESIAN_POINT('Ctrl Pts',(30.6672297149442,49.2650911286699,70.6862711816059)) ;
#5825=CARTESIAN_POINT('Ctrl Pts',(30.666520422233,49.268813158774,70.6883399479886)) ;
#5826=CARTESIAN_POINT('Ctrl Pts',(30.6163861031706,49.5315653220715,70.8343594519423)) ;
#5827=CARTESIAN_POINT('Ctrl Pts',(30.5626668547145,49.7905771610405,70.9767535845282)) ;
#5828=CARTESIAN_POINT('Ctrl Pts',(30.5029239276412,50.0572510953406,71.121757941137)) ;
#5829=CARTESIAN_POINT('Ctrl Pts',(30.5012000878133,50.0649289262866,71.1259313834614)) ;
#5830=CARTESIAN_POINT('Ctrl Pts',(30.4429225840978,50.3239244418443,71.2666667874793)) ;
#5831=CARTESIAN_POINT('Ctrl Pts',(30.3824337723248,50.57540159488,71.4014830392169)) ;
#5832=CARTESIAN_POINT('Ctrl Pts',(30.3131067557725,50.8461423400815,71.5446584556825)) ;
#5833=CARTESIAN_POINT('Ctrl Pts',(30.3081912119758,50.8652509230901,71.5547530784007)) ;
#5834=CARTESIAN_POINT('Ctrl Pts',(30.2411699989914,51.1245997230081,71.6916179346065)) ;
#5835=CARTESIAN_POINT('Ctrl Pts',(30.1754230730788,51.3650618940604,71.8169064463964)) ;
#5836=CARTESIAN_POINT('Ctrl Pts',(30.0975881230115,51.635843742555,71.9556952593753)) ;
#5837=CARTESIAN_POINT('Ctrl Pts',(30.088754982762,51.6663832990536,71.9713156300781)) ;
#5838=CARTESIAN_POINT('Ctrl Pts',(30.0010861726626,51.9676379850986,72.1250705521229)) ;
#5839=CARTESIAN_POINT('Ctrl Pts',(29.9180156669,52.238164456489,72.2606837295049)) ;
#5840=CARTESIAN_POINT('Ctrl Pts',(29.7606847862324,52.7256472364709,72.5003125758719)) ;
#5841=CARTESIAN_POINT('Ctrl Pts',(29.6880049010229,52.9427458528976,72.6051556822608)) ;
#5842=CARTESIAN_POINT('Ctrl Pts',(29.5942325442125,53.2131562545788,72.7334055575667)) ;
#5843=CARTESIAN_POINT('Ctrl Pts',(29.5755892637938,53.2664641483663,72.758575460154)) ;
#5844=CARTESIAN_POINT('Ctrl Pts',(29.484238140167,53.5254861983917,72.8803269249872)) ;
#5845=CARTESIAN_POINT('Ctrl Pts',(29.4093245268927,53.7311956119235,72.9753597322604)) ;
#5846=CARTESIAN_POINT('Ctrl Pts',(29.3079124503544,54.0017837515365,73.0978749780937)) ;
#5847=CARTESIAN_POINT('Ctrl Pts',(29.283425087555,54.0665473332678,73.1270096919038)) ;
#5848=CARTESIAN_POINT('Ctrl Pts',(29.1845494593619,54.3258257235604,73.242870772065)) ;
#5849=CARTESIAN_POINT('Ctrl Pts',(29.1083294283321,54.5205088505458,73.3282083519262)) ;
#5850=CARTESIAN_POINT('Ctrl Pts',(28.9995814541329,54.791419972509,73.4445685151767)) ;
#5851=CARTESIAN_POINT('Ctrl Pts',(28.9686820524854,54.8676682916987,73.4770501086411)) ;
#5852=CARTESIAN_POINT('Ctrl Pts',(28.8267551920768,55.2146576988594,73.6236213185704)) ;
#5853=CARTESIAN_POINT('Ctrl Pts',(28.7126177925182,55.4852678000175,73.7343097498549)) ;
#5854=CARTESIAN_POINT('Ctrl Pts',(28.5205593627065,55.9272948494755,73.9092265825147)) ;
#5855=CARTESIAN_POINT('Ctrl Pts',(28.4446562120935,56.0987899530306,73.9756393685776)) ;
#5856=CARTESIAN_POINT('Ctrl Pts',(28.3229756917417,56.3691923043808,74.0779062132529)) ;
#5857=CARTESIAN_POINT('Ctrl Pts',(28.2780539678421,56.4680781862301,74.1147900724143)) ;
#5858=CARTESIAN_POINT('Ctrl Pts',(28.0405709787764,56.9862401445908,74.3052598553338)) ;
#5859=CARTESIAN_POINT('Ctrl Pts',(27.8407773809973,57.405632674829,74.4501409788345)) ;
#5860=CARTESIAN_POINT('Ctrl Pts',(27.6341058620046,57.8256477521656,74.5851509282983)) ;
#5861=CARTESIAN_POINT('',(27.6340702364062,57.8265499696741,74.5851752834194)) ;
#5862=CARTESIAN_POINT('Ctrl Pts',(27.6340835637164,57.8256930685524,74.5851654947913)) ;
#5863=CARTESIAN_POINT('Ctrl Pts',(27.634069752068,57.8259720706221,74.5851745186134)) ;
#5864=CARTESIAN_POINT('Ctrl Pts',(27.6340698179607,57.8262610184418,74.5851746396025)) ;
#5865=CARTESIAN_POINT('Ctrl Pts',(27.6340699848282,57.826549969134,74.5851749064526)) ;
#5866=CARTESIAN_POINT('',(27.6340703658488,58.7660385728177,74.5851754951966)) ;
#5867=CARTESIAN_POINT('',(27.6340704790844,43.8830586252741,74.5851756661337)) ;
#5868=CARTESIAN_POINT('Ctrl Pts',(27.6340702509209,58.766038570856,74.5851753253735)) ;
#5869=CARTESIAN_POINT('Ctrl Pts',(27.7600299425795,58.5098890074295,74.5028909240232)) ;
#5870=CARTESIAN_POINT('Ctrl Pts',(27.8836766516442,58.253780180156,74.4167771302412)) ;
#5871=CARTESIAN_POINT('Ctrl Pts',(28.0101438591921,57.9857873917738,74.3229987438209)) ;
#5872=CARTESIAN_POINT('Ctrl Pts',(28.0157801192334,57.973831995724,74.318807191727)) ;
#5873=CARTESIAN_POINT('Ctrl Pts',(28.147615118801,57.6939113334552,74.2204803220524)) ;
#5874=CARTESIAN_POINT('Ctrl Pts',(28.2708796194584,57.426263839475,74.1224374801235)) ;
#5875=CARTESIAN_POINT('Ctrl Pts',(28.3922280683633,57.1556222836718,74.0196140263438)) ;
#5876=CARTESIAN_POINT('Ctrl Pts',(28.3935945166274,57.1525737751886,74.0184553483433)) ;
#5877=CARTESIAN_POINT('Ctrl Pts',(28.5215787684715,56.8669561800162,73.9098533842011)) ;
#5878=CARTESIAN_POINT('Ctrl Pts',(28.644551100692,56.5844497694098,73.7983737701696)) ;
#5879=CARTESIAN_POINT('Ctrl Pts',(28.8692587681259,56.0525625568707,73.5808364497842)) ;
#5880=CARTESIAN_POINT('Ctrl Pts',(28.9716456686909,55.8030380923874,73.4758091882058)) ;
#5881=CARTESIAN_POINT('Ctrl Pts',(29.0840928441225,55.5203596436975,73.3535741415821)) ;
#5882=CARTESIAN_POINT('Ctrl Pts',(29.0971736066216,55.487339023581,73.3392450682227)) ;
#5883=CARTESIAN_POINT('Ctrl Pts',(29.202780837364,55.2196257773339,73.2226665271722)) ;
#5884=CARTESIAN_POINT('Ctrl Pts',(29.2927320594827,54.9847737061719,73.1177666619654)) ;
#5885=CARTESIAN_POINT('Ctrl Pts',(29.3975387478343,54.7017289710564,72.9885809457978)) ;
#5886=CARTESIAN_POINT('Ctrl Pts',(29.4152135223729,54.6536565138857,72.9665446527025)) ;
#5887=CARTESIAN_POINT('Ctrl Pts',(29.5130363251233,54.3856593021878,72.8431766243648)) ;
#5888=CARTESIAN_POINT('Ctrl Pts',(29.5906542386682,54.1659530442002,72.7399905215469)) ;
#5889=CARTESIAN_POINT('Ctrl Pts',(29.6871182370823,53.8833573751818,72.6047103924036)) ;
#5890=CARTESIAN_POINT('Ctrl Pts',(29.7083973107427,53.8203770818542,72.5744025927511)) ;
#5891=CARTESIAN_POINT('Ctrl Pts',(29.7978525182514,53.5528374916877,72.4449910678865)) ;
#5892=CARTESIAN_POINT('Ctrl Pts',(29.8638327717365,53.348275131605,72.3445230657125)) ;
#5893=CARTESIAN_POINT('Ctrl Pts',(29.9516247240262,53.0657839416432,72.2036705749113)) ;
#5894=CARTESIAN_POINT('Ctrl Pts',(29.9754972013003,52.9878441570689,72.1645872031147)) ;
#5895=CARTESIAN_POINT('Ctrl Pts',(30.0562338081894,52.7203373164194,72.029683143324)) ;
#5896=CARTESIAN_POINT('Ctrl Pts',(30.1113680689016,52.5307715920929,71.932783916218)) ;
#5897=CARTESIAN_POINT('Ctrl Pts',(30.1903188679312,52.2481729096978,71.7866399275519)) ;
#5898=CARTESIAN_POINT('Ctrl Pts',(30.2157706265884,52.1552026240065,71.7382875582465)) ;
#5899=CARTESIAN_POINT('Ctrl Pts',(30.2785909073748,51.9208262076072,71.6157534900977)) ;
#5900=CARTESIAN_POINT('Ctrl Pts',(30.3152863743369,51.7794006203881,71.5411932918103)) ;
#5901=CARTESIAN_POINT('Ctrl Pts',(30.3591587242532,51.60452330737,71.448227653069)) ;
#5902=CARTESIAN_POINT('Ctrl Pts',(30.3674716743981,51.5711185095033,71.4304337880207)) ;
#5903=CARTESIAN_POINT('Ctrl Pts',(30.4023942104701,51.4296212255096,71.3549201756335)) ;
#5904=CARTESIAN_POINT('Ctrl Pts',(30.4283592597888,51.3215155544796,71.2968765915474)) ;
#5905=CARTESIAN_POINT('Ctrl Pts',(30.4908183940924,51.0537368175205,71.152420071463)) ;
#5906=CARTESIAN_POINT('Ctrl Pts',(30.5264364258323,50.8941113379638,71.0656618252809)) ;
#5907=CARTESIAN_POINT('Ctrl Pts',(30.5865621606833,50.6118990016945,70.9111362808276)) ;
#5908=CARTESIAN_POINT('Ctrl Pts',(30.6117380024369,50.4892574041004,70.8436019858225)) ;
#5909=CARTESIAN_POINT('Ctrl Pts',(30.6644649877661,50.2223202255289,70.6957801754687)) ;
#5910=CARTESIAN_POINT('Ctrl Pts',(30.6916211845518,50.0780242815205,70.6154142118301)) ;
#5911=CARTESIAN_POINT('Ctrl Pts',(30.7419452106475,49.7965776405067,70.4578470852657)) ;
#5912=CARTESIAN_POINT('Ctrl Pts',(30.7652403570727,49.6594152246682,70.3806899793754)) ;
#5913=CARTESIAN_POINT('Ctrl Pts',(30.8081006160294,49.3929482765754,70.2301253928115)) ;
#5914=CARTESIAN_POINT('Ctrl Pts',(30.8278110118762,49.2636615036751,70.1567171260021)) ;
#5915=CARTESIAN_POINT('Ctrl Pts',(30.8682544166326,48.9827045772249,69.9965436405729)) ;
#5916=CARTESIAN_POINT('Ctrl Pts',(30.8885647864592,48.8310367404956,69.9096944982135)) ;
#5917=CARTESIAN_POINT('Ctrl Pts',(30.9214998312479,48.5648138959559,69.7567724669571)) ;
#5918=CARTESIAN_POINT('Ctrl Pts',(30.9347940974624,48.4502757510319,69.6908019636932)) ;
#5919=CARTESIAN_POINT('Ctrl Pts',(30.9652388398132,48.169433296079,69.528627660098)) ;
#5920=CARTESIAN_POINT('Ctrl Pts',(30.9814192229612,48.0031363324805,69.4322203252873)) ;
#5921=CARTESIAN_POINT('Ctrl Pts',(31.0043480443608,47.7369180822766,69.2773466723917)) ;
#5922=CARTESIAN_POINT('Ctrl Pts',(31.0122778434617,47.6369794599077,69.2191365361054)) ;
#5923=CARTESIAN_POINT('Ctrl Pts',(31.032663409965,47.3560315968962,69.0553072016704)) ;
#5924=CARTESIAN_POINT('Ctrl Pts',(31.0435800890746,47.1749633576186,68.9494892744708)) ;
#5925=CARTESIAN_POINT('Ctrl Pts',(31.0657783101076,46.7126338479033,68.6787096511655)) ;
#5926=CARTESIAN_POINT('Ctrl Pts',(31.0739241994752,46.4312682182311,68.513324772655)) ;
#5927=CARTESIAN_POINT('Ctrl Pts',(31.0773432634457,46.0783306369255,68.3060020525323)) ;
#5928=CARTESIAN_POINT('Ctrl Pts',(31.0776880663112,46.0072326116127,68.2642279969038)) ;
#5929=CARTESIAN_POINT('Ctrl Pts',(31.0776881068351,45.9361079682071,68.2224337399966)) ;
#5930=CARTESIAN_POINT('',(15.8776875119243,53.1208403600521,68.2224337443077)) ;
#5931=CARTESIAN_POINT('',(16.3751686437571,57.8256698856438,65.5179563592932)) ;
#5932=CARTESIAN_POINT('Ctrl Pts',(15.8776875119243,53.1208403600521,68.2224337443077)) ;
#5933=CARTESIAN_POINT('Ctrl Pts',(15.8776877387063,53.1871490007968,68.1834760773303)) ;
#5934=CARTESIAN_POINT('Ctrl Pts',(15.8779875469879,53.2534600732653,68.1445152562114)) ;
#5935=CARTESIAN_POINT('Ctrl Pts',(15.8810308727502,53.5902066966755,67.946652756444)) ;
#5936=CARTESIAN_POINT('Ctrl Pts',(15.888467388127,53.860642481361,67.7876705864655)) ;
#5937=CARTESIAN_POINT('Ctrl Pts',(15.9034088077128,54.1864226824151,67.5968601517276)) ;
#5938=CARTESIAN_POINT('Ctrl Pts',(15.9061431888012,54.2415348490089,67.5645950586243)) ;
#5939=CARTESIAN_POINT('Ctrl Pts',(15.9195506920211,54.4928052763559,67.4175674694017)) ;
#5940=CARTESIAN_POINT('Ctrl Pts',(15.9326424619461,54.6891498815712,67.3028817310846)) ;
#5941=CARTESIAN_POINT('Ctrl Pts',(15.9498927681818,54.9048361953365,67.1772400978473)) ;
#5942=CARTESIAN_POINT('Ctrl Pts',(15.9514802349652,54.9243619105753,67.1658693825961)) ;
#5943=CARTESIAN_POINT('Ctrl Pts',(15.9676855587794,55.1204950653914,67.0516873615927)) ;
#5944=CARTESIAN_POINT('Ctrl Pts',(15.9843658342187,55.2970548144963,66.9492903649222)) ;
#5945=CARTESIAN_POINT('Ctrl Pts',(16.0131302290761,55.5676362557331,66.7929442727957)) ;
#5946=CARTESIAN_POINT('Ctrl Pts',(16.0237231107349,55.6616980715273,66.738701338355)) ;
#5947=CARTESIAN_POINT('Ctrl Pts',(16.0670697461354,56.0262039248394,66.5289163363484)) ;
#5948=CARTESIAN_POINT('Ctrl Pts',(16.1041291773361,56.2965161322938,66.3742241105852)) ;
#5949=CARTESIAN_POINT('Ctrl Pts',(16.2108439844322,56.9862189711356,65.9833159733028)) ;
#5950=CARTESIAN_POINT('Ctrl Pts',(16.2873230212551,57.4056466389749,65.7486646609522)) ;
#5951=CARTESIAN_POINT('Ctrl Pts',(16.3751640146366,57.8256477521648,65.5179685166535)) ;
#5952=CARTESIAN_POINT('',(16.3751780994845,57.8271591849708,65.5179277057667)) ;
#5953=CARTESIAN_POINT('Ctrl Pts',(16.3751735099526,57.8256931526636,65.5179435793076)) ;
#5954=CARTESIAN_POINT('Ctrl Pts',(16.375179360142,57.8261752208488,65.5179282095724)) ;
#5955=CARTESIAN_POINT('Ctrl Pts',(16.3751789637411,57.8266672012913,65.5179280439107)) ;
#5956=CARTESIAN_POINT('Ctrl Pts',(16.3751780994845,57.8271591849708,65.5179277057666)) ;
#5957=CARTESIAN_POINT('',(16.3751775163941,58.7660404020332,65.5179292370655)) ;
#5958=CARTESIAN_POINT('',(16.3751780994845,43.8830586252741,65.5179277057667)) ;
#5959=CARTESIAN_POINT('',(15.87768801576,54.0610773150226,68.2224337400137)) ;
#5960=CARTESIAN_POINT('Ctrl Pts',(16.3751775163941,58.7660404020332,65.5179292370655)) ;
#5961=CARTESIAN_POINT('Ctrl Pts',(16.318048692533,58.4927517118959,65.6679597032189)) ;
#5962=CARTESIAN_POINT('Ctrl Pts',(16.2656591635554,58.2194425159302,65.8198505460739)) ;
#5963=CARTESIAN_POINT('Ctrl Pts',(16.1974167526078,57.8271113937991,66.0401048199781)) ;
#5964=CARTESIAN_POINT('Ctrl Pts',(16.1776103066955,57.7079337985678,66.1073050755783)) ;
#5965=CARTESIAN_POINT('Ctrl Pts',(16.1031323071922,57.2377082464182,66.3735075476004)) ;
#5966=CARTESIAN_POINT('Ctrl Pts',(16.0556887898407,56.8868665748457,66.574271919069)) ;
#5967=CARTESIAN_POINT('Ctrl Pts',(16.0118950098979,56.495184630307,66.8002830769449)) ;
#5968=CARTESIAN_POINT('Ctrl Pts',(16.0074344951922,56.4542916276441,66.8239023131688)) ;
#5969=CARTESIAN_POINT('Ctrl Pts',(15.9614349400052,56.0217278514861,67.0739792638625)) ;
#5970=CARTESIAN_POINT('Ctrl Pts',(15.9300813885958,55.6299821269397,67.3022360334898)) ;
#5971=CARTESIAN_POINT('Ctrl Pts',(15.8992014526108,55.05188349398,67.6406353482144)) ;
#5972=CARTESIAN_POINT('Ctrl Pts',(15.8916062131826,54.8657705646704,67.7498652264096)) ;
#5973=CARTESIAN_POINT('Ctrl Pts',(15.8860940383579,54.6695659260189,67.865031687881)) ;
#5974=CARTESIAN_POINT('Ctrl Pts',(15.8858167980585,54.6594490920002,67.8709700152553)) ;
#5975=CARTESIAN_POINT('Ctrl Pts',(15.8803052730986,54.4531311678522,67.9920733247475)) ;
#5976=CARTESIAN_POINT('Ctrl Pts',(15.8776880157599,54.2570462500708,68.1072484844461)) ;
#5977=CARTESIAN_POINT('Ctrl Pts',(15.87768801576,54.0610773150155,68.2224337400016)) ;
#5978=CARTESIAN_POINT('',(17.5258214371218,45.3830586252742,72.9484557858036)) ;
#5979=CARTESIAN_POINT('Ctrl Pts',(15.87768801576,54.0610773150297,68.2224337400258)) ;
#5980=CARTESIAN_POINT('Ctrl Pts',(15.8776880157602,53.9598262897505,68.2819463623541)) ;
#5981=CARTESIAN_POINT('Ctrl Pts',(15.8783870294523,53.8586011420046,68.3414526422372)) ;
#5982=CARTESIAN_POINT('Ctrl Pts',(15.8797847080111,53.7573959543402,68.4009423563146)) ;
#5983=CARTESIAN_POINT('Ctrl Pts',(15.8834278383639,53.4935987538091,68.5560057517411)) ;
#5984=CARTESIAN_POINT('Ctrl Pts',(15.8918090487111,53.2298184766074,68.7107644985098)) ;
#5985=CARTESIAN_POINT('Ctrl Pts',(15.9049188360724,52.966059183431,68.8652143800119)) ;
#5986=CARTESIAN_POINT('Ctrl Pts',(15.9058492786295,52.947339362548,68.8761761705229)) ;
#5987=CARTESIAN_POINT('Ctrl Pts',(15.9068035616431,52.9286196473653,68.8871364041267)) ;
#5988=CARTESIAN_POINT('Ctrl Pts',(15.9077816916672,52.9099000393348,68.8980950785868)) ;
#5989=CARTESIAN_POINT('Ctrl Pts',(15.922541707333,52.6274205110582,69.063461852667)) ;
#5990=CARTESIAN_POINT('Ctrl Pts',(15.9427340901668,52.3449496227476,69.2284477477508)) ;
#5991=CARTESIAN_POINT('Ctrl Pts',(15.9683106417657,52.0622051908031,69.3925839247815)) ;
#5992=CARTESIAN_POINT('Ctrl Pts',(15.9735819620023,52.0039316412923,69.4264123456382)) ;
#5993=CARTESIAN_POINT('Ctrl Pts',(15.9790825849275,51.9456496648422,69.4602098098499)) ;
#5994=CARTESIAN_POINT('Ctrl Pts',(15.984812754553,51.8873592927888,69.4939762363384)) ;
#5995=CARTESIAN_POINT('Ctrl Pts',(15.992984279923,51.8042341350373,69.542128948865)) ;
#5996=CARTESIAN_POINT('Ctrl Pts',(16.0016230688955,51.7210878853372,69.590221238424)) ;
#5997=CARTESIAN_POINT('Ctrl Pts',(16.0107299125882,51.6379247117809,69.6382503543534)) ;
#5998=CARTESIAN_POINT('Ctrl Pts',(16.0214869739339,51.5396918453961,69.6949826497423)) ;
#5999=CARTESIAN_POINT('Ctrl Pts',(16.0329010704352,51.4414217778531,69.7516433072497)) ;
#6000=CARTESIAN_POINT('Ctrl Pts',(16.0449492807277,51.3432074537042,69.8081181022716)) ;
#6001=CARTESIAN_POINT('Ctrl Pts',(16.0502540143438,51.2999644479586,69.8329835168309)) ;
#6002=CARTESIAN_POINT('Ctrl Pts',(16.0556820779081,51.2567285488362,69.8578153874229)) ;
#6003=CARTESIAN_POINT('Ctrl Pts',(16.061231033401,51.2135073972261,69.8826041616199)) ;
#6004=CARTESIAN_POINT('Ctrl Pts',(16.0789544785872,51.0754584054067,69.9617798697825)) ;
#6005=CARTESIAN_POINT('Ctrl Pts',(16.0979255370188,50.9375082770569,70.0405823222603)) ;
#6006=CARTESIAN_POINT('Ctrl Pts',(16.1181351551565,50.7996661916347,70.1190047753123)) ;
#6007=CARTESIAN_POINT('Ctrl Pts',(16.1393118540383,50.6552280178723,70.2011799387692)) ;
#6008=CARTESIAN_POINT('Ctrl Pts',(16.1618492668502,50.5109057227833,70.2829413721308)) ;
#6009=CARTESIAN_POINT('Ctrl Pts',(16.1857433083364,50.3666994632668,70.3642886332832)) ;
#6010=CARTESIAN_POINT('Ctrl Pts',(16.2217335002578,50.1494900406054,70.4868172370292)) ;
#6011=CARTESIAN_POINT('Ctrl Pts',(16.2607672253128,49.9324691220747,70.6082868352782)) ;
#6012=CARTESIAN_POINT('Ctrl Pts',(16.3027912912963,49.715573436112,70.7285975401703)) ;
#6013=CARTESIAN_POINT('Ctrl Pts',(16.3152762507575,49.65113574349,70.7643407325098)) ;
#6014=CARTESIAN_POINT('Ctrl Pts',(16.3280255475019,49.5867095881029,70.7999827452736)) ;
#6015=CARTESIAN_POINT('Ctrl Pts',(16.3410378746391,49.5222932712664,70.8355209492688)) ;
#6016=CARTESIAN_POINT('Ctrl Pts',(16.3926299094743,49.2668916949656,70.9764248966691)) ;
#6017=CARTESIAN_POINT('Ctrl Pts',(16.4484105732616,49.0117332177746,71.1158311082438)) ;
#6018=CARTESIAN_POINT('Ctrl Pts',(16.5082176847315,48.7565688872915,71.2533549374115)) ;
#6019=CARTESIAN_POINT('Ctrl Pts',(16.5142510416214,48.730827843567,71.2672283769047)) ;
#6020=CARTESIAN_POINT('Ctrl Pts',(16.5203253348275,48.7050867402745,71.2810826771504)) ;
#6021=CARTESIAN_POINT('Ctrl Pts',(16.5264403710249,48.6793453218294,71.2949174554279)) ;
#6022=CARTESIAN_POINT('Ctrl Pts',(16.5931574897773,48.3984977167074,71.445859578331)) ;
#6023=CARTESIAN_POINT('Ctrl Pts',(16.6647653754236,48.1176791006564,71.5945788691957)) ;
#6024=CARTESIAN_POINT('Ctrl Pts',(16.7412285650833,47.8368320972583,71.7409723669579)) ;
#6025=CARTESIAN_POINT('Ctrl Pts',(16.7670315043542,47.7420586748396,71.7903736873739)) ;
#6026=CARTESIAN_POINT('Ctrl Pts',(16.7933718109271,47.6472611060918,71.8394797343875)) ;
#6027=CARTESIAN_POINT('Ctrl Pts',(16.820248904836,47.5524394572103,71.8882903226211)) ;
#6028=CARTESIAN_POINT('Ctrl Pts',(16.8730041029354,47.366320567728,71.9840972673871)) ;
#6029=CARTESIAN_POINT('Ctrl Pts',(16.9278282648647,47.1801103309901,72.078769184525)) ;
#6030=CARTESIAN_POINT('Ctrl Pts',(16.9847270270042,46.9938102819949,72.1723017882395)) ;
#6031=CARTESIAN_POINT('Ctrl Pts',(17.0380761434748,46.8191326152305,72.2599993335239)) ;
#6032=CARTESIAN_POINT('Ctrl Pts',(17.0932559186719,46.6443819715505,72.346703095831)) ;
#6033=CARTESIAN_POINT('Ctrl Pts',(17.1502082429138,46.4694842601059,72.4323030638899)) ;
#6034=CARTESIAN_POINT('Ctrl Pts',(17.1849311118386,46.3628520832706,72.4844919167672)) ;
#6035=CARTESIAN_POINT('Ctrl Pts',(17.220311010757,46.2561640031219,72.5362680765448)) ;
#6036=CARTESIAN_POINT('Ctrl Pts',(17.2563345933752,46.1494043647081,72.5876097494857)) ;
#6037=CARTESIAN_POINT('Ctrl Pts',(17.3424138503274,45.8942995228455,72.7102919686384)) ;
#6038=CARTESIAN_POINT('Ctrl Pts',(17.4322561663653,45.6388798336617,72.8306213626458)) ;
#6039=CARTESIAN_POINT('Ctrl Pts',(17.5258214447123,45.3830586252743,72.9484557797765)) ;
#6040=CARTESIAN_POINT('',(17.1981488755629,45.3830634197606,72.5034839444725)) ;
#6041=CARTESIAN_POINT('Origin',(23.47768801576,45.3830586252741,68.2224337400009)) ;
#6042=CARTESIAN_POINT('Ctrl Pts',(17.1981485126538,45.3830652730852,72.5034835325328)) ;
#6043=CARTESIAN_POINT('Ctrl Pts',(17.1284537177608,45.5935267173151,72.4012543694107)) ;
#6044=CARTESIAN_POINT('Ctrl Pts',(17.0613339404697,45.8038970071019,72.2974387949214)) ;
#6045=CARTESIAN_POINT('Ctrl Pts',(16.962354850366,46.1264421086301,72.1358443111681)) ;
#6046=CARTESIAN_POINT('Ctrl Pts',(16.9286362979452,46.2386508709495,72.0791500238972)) ;
#6047=CARTESIAN_POINT('Ctrl Pts',(16.8491643584742,46.5090378891581,71.9414799227803)) ;
#6048=CARTESIAN_POINT('Ctrl Pts',(16.8041447292678,46.6672026152944,71.8600789986582)) ;
#6049=CARTESIAN_POINT('Ctrl Pts',(16.7155010485011,46.9896373648865,71.6926127002568)) ;
#6050=CARTESIAN_POINT('Ctrl Pts',(16.671982425607,47.1538972164843,71.606471066007)) ;
#6051=CARTESIAN_POINT('Ctrl Pts',(16.602990660836,47.4245379703279,71.4631823632395)) ;
#6052=CARTESIAN_POINT('Ctrl Pts',(16.5765640699983,47.5309048058355,71.4065194705275)) ;
#6053=CARTESIAN_POINT('Ctrl Pts',(16.4984989659946,47.8535340062433,71.2335950304104)) ;
#6054=CARTESIAN_POINT('Ctrl Pts',(16.4490923792239,48.069949799947,71.1163855119266)) ;
#6055=CARTESIAN_POINT('Ctrl Pts',(16.3909875905432,48.3407265621182,70.9682854354735)) ;
#6056=CARTESIAN_POINT('Ctrl Pts',(16.3794669871731,48.3952944415037,70.93836556585)) ;
#6057=CARTESIAN_POINT('Ctrl Pts',(16.3125132413207,48.7177229150411,70.7611427633822)) ;
#6058=CARTESIAN_POINT('Ctrl Pts',(16.261446163163,48.9853758417281,70.6121169893423)) ;
#6059=CARTESIAN_POINT('Ctrl Pts',(16.2146236633515,49.2558099187254,70.4602672618887)) ;
#6060=CARTESIAN_POINT('Ctrl Pts',(16.214142876459,49.2585897556055,70.4587062362067)) ;
#6061=CARTESIAN_POINT('Ctrl Pts',(16.2136625986088,49.2613695957061,70.4571450723729)) ;
#6062=CARTESIAN_POINT('Ctrl Pts',(16.1669395803816,49.5318016375275,70.3052698896535)) ;
#6063=CARTESIAN_POINT('Ctrl Pts',(16.1249977580323,49.8022075449293,70.1520021909819)) ;
#6064=CARTESIAN_POINT('Ctrl Pts',(16.0811359667075,50.1215492476701,69.9693871962945)) ;
#6065=CARTESIAN_POINT('Ctrl Pts',(16.0745730607129,50.1705005823631,69.9413635189957)) ;
#6066=CARTESIAN_POINT('Ctrl Pts',(16.0391975693541,50.4409777252529,69.7863498226791)) ;
#6067=CARTESIAN_POINT('Ctrl Pts',(16.0135016772283,50.6626055143604,69.6587142024686)) ;
#6068=CARTESIAN_POINT('Ctrl Pts',(15.9808848681758,50.9851624100752,69.4720136822115)) ;
#6069=CARTESIAN_POINT('Ctrl Pts',(15.9713682691362,51.0859939056647,69.4135045221654)) ;
#6070=CARTESIAN_POINT('Ctrl Pts',(15.9476364035747,51.3568997827781,69.2560008379473)) ;
#6071=CARTESIAN_POINT('Ctrl Pts',(15.9346854871418,51.5269679364528,69.1568228822683)) ;
#6072=CARTESIAN_POINT('Ctrl Pts',(15.9138635938771,51.8494753760342,68.9684861773292)) ;
#6073=CARTESIAN_POINT('Ctrl Pts',(15.9055941627483,52.0019638251988,68.879264954564)) ;
#6074=CARTESIAN_POINT('Ctrl Pts',(15.8937230547787,52.2724926312743,68.7207266752105)) ;
#6075=CARTESIAN_POINT('Ctrl Pts',(15.8894894402357,52.3905429898142,68.6514552394551)) ;
#6076=CARTESIAN_POINT('Ctrl Pts',(15.8805247574606,52.7126477889991,68.4622522192294)) ;
#6077=CARTESIAN_POINT('Ctrl Pts',(15.8776868138709,52.9167369537098,68.342348621825)) ;
#6078=CARTESIAN_POINT('Ctrl Pts',(15.8776875119243,53.1208403600521,68.2224337443077)) ;
#6079=CARTESIAN_POINT('',(26.0416037428036,45.3830634900494,61.0679708775511)) ;
#6080=CARTESIAN_POINT('',(30.8133987679008,57.8256696110844,66.2356456049943)) ;
#6081=CARTESIAN_POINT('Ctrl Pts',(26.041604258221,45.3830652730984,61.0679709929564)) ;
#6082=CARTESIAN_POINT('Ctrl Pts',(26.1580773630691,45.593526784071,61.1097105638754)) ;
#6083=CARTESIAN_POINT('Ctrl Pts',(26.2734067453744,45.8038922450035,61.1542499492565)) ;
#6084=CARTESIAN_POINT('Ctrl Pts',(26.4141578631216,46.0632318316992,61.212585328639)) ;
#6085=CARTESIAN_POINT('Ctrl Pts',(26.4407101196587,46.1122612415126,61.2237676201864)) ;
#6086=CARTESIAN_POINT('Ctrl Pts',(26.586832843751,46.3827042839367,61.2862869523435)) ;
#6087=CARTESIAN_POINT('Ctrl Pts',(26.7052078067137,46.604012592347,61.3405705010222)) ;
#6088=CARTESIAN_POINT('Ctrl Pts',(26.8420129650536,46.8632622432158,61.4076107275278)) ;
#6089=CARTESIAN_POINT('Ctrl Pts',(26.8619485618899,46.9011261856477,61.4174887031528)) ;
#6090=CARTESIAN_POINT('Ctrl Pts',(27.0040850331528,47.1717033808736,61.4886953286622)) ;
#6091=CARTESIAN_POINT('Ctrl Pts',(27.1246612717725,47.4044689603647,61.5532259360897)) ;
#6092=CARTESIAN_POINT('Ctrl Pts',(27.257162671145,47.6638628919003,61.6288144342943)) ;
#6093=CARTESIAN_POINT('Ctrl Pts',(27.2707127104083,47.6904386808345,61.6365999303412)) ;
#6094=CARTESIAN_POINT('Ctrl Pts',(27.408558191849,47.961299863614,61.7163691635019)) ;
#6095=CARTESIAN_POINT('Ctrl Pts',(27.5307957603664,48.2057236046437,61.7918123691392)) ;
#6096=CARTESIAN_POINT('Ctrl Pts',(27.6581094410944,48.4649882125096,61.8754536832722)) ;
#6097=CARTESIAN_POINT('Ctrl Pts',(27.6655357210229,48.4801277704428,61.8803512377111)) ;
#6098=CARTESIAN_POINT('Ctrl Pts',(27.7981505933644,48.7507815722807,61.9681441307179)) ;
#6099=CARTESIAN_POINT('Ctrl Pts',(27.9209138440538,49.0060603871173,62.0547560051701)) ;
#6100=CARTESIAN_POINT('Ctrl Pts',(28.0426272365086,49.2650911286676,62.1461408986514)) ;
#6101=CARTESIAN_POINT('Ctrl Pts',(28.0443755667558,49.2688131587718,62.147454760076)) ;
#6102=CARTESIAN_POINT('Ctrl Pts',(28.1677560109025,49.5315653220715,62.2402578391401)) ;
#6103=CARTESIAN_POINT('Ctrl Pts',(28.2865807178825,49.7905771610405,62.3353500873029)) ;
#6104=CARTESIAN_POINT('Ctrl Pts',(28.4060264763688,50.0572510953393,62.4369777978504)) ;
#6105=CARTESIAN_POINT('Ctrl Pts',(28.4094629600844,50.0649289262853,62.4399069315551)) ;
#6106=CARTESIAN_POINT('Ctrl Pts',(28.5253015441136,50.3239244418434,62.538821762771)) ;
#6107=CARTESIAN_POINT('Ctrl Pts',(28.634827348025,50.5754015948757,62.6380105542769)) ;
#6108=CARTESIAN_POINT('Ctrl Pts',(28.749572034541,50.8461423400794,62.7481881019863)) ;
#6109=CARTESIAN_POINT('Ctrl Pts',(28.7576536046867,50.8652509230882,62.7559824719168)) ;
#6110=CARTESIAN_POINT('Ctrl Pts',(28.8671091242344,51.1245997230133,62.8620169997531)) ;
#6111=CARTESIAN_POINT('Ctrl Pts',(28.9659486623374,51.3650618940756,62.9632623213938)) ;
#6112=CARTESIAN_POINT('Ctrl Pts',(29.0738923449893,51.6358437425653,63.0801758596971)) ;
#6113=CARTESIAN_POINT('Ctrl Pts',(29.0860186098835,51.6663832990628,63.0934036352977)) ;
#6114=CARTESIAN_POINT('Ctrl Pts',(29.2051570782229,51.9676379850836,63.2242945123136)) ;
#6115=CARTESIAN_POINT('Ctrl Pts',(29.308462676244,52.2381644564847,63.34520603459)) ;
#6116=CARTESIAN_POINT('Ctrl Pts',(29.4877453362116,52.7256472364854,63.568885979738)) ;
#6117=CARTESIAN_POINT('Ctrl Pts',(29.5649977360443,52.9427458529092,63.6704069597754)) ;
#6118=CARTESIAN_POINT('Ctrl Pts',(29.6579933638176,53.2131562545837,63.7992211617736)) ;
#6119=CARTESIAN_POINT('Ctrl Pts',(29.6761702732096,53.2664641483689,63.8247299027501)) ;
#6120=CARTESIAN_POINT('Ctrl Pts',(29.7637337475682,53.5254861983816,63.9492332558931)) ;
#6121=CARTESIAN_POINT('Ctrl Pts',(29.830965738571,53.7311956119134,64.0498470884217)) ;
#6122=CARTESIAN_POINT('Ctrl Pts',(29.9161466063752,54.0017837515308,64.1841549976686)) ;
#6123=CARTESIAN_POINT('Ctrl Pts',(29.9362883545417,54.0665473332625,64.2164469853188)) ;
#6124=CARTESIAN_POINT('Ctrl Pts',(30.0159245403778,54.325825723567,64.3462863385794)) ;
#6125=CARTESIAN_POINT('Ctrl Pts',(30.0735321168821,54.5205088505445,64.445146658184)) ;
#6126=CARTESIAN_POINT('Ctrl Pts',(30.1505922362448,54.7914199725069,64.5845293955896)) ;
#6127=CARTESIAN_POINT('Ctrl Pts',(30.1719356271454,54.8676682916929,64.6239538372645)) ;
#6128=CARTESIAN_POINT('Ctrl Pts',(30.2674753196619,55.2146576988569,64.8042272975172)) ;
#6129=CARTESIAN_POINT('Ctrl Pts',(30.3374758773342,55.4852678000175,64.9469830214306)) ;
#6130=CARTESIAN_POINT('Ctrl Pts',(30.4444823520982,55.9272948494787,65.1836937164577)) ;
#6131=CARTESIAN_POINT('Ctrl Pts',(30.4841893015841,56.0987899530359,65.2764045819959)) ;
#6132=CARTESIAN_POINT('Ctrl Pts',(30.5438495019435,56.3691923043857,65.4237318267551)) ;
#6133=CARTESIAN_POINT('Ctrl Pts',(30.565046560445,56.4680781862336,65.4778526642952)) ;
#6134=CARTESIAN_POINT('Ctrl Pts',(30.6728078091545,56.9862401445904,65.7625708083994)) ;
#6135=CARTESIAN_POINT('Ctrl Pts',(30.7488583286256,57.4056326749329,65.9973565406346)) ;
#6136=CARTESIAN_POINT('Ctrl Pts',(30.8133954092186,57.8256477522358,66.2356332043538)) ;
#6137=CARTESIAN_POINT('',(30.8134080024022,57.8271591829153,66.2356745000382)) ;
#6138=CARTESIAN_POINT('Ctrl Pts',(30.8134023722464,57.8256930687507,66.2356589126527)) ;
#6139=CARTESIAN_POINT('Ctrl Pts',(30.8134066863751,57.8261751443407,66.2356748334161)) ;
#6140=CARTESIAN_POINT('Ctrl Pts',(30.8134071043806,57.8266671620021,66.2356747344862)) ;
#6141=CARTESIAN_POINT('Ctrl Pts',(30.8134080024022,57.8271591829153,66.2356745000382)) ;
#6142=CARTESIAN_POINT('',(30.8134078048396,58.7660385728356,66.2356745549092)) ;
#6143=CARTESIAN_POINT('',(30.8134080024022,43.8830586252741,66.2356745000382)) ;
#6144=CARTESIAN_POINT('',(25.5149631655986,45.3830586252742,60.9005821906198)) ;
#6145=CARTESIAN_POINT('Ctrl Pts',(30.8134076078136,58.766038570874,66.2356746117338)) ;
#6146=CARTESIAN_POINT('Ctrl Pts',(30.7740741903988,58.5098890944364,66.0904525970946)) ;
#6147=CARTESIAN_POINT('Ctrl Pts',(30.7303837591305,58.2537790654507,65.9462463126743)) ;
#6148=CARTESIAN_POINT('Ctrl Pts',(30.6781206959667,57.9742522431174,65.7905703303672)) ;
#6149=CARTESIAN_POINT('Ctrl Pts',(30.6736933470961,57.9507654759312,65.7775007825044)) ;
#6150=CARTESIAN_POINT('Ctrl Pts',(30.6199239898024,57.6678169639212,65.6201853252031)) ;
#6151=CARTESIAN_POINT('Ctrl Pts',(30.5662766775329,57.4086482068897,65.4774198047579)) ;
#6152=CARTESIAN_POINT('Ctrl Pts',(30.5039911943873,57.1295421623675,65.3256766635461)) ;
#6153=CARTESIAN_POINT('Ctrl Pts',(30.4995069859816,57.1095594972727,65.3148236099938)) ;
#6154=CARTESIAN_POINT('Ctrl Pts',(30.4357484934212,56.8270031281969,65.1615169533963)) ;
#6155=CARTESIAN_POINT('Ctrl Pts',(30.3722090617258,56.564476578324,65.0209656506715)) ;
#6156=CARTESIAN_POINT('Ctrl Pts',(30.231391164111,56.0195645927232,64.733153409457)) ;
#6157=CARTESIAN_POINT('Ctrl Pts',(30.1535492863315,55.7370242482923,64.5864375767227)) ;
#6158=CARTESIAN_POINT('Ctrl Pts',(30.0671126637342,55.4412538423175,64.4356750041807)) ;
#6159=CARTESIAN_POINT('Ctrl Pts',(30.0632845069496,55.4281899051451,64.4290213842513)) ;
#6160=CARTESIAN_POINT('Ctrl Pts',(29.980209397746,55.1454478704628,64.2851365736848)) ;
#6161=CARTESIAN_POINT('Ctrl Pts',(29.8965031969772,54.8754942178628,64.1500929953628)) ;
#6162=CARTESIAN_POINT('Ctrl Pts',(29.8056563100459,54.5959998499613,64.013294987841)) ;
#6163=CARTESIAN_POINT('Ctrl Pts',(29.8025330838997,54.5864072020384,64.0086033390302)) ;
#6164=CARTESIAN_POINT('Ctrl Pts',(29.7102548621509,54.3034579214823,63.8703184606095)) ;
#6165=CARTESIAN_POINT('Ctrl Pts',(29.6169368731029,54.0303635369496,63.7396467695494)) ;
#6166=CARTESIAN_POINT('Ctrl Pts',(29.5174033116676,53.7513016854052,63.609207965875)) ;
#6167=CARTESIAN_POINT('Ctrl Pts',(29.5152226671596,53.7451933157237,63.6063544218082)) ;
#6168=CARTESIAN_POINT('Ctrl Pts',(29.4142735180212,53.4626708411959,63.4744482683264)) ;
#6169=CARTESIAN_POINT('Ctrl Pts',(29.3114984136886,53.1862776071793,63.3487247516879)) ;
#6170=CARTESIAN_POINT('Ctrl Pts',(29.2036980777988,52.9072592699432,63.2251533607292)) ;
#6171=CARTESIAN_POINT('Ctrl Pts',(29.2026751441895,52.9046125716399,63.2239815002338)) ;
#6172=CARTESIAN_POINT('Ctrl Pts',(29.2016518445348,52.9019658736982,63.2228099471636)) ;
#6173=CARTESIAN_POINT('Ctrl Pts',(29.0937743039087,52.6229476375472,63.0993033444404)) ;
#6174=CARTESIAN_POINT('Ctrl Pts',(28.9818294925969,52.3439334673732,62.9792145060285)) ;
#6175=CARTESIAN_POINT('Ctrl Pts',(28.865782176196,52.0638397190087,62.8625418056171)) ;
#6176=CARTESIAN_POINT('Ctrl Pts',(28.8654435444416,52.0630224673026,62.8622014135336)) ;
#6177=CARTESIAN_POINT('Ctrl Pts',(28.8651048804777,52.0622052134034,62.8618610536397)) ;
#6178=CARTESIAN_POINT('Ctrl Pts',(28.8065187928208,51.9208269928423,62.8029815840101)) ;
#6179=CARTESIAN_POINT('Ctrl Pts',(28.7469483924193,51.7794019307221,62.7450428274934)) ;
#6180=CARTESIAN_POINT('Ctrl Pts',(28.6276680578051,51.5007457293394,62.6327818911217)) ;
#6181=CARTESIAN_POINT('Ctrl Pts',(28.5679909177056,51.3634912127544,62.5783831680472)) ;
#6182=CARTESIAN_POINT('Ctrl Pts',(28.5056907825906,51.2220958064459,62.5233816695522)) ;
#6183=CARTESIAN_POINT('Ctrl Pts',(28.5037978670285,51.2178014570208,62.5217121950908)) ;
#6184=CARTESIAN_POINT('Ctrl Pts',(28.3806353677896,50.9385050159945,62.4131971637078)) ;
#6185=CARTESIAN_POINT('Ctrl Pts',(28.2562425325705,50.6639128623093,62.3104626930187)) ;
#6186=CARTESIAN_POINT('Ctrl Pts',(28.1251946565102,50.3820631700627,62.2090567779632)) ;
#6187=CARTESIAN_POINT('Ctrl Pts',(28.1216204064942,50.374381438015,62.2062960797886)) ;
#6188=CARTESIAN_POINT('Ctrl Pts',(27.9919781190897,50.0959566887312,62.1063464520381)) ;
#6189=CARTESIAN_POINT('Ctrl Pts',(27.8630520121241,49.8255092945984,62.013263065848)) ;
#6190=CARTESIAN_POINT('Ctrl Pts',(27.7261122130716,49.5442578124092,61.9207725737991)) ;
#6191=CARTESIAN_POINT('Ctrl Pts',(27.7207631223362,49.533281035922,61.9171696510503)) ;
#6192=CARTESIAN_POINT('Ctrl Pts',(27.5852110368569,49.2553528965713,61.8261180197291)) ;
#6193=CARTESIAN_POINT('Ctrl Pts',(27.4522724975945,48.9886632517188,61.7426780639602)) ;
#6194=CARTESIAN_POINT('Ctrl Pts',(27.3098129532935,48.7077521761841,61.6592875552603)) ;
#6195=CARTESIAN_POINT('Ctrl Pts',(27.30260566038,48.6935533493115,61.6550846084527)) ;
#6196=CARTESIAN_POINT('Ctrl Pts',(27.1527029138186,48.3985015698037,61.567999345586)) ;
#6197=CARTESIAN_POINT('Ctrl Pts',(27.0073620617917,48.1176788676491,61.4897761421026)) ;
#6198=CARTESIAN_POINT('Ctrl Pts',(26.7223664286535,47.5765229674271,61.3481705003658)) ;
#6199=CARTESIAN_POINT('Ctrl Pts',(26.583304786595,47.3160356130356,61.2842340603531)) ;
#6200=CARTESIAN_POINT('Ctrl Pts',(26.4311701471226,47.0348519182515,61.2197850173879)) ;
#6201=CARTESIAN_POINT('Ctrl Pts',(26.4200560008957,47.0143316503714,61.2151078541788)) ;
#6202=CARTESIAN_POINT('Ctrl Pts',(26.2692807870402,46.7362435810598,61.1520787578222)) ;
#6203=CARTESIAN_POINT('Ctrl Pts',(26.1276801094453,46.4785159096922,61.0977909490593)) ;
#6204=CARTESIAN_POINT('Ctrl Pts',(25.9713733923796,46.1967318999707,61.0431770974691)) ;
#6205=CARTESIAN_POINT('Ctrl Pts',(25.9582359874009,46.1730689512029,61.038627292554)) ;
#6206=CARTESIAN_POINT('Ctrl Pts',(25.8033345595273,45.8942981208808,60.9854572360907)) ;
#6207=CARTESIAN_POINT('Ctrl Pts',(25.6599204237631,45.6388798207738,60.9409158281036)) ;
#6208=CARTESIAN_POINT('Ctrl Pts',(25.5149631682039,45.3830586252743,60.9005821812565)) ;
#6209=CARTESIAN_POINT('Origin',(23.47768801576,45.3830586252741,68.2224337400009)) ;
#6210=CARTESIAN_POINT('',(17.4656830216285,45.3830634900533,63.5731543704541)) ;
#6211=CARTESIAN_POINT('',(23.8549995017264,57.8256696110329,60.6318069295841)) ;
#6212=CARTESIAN_POINT('Ctrl Pts',(17.4656832906589,45.3830652731062,63.5731539159243)) ;
#6213=CARTESIAN_POINT('Ctrl Pts',(17.5413721503497,45.5935267840849,63.4752796473432)) ;
#6214=CARTESIAN_POINT('Ctrl Pts',(17.6193703621342,45.8038922449965,63.3793583137785)) ;
#6215=CARTESIAN_POINT('Ctrl Pts',(17.7183450921985,46.0632318316999,63.2635226696589)) ;
#6216=CARTESIAN_POINT('Ctrl Pts',(17.737185181951,46.1122612415128,63.2417254911808)) ;
#6217=CARTESIAN_POINT('Ctrl Pts',(17.841799005201,46.3827042839374,63.1220740583684)) ;
#6218=CARTESIAN_POINT('Ctrl Pts',(17.9300056031499,46.6040125923438,63.0262673175482)) ;
#6219=CARTESIAN_POINT('Ctrl Pts',(18.0360397662805,46.8632622432172,62.9168744495294)) ;
#6220=CARTESIAN_POINT('Ctrl Pts',(18.0515947175824,46.9011261856486,62.9009670325896)) ;
#6221=CARTESIAN_POINT('Ctrl Pts',(18.1632388279165,47.1717033808736,62.7877912727863)) ;
#6222=CARTESIAN_POINT('Ctrl Pts',(18.2618711894541,47.4044689603724,62.6930575096971)) ;
#6223=CARTESIAN_POINT('Ctrl Pts',(18.3747053074258,47.6638628918969,62.5903993209187)) ;
#6224=CARTESIAN_POINT('Ctrl Pts',(18.3862969465815,47.6904386808303,62.5799183183686)) ;
#6225=CARTESIAN_POINT('Ctrl Pts',(18.5047585919478,47.961299863605,62.4734695236722)) ;
#6226=CARTESIAN_POINT('Ctrl Pts',(18.6142828302904,48.2057236046444,62.3805279202602)) ;
#6227=CARTESIAN_POINT('Ctrl Pts',(18.733172538089,48.4649882125105,62.2852920020896)) ;
#6228=CARTESIAN_POINT('Ctrl Pts',(18.740125235855,48.4801277704437,62.2797426177243)) ;
#6229=CARTESIAN_POINT('Ctrl Pts',(18.8646014880951,48.7507815722807,62.1807478751498)) ;
#6230=CARTESIAN_POINT('Ctrl Pts',(18.984910206447,49.006060387104,62.0907576267275)) ;
#6231=CARTESIAN_POINT('Ctrl Pts',(19.1094339115856,49.2650911286613,62.0032407968347)) ;
#6232=CARTESIAN_POINT('Ctrl Pts',(19.111223731813,49.2688131587655,62.001984041469)) ;
#6233=CARTESIAN_POINT('Ctrl Pts',(19.1130140805669,49.2725351845606,62.0007280675306)) ;
#6234=CARTESIAN_POINT('Ctrl Pts',(19.2376113588956,49.5315653220715,61.9133199946472)) ;
#6235=CARTESIAN_POINT('Ctrl Pts',(19.3647683149683,49.7905771610406,61.8296961034925)) ;
#6236=CARTESIAN_POINT('Ctrl Pts',(19.4983327806004,50.0572510953383,61.747501126198)) ;
#6237=CARTESIAN_POINT('Ctrl Pts',(19.5021804841665,50.0649289262843,61.7451379880606)) ;
#6238=CARTESIAN_POINT('Ctrl Pts',(19.6320501700217,50.3239244418398,61.6655353117229)) ;
#6239=CARTESIAN_POINT('Ctrl Pts',(19.7602296512367,50.5754015948895,61.5920211044488)) ;
#6240=CARTESIAN_POINT('Ctrl Pts',(19.9004727840933,50.8461423400857,61.5169391572625)) ;
#6241=CARTESIAN_POINT('Ctrl Pts',(19.9103830129235,50.8652509230937,61.5116617200819)) ;
#6242=CARTESIAN_POINT('Ctrl Pts',(20.0450514572642,51.1245997230103,61.4403298060522)) ;
#6243=CARTESIAN_POINT('Ctrl Pts',(20.1718845771644,51.3650618940538,61.3776143442512)) ;
#6244=CARTESIAN_POINT('Ctrl Pts',(20.3164323919744,51.6358437425513,61.3110820716862)) ;
#6245=CARTESIAN_POINT('Ctrl Pts',(20.332759976084,51.6663832990502,61.3036369158996)) ;
#6246=CARTESIAN_POINT('Ctrl Pts',(20.4940604089653,51.9676379850866,61.2307770046641)) ;
#6247=CARTESIAN_POINT('Ctrl Pts',(20.6409772855714,52.2381644565101,61.1698912576762)) ;
#6248=CARTESIAN_POINT('Ctrl Pts',(20.9091109436541,52.7256472364568,61.0685042200231)) ;
#6249=CARTESIAN_POINT('Ctrl Pts',(21.0295354376883,52.9427458528919,61.0264045298722)) ;
#6250=CARTESIAN_POINT('Ctrl Pts',(21.1807822532647,53.2131562545791,60.9777662096284)) ;
#6251=CARTESIAN_POINT('Ctrl Pts',(21.2106594814961,53.2664641483671,60.9683615759732)) ;
#6252=CARTESIAN_POINT('Ctrl Pts',(21.3561278084265,53.5254861983863,60.9235574150852)) ;
#6253=CARTESIAN_POINT('Ctrl Pts',(21.472593077294,53.7311956119202,60.8907073760518)) ;
#6254=CARTESIAN_POINT('Ctrl Pts',(21.6266498253265,54.0017837515366,60.8511989830966)) ;
#6255=CARTESIAN_POINT('Ctrl Pts',(21.6635854730858,54.0665473332689,60.842021815219)) ;
#6256=CARTESIAN_POINT('Ctrl Pts',(21.8116789708385,54.3258257235488,60.8064058684495)) ;
#6257=CARTESIAN_POINT('Ctrl Pts',(21.923502442178,54.5205088505476,60.7821673262479)) ;
#6258=CARTESIAN_POINT('Ctrl Pts',(22.0798761893219,54.7914199725089,60.7519504321609)) ;
#6259=CARTESIAN_POINT('Ctrl Pts',(22.1239665319832,54.8676682916975,60.7438344836362)) ;
#6260=CARTESIAN_POINT('Ctrl Pts',(22.3249401696415,55.2146576988347,60.708678399366)) ;
#6261=CARTESIAN_POINT('Ctrl Pts',(22.4823402930707,55.4852678000144,60.6862178575749)) ;
#6262=CARTESIAN_POINT('Ctrl Pts',(22.7405323613007,55.9272948494774,60.6575962799744)) ;
#6263=CARTESIAN_POINT('Ctrl Pts',(22.8409757562831,56.0987899530342,60.6484819599386)) ;
#6264=CARTESIAN_POINT('Ctrl Pts',(22.9995283082329,56.3691923043824,60.637268359989)) ;
#6265=CARTESIAN_POINT('Ctrl Pts',(23.0575505347489,56.4680781862304,60.6338330179249)) ;
#6266=CARTESIAN_POINT('Ctrl Pts',(23.3616336382064,56.9862401445896,60.6193287252703)) ;
#6267=CARTESIAN_POINT('Ctrl Pts',(23.6084290417824,57.4056326748909,60.6195531644626)) ;
#6268=CARTESIAN_POINT('Ctrl Pts',(23.8549866701408,57.8256477522086,60.6318062918727)) ;
#6269=CARTESIAN_POINT('',(23.8550298361323,57.8271591833517,60.6318070761082)) ;
#6270=CARTESIAN_POINT('Ctrl Pts',(23.8550132718507,57.825693068674,60.6318076139396)) ;
#6271=CARTESIAN_POINT('Ctrl Pts',(23.8550297465186,57.8261751444418,60.6318084307449)) ;
#6272=CARTESIAN_POINT('Ctrl Pts',(23.8550297816016,57.8266671622709,60.6318080026266)) ;
#6273=CARTESIAN_POINT('Ctrl Pts',(23.8550298361323,57.8271591833517,60.6318070761082)) ;
#6274=CARTESIAN_POINT('',(23.8550298272675,58.7660385728413,60.6318072809575)) ;
#6275=CARTESIAN_POINT('',(23.8550298361323,43.8830586252741,60.6318070761082)) ;
#6276=CARTESIAN_POINT('',(17.1437460318932,45.3830586252742,64.0222933742113)) ;
#6277=CARTESIAN_POINT('Ctrl Pts',(23.8550298204266,58.7660385708796,60.6318074859001)) ;
#6278=CARTESIAN_POINT('Ctrl Pts',(23.7047607826612,58.5098890944426,60.624339718359)) ;
#6279=CARTESIAN_POINT('Ctrl Pts',(23.5541113704526,58.2537790654492,60.6213295951355)) ;
#6280=CARTESIAN_POINT('Ctrl Pts',(23.3899045383306,57.9742522431133,60.6229281977702)) ;
#6281=CARTESIAN_POINT('Ctrl Pts',(23.3761065336288,57.9507654759275,60.6231001443651)) ;
#6282=CARTESIAN_POINT('Ctrl Pts',(23.2098749976631,57.6678169639206,60.6256246922118)) ;
#6283=CARTESIAN_POINT('Ctrl Pts',(23.0575189879674,57.4086482068946,60.6325293460982)) ;
#6284=CARTESIAN_POINT('Ctrl Pts',(22.8939554119029,57.1295421623652,60.6448751513013)) ;
#6285=CARTESIAN_POINT('Ctrl Pts',(22.8822478479962,57.1095594972706,60.6457861089375)) ;
#6286=CARTESIAN_POINT('Ctrl Pts',(22.7167420955076,56.8270031281923,60.6590496765166)) ;
#6287=CARTESIAN_POINT('Ctrl Pts',(22.5634350990063,56.5644765783291,60.6760465259443)) ;
#6288=CARTESIAN_POINT('Ctrl Pts',(22.2461942679969,56.0195645927191,60.7210334313653)) ;
#6289=CARTESIAN_POINT('Ctrl Pts',(22.0826047561317,55.7370242483032,60.7497277708092)) ;
#6290=CARTESIAN_POINT('Ctrl Pts',(21.9125106437908,55.4412538423216,60.7853456869443)) ;
#6291=CARTESIAN_POINT('Ctrl Pts',(21.9049997096968,55.428189905149,60.7869303987674)) ;
#6292=CARTESIAN_POINT('Ctrl Pts',(21.7424855024646,55.1454478704628,60.8214766710187)) ;
#6293=CARTESIAN_POINT('Ctrl Pts',(21.5881847887512,54.8754942178679,60.8593552380298)) ;
#6294=CARTESIAN_POINT('Ctrl Pts',(21.430008920329,54.5959998499605,60.9034828527113)) ;
#6295=CARTESIAN_POINT('Ctrl Pts',(21.4245817671989,54.5864072020377,60.9050034180752)) ;
#6296=CARTESIAN_POINT('Ctrl Pts',(21.2645494937397,54.3034579214823,60.9500328446847)) ;
#6297=CARTESIAN_POINT('Ctrl Pts',(21.111436485969,54.0303635369511,60.9984037530338)) ;
#6298=CARTESIAN_POINT('Ctrl Pts',(20.9566242497591,53.7513016854048,61.0527579881668)) ;
#6299=CARTESIAN_POINT('Ctrl Pts',(20.9532365118681,53.7451933157233,61.053950110725)) ;
#6300=CARTESIAN_POINT('Ctrl Pts',(20.7965913024079,53.4626708411959,61.1091972137392)) ;
#6301=CARTESIAN_POINT('Ctrl Pts',(20.6452618788204,53.186277607177,61.1680914431933)) ;
#6302=CARTESIAN_POINT('Ctrl Pts',(20.4944263664219,52.9072592699496,61.2324299952799)) ;
#6303=CARTESIAN_POINT('Ctrl Pts',(20.4929957569922,52.9046125716463,61.2330407381467)) ;
#6304=CARTESIAN_POINT('Ctrl Pts',(20.3407675741267,52.6229476375602,61.2980839229628)) ;
#6305=CARTESIAN_POINT('Ctrl Pts',(20.1919634527057,52.3439334673782,61.3674402733172)) ;
#6306=CARTESIAN_POINT('Ctrl Pts',(20.0451405277899,52.0638397190112,61.4417539825704)) ;
#6307=CARTESIAN_POINT('Ctrl Pts',(20.0447121527138,52.0630224673051,61.4419708535685)) ;
#6308=CARTESIAN_POINT('Ctrl Pts',(20.0442837982987,52.0622052134059,61.4421877651467)) ;
#6309=CARTESIAN_POINT('Ctrl Pts',(19.9701819983144,51.9208269928453,61.4797116888403)) ;
#6310=CARTESIAN_POINT('Ctrl Pts',(19.8966707002981,51.7794019307423,61.5184624459233)) ;
#6311=CARTESIAN_POINT('Ctrl Pts',(19.7530445547343,51.5007457293231,61.5972142482874)) ;
#6312=CARTESIAN_POINT('Ctrl Pts',(19.6828670441985,51.3634912127728,61.6371604513572)) ;
#6313=CARTESIAN_POINT('Ctrl Pts',(19.6113057101537,51.2220958064568,61.6794150030693)) ;
#6314=CARTESIAN_POINT('Ctrl Pts',(19.6091330025111,51.2178014570316,61.680699376769)) ;
#6315=CARTESIAN_POINT('Ctrl Pts',(19.4678697694841,50.9385050159871,61.7643008853794)) ;
#6316=CARTESIAN_POINT('Ctrl Pts',(19.3317239816368,50.6639128622978,61.8508588045359)) ;
#6317=CARTESIAN_POINT('Ctrl Pts',(19.1947852045447,50.3820631700569,61.9441565899327)) ;
#6318=CARTESIAN_POINT('Ctrl Pts',(19.1910551205589,50.3743814380095,61.9467028010492)) ;
#6319=CARTESIAN_POINT('Ctrl Pts',(19.0559357057821,50.0959566887385,62.03911380972)) ;
#6320=CARTESIAN_POINT('Ctrl Pts',(18.9275677867106,49.8255092946014,62.132965475648)) ;
#6321=CARTESIAN_POINT('Ctrl Pts',(18.7972873764406,49.5442578124104,62.2346218300143)) ;
#6322=CARTESIAN_POINT('Ctrl Pts',(18.792207833341,49.5332810359232,62.2385957532556)) ;
#6323=CARTESIAN_POINT('Ctrl Pts',(18.663724688025,49.2553528965829,62.3393769459986)) ;
#6324=CARTESIAN_POINT('Ctrl Pts',(18.5432883065279,48.9886632517177,62.4400246456917)) ;
#6325=CARTESIAN_POINT('Ctrl Pts',(18.4199567996313,48.7077521761834,62.5497426392499)) ;
#6326=CARTESIAN_POINT('Ctrl Pts',(18.4137323836886,48.6935533493109,62.5552984001501)) ;
#6327=CARTESIAN_POINT('Ctrl Pts',(18.284586880776,48.3985015698064,62.6709535578915)) ;
#6328=CARTESIAN_POINT('Ctrl Pts',(18.1652794001422,48.1176788676501,62.7850086230464)) ;
#6329=CARTESIAN_POINT('Ctrl Pts',(17.9425359378238,47.5765229674263,63.012297027301)) ;
#6330=CARTESIAN_POINT('Ctrl Pts',(17.8387563592619,47.3160356130502,63.1247950616225)) ;
#6331=CARTESIAN_POINT('Ctrl Pts',(17.7304494879593,47.0348519182585,63.2495678522903)) ;
#6332=CARTESIAN_POINT('Ctrl Pts',(17.7225667813501,47.0143316503778,63.2586927105645)) ;
#6333=CARTESIAN_POINT('Ctrl Pts',(17.6160304451424,46.7362435810516,63.3826113982718)) ;
#6334=CARTESIAN_POINT('Ctrl Pts',(17.5206426550712,46.478515909689,63.5005057899146)) ;
#6335=CARTESIAN_POINT('Ctrl Pts',(17.4204003637262,46.1967318999692,63.6322857034532)) ;
#6336=CARTESIAN_POINT('Ctrl Pts',(17.4120135607131,46.1730689512017,63.6433741510259)) ;
#6337=CARTESIAN_POINT('Ctrl Pts',(17.3135786583707,45.8942981208826,63.7742637123565)) ;
#6338=CARTESIAN_POINT('Ctrl Pts',(17.2268998568785,45.6388798207739,63.8968946086769)) ;
#6339=CARTESIAN_POINT('Ctrl Pts',(17.1437460237932,45.3830586252743,64.0222933688401)) ;
#6340=CARTESIAN_POINT('Origin',(23.47768801576,45.3830586252741,68.2224337400009)) ;
#6341=CARTESIAN_POINT('',(25.608724379063,45.3830634900508,75.5175476338228)) ;
#6342=CARTESIAN_POINT('',(18.7107781165901,57.8256696109658,74.1416017005878)) ;
#6343=CARTESIAN_POINT('Ctrl Pts',(25.6087238942477,45.3830652731009,75.5175478434128)) ;
#6344=CARTESIAN_POINT('Ctrl Pts',(25.4899612688168,45.5935267840753,75.5522409945192)) ;
#6345=CARTESIAN_POINT('Ctrl Pts',(25.3704782447056,45.8038922449995,75.5839967849029)) ;
#6346=CARTESIAN_POINT('Ctrl Pts',(25.2223195227794,46.0632318317002,75.6195339028655)) ;
#6347=CARTESIAN_POINT('Ctrl Pts',(25.1942655099435,46.1122612415132,75.6260942637752)) ;
#6348=CARTESIAN_POINT('Ctrl Pts',(25.0393018014623,46.3827042839383,75.6614038438299)) ;
#6349=CARTESIAN_POINT('Ctrl Pts',(24.9116273753729,46.6040125923255,75.6870665879016)) ;
#6350=CARTESIAN_POINT('Ctrl Pts',(24.7615444208957,46.8632622432174,75.7132419598636)) ;
#6351=CARTESIAN_POINT('Ctrl Pts',(24.7396100558675,46.9011261856493,75.716968359529)) ;
#6352=CARTESIAN_POINT('Ctrl Pts',(24.5827650307564,47.1717033808735,75.7429067110011)) ;
#6353=CARTESIAN_POINT('Ctrl Pts',(24.4472866652317,47.4044689603717,75.7615732877718)) ;
#6354=CARTESIAN_POINT('Ctrl Pts',(24.2956609768662,47.6638628918981,75.778303276605)) ;
#6355=CARTESIAN_POINT('Ctrl Pts',(24.2801225650689,47.690438680832,75.7799691912404)) ;
#6356=CARTESIAN_POINT('Ctrl Pts',(24.1217160491427,47.9612998636085,75.7964580670714)) ;
#6357=CARTESIAN_POINT('Ctrl Pts',(23.9784793752071,48.2057236046616,75.8072726716508)) ;
#6358=CARTESIAN_POINT('Ctrl Pts',(23.8263173129591,48.4649882125116,75.814438531032)) ;
#6359=CARTESIAN_POINT('Ctrl Pts',(23.8174306160203,48.4801277704447,75.8148413840814)) ;
#6360=CARTESIAN_POINT('Ctrl Pts',(23.6585395628197,48.7507815722807,75.8217645078505)) ;
#6361=CARTESIAN_POINT('Ctrl Pts',(23.5083128242133,49.0060603870971,75.8238524577829)) ;
#6362=CARTESIAN_POINT('Ctrl Pts',(23.3561299286236,49.265091128657,75.8214618630187)) ;
#6363=CARTESIAN_POINT('Ctrl Pts',(23.3539432313732,49.2688131587613,75.8214265695334)) ;
#6364=CARTESIAN_POINT('Ctrl Pts',(23.1995780740611,49.5315653220715,75.8188685069308)) ;
#6365=CARTESIAN_POINT('Ctrl Pts',(23.0475530456853,49.7905771610406,75.811780672505)) ;
#6366=CARTESIAN_POINT('Ctrl Pts',(22.8911841276718,50.0572510953345,75.7997705828591)) ;
#6367=CARTESIAN_POINT('Ctrl Pts',(22.8866822523511,50.0649289262804,75.799420778361)) ;
#6368=CARTESIAN_POINT('Ctrl Pts',(22.7348261902374,50.3239244418333,75.7874852102496)) ;
#6369=CARTESIAN_POINT('Ctrl Pts',(22.5879162447379,50.5754015948824,75.7716174445575)) ;
#6370=CARTESIAN_POINT('Ctrl Pts',(22.4303251056493,50.8461423400821,75.7499271705742)) ;
#6371=CARTESIAN_POINT('Ctrl Pts',(22.4192055623634,50.8652509230905,75.7483716205869)) ;
#6372=CARTESIAN_POINT('Ctrl Pts',(22.2683286552059,51.1245997230184,75.7269242257462)) ;
#6373=CARTESIAN_POINT('Ctrl Pts',(22.1288552822128,51.3650618940492,75.7031114627724)) ;
#6374=CARTESIAN_POINT('Ctrl Pts',(21.9728069549191,51.6358437425482,75.6719741281559)) ;
#6375=CARTESIAN_POINT('Ctrl Pts',(21.9552215091257,51.6663832990475,75.668400272568)) ;
#6376=CARTESIAN_POINT('Ctrl Pts',(21.7819007364219,51.9676379851017,75.6325351633311)) ;
#6377=CARTESIAN_POINT('Ctrl Pts',(21.6272547423225,52.2381644564706,75.5954371939749)) ;
#6378=CARTESIAN_POINT('Ctrl Pts',(21.3507362506827,52.7256472364779,75.5198560205866)) ;
#6379=CARTESIAN_POINT('Ctrl Pts',(21.2285652114554,52.9427458528933,75.4831316437627)) ;
#6380=CARTESIAN_POINT('Ctrl Pts',(21.077615079979,53.2131562545778,75.4335802237679)) ;
#6381=CARTESIAN_POINT('Ctrl Pts',(21.0479159896309,53.266464148367,75.4236273380877)) ;
#6382=CARTESIAN_POINT('Ctrl Pts',(20.9038944160104,53.5254861983966,75.3743705284267)) ;
#6383=CARTESIAN_POINT('Ctrl Pts',(20.7903632657492,53.7311956119258,75.332490200822)) ;
#6384=CARTESIAN_POINT('Ctrl Pts',(20.6425062877679,54.0017837515375,75.2739008776323)) ;
#6385=CARTESIAN_POINT('Ctrl Pts',(20.6072305170954,54.0665473332692,75.2596151333686)) ;
#6386=CARTESIAN_POINT('Ctrl Pts',(20.4664858323946,54.3258257235614,75.2013818656345)) ;
#6387=CARTESIAN_POINT('Ctrl Pts',(20.3617716860696,54.5205088505461,75.1552630708817)) ;
#6388=CARTESIAN_POINT('Ctrl Pts',(20.2175016224408,54.7914199725073,75.0877948692979)) ;
#6389=CARTESIAN_POINT('Ctrl Pts',(20.1770613510901,54.8676682916958,75.0684451563956)) ;
#6390=CARTESIAN_POINT('Ctrl Pts',(19.9938060349454,55.2146576988565,74.9787576857131)) ;
#6391=CARTESIAN_POINT('Ctrl Pts',(19.8532646849623,55.4852677999964,74.904411174471)) ;
#6392=CARTESIAN_POINT('Ctrl Pts',(19.6275595727133,55.9272948494813,74.7758050271755)) ;
#6393=CARTESIAN_POINT('Ctrl Pts',(19.5409418963078,56.0987899530378,74.724139520722)) ;
#6394=CARTESIAN_POINT('Ctrl Pts',(19.4060789986044,56.3691923043834,74.6400166619002)) ;
#6395=CARTESIAN_POINT('Ctrl Pts',(19.3571187878985,56.4680781862293,74.6086913029594)) ;
#6396=CARTESIAN_POINT('Ctrl Pts',(19.1025849801468,56.9862401445611,74.4416899585013)) ;
#6397=CARTESIAN_POINT('Ctrl Pts',(18.9030552265289,57.405632674834,74.2964456847875)) ;
#6398=CARTESIAN_POINT('Ctrl Pts',(18.710788122709,57.8256477521734,74.1416097587122)) ;
#6399=CARTESIAN_POINT('',(18.7107539506873,57.8265499698715,74.1415834028921)) ;
#6400=CARTESIAN_POINT('Ctrl Pts',(18.7107673785944,57.8256930685744,74.1415930530686)) ;
#6401=CARTESIAN_POINT('Ctrl Pts',(18.7107545283917,57.8259720707006,74.1415827059215)) ;
#6402=CARTESIAN_POINT('Ctrl Pts',(18.7107544336864,57.8262610185798,74.1415828059768)) ;
#6403=CARTESIAN_POINT('Ctrl Pts',(18.7107542314619,57.8265499693315,74.1415830471385)) ;
#6404=CARTESIAN_POINT('',(18.7107537892754,58.7660385728357,74.1415835914416)) ;
#6405=CARTESIAN_POINT('',(18.7107536616963,43.8830586252741,74.1415837519576)) ;
#6406=CARTESIAN_POINT('',(26.1331741575238,45.3830586252742,75.3434163616778)) ;
#6407=CARTESIAN_POINT('Ctrl Pts',(18.7107539152721,58.766038570874,74.1415834296607)) ;
#6408=CARTESIAN_POINT('Ctrl Pts',(18.827934676918,58.5098890944341,74.2359509047808)) ;
#6409=CARTESIAN_POINT('Ctrl Pts',(18.948043305545,58.2537790654364,74.3269356483841)) ;
#6410=CARTESIAN_POINT('Ctrl Pts',(19.0818290583823,57.9742522431095,74.4221607059362)) ;
#6411=CARTESIAN_POINT('Ctrl Pts',(19.0930929463476,57.9507654759241,74.430131861894)) ;
#6412=CARTESIAN_POINT('Ctrl Pts',(19.2290609759425,57.66781696392,74.5257979050929)) ;
#6413=CARTESIAN_POINT('Ctrl Pts',(19.3563780307201,57.4086482069147,74.6097645383633)) ;
#6414=CARTESIAN_POINT('Ctrl Pts',(19.49596042564,57.1295421623709,74.6959168299655)) ;
#6415=CARTESIAN_POINT('Ctrl Pts',(19.5059674912669,57.1095594972761,74.7020613831611)) ;
#6416=CARTESIAN_POINT('Ctrl Pts',(19.6476605871094,56.8270031281938,74.7886127720636)) ;
#6417=CARTESIAN_POINT('Ctrl Pts',(19.7816790500644,56.5644765783529,74.8649736236426)) ;
#6418=CARTESIAN_POINT('Ctrl Pts',(20.0647749132364,56.0195645927199,75.0150479345363)) ;
#6419=CARTESIAN_POINT('Ctrl Pts',(20.2139877179671,55.7370242483082,75.0879892287777)) ;
#6420=CARTESIAN_POINT('Ctrl Pts',(20.3725324313107,55.4412538423241,75.1591525400536)) ;
#6421=CARTESIAN_POINT('Ctrl Pts',(20.379540374875,55.4281899051513,75.1622852975488)) ;
#6422=CARTESIAN_POINT('Ctrl Pts',(20.5313229197007,55.1454478704631,75.2298602305026)) ;
#6423=CARTESIAN_POINT('Ctrl Pts',(20.6784192824002,54.8754942178506,75.2899115100048)) ;
#6424=CARTESIAN_POINT('Ctrl Pts',(20.8323238091829,54.5959998499574,75.3471849625336)) ;
#6425=CARTESIAN_POINT('Ctrl Pts',(20.8376082341926,54.5864072020347,75.349144799885)) ;
#6426=CARTESIAN_POINT('Ctrl Pts',(20.9935446959547,54.3034579214823,75.4067798387431)) ;
#6427=CARTESIAN_POINT('Ctrl Pts',(21.1458474278724,54.0303635369504,75.4576445197581)) ;
#6428=CARTESIAN_POINT('Ctrl Pts',(21.3030417757119,53.7513016854057,75.5046673691372)) ;
#6429=CARTESIAN_POINT('Ctrl Pts',(21.3064832252968,53.7451933157242,75.5056941840992)) ;
#6430=CARTESIAN_POINT('Ctrl Pts',(21.4656852942199,53.4626708411959,75.5530720828333)) ;
#6431=CARTESIAN_POINT('Ctrl Pts',(21.6227305291694,53.1862776071773,75.5943748537571)) ;
#6432=CARTESIAN_POINT('Ctrl Pts',(21.7825762741261,52.9072592699501,75.6309827614355)) ;
#6433=CARTESIAN_POINT('Ctrl Pts',(21.7840926471172,52.9046125716468,75.6313295512016)) ;
#6434=CARTESIAN_POINT('Ctrl Pts',(21.945479258876,52.6229476375612,75.6681859901889)) ;
#6435=CARTESIAN_POINT('Ctrl Pts',(22.1066309618375,52.3439334673839,75.6995403921371)) ;
#6436=CARTESIAN_POINT('Ctrl Pts',(22.2690937055957,52.063839719014,75.7257196883994)) ;
#6437=CARTESIAN_POINT('Ctrl Pts',(22.2695677418866,52.0630224673079,75.7257960286286)) ;
#6438=CARTESIAN_POINT('Ctrl Pts',(22.2700417853147,52.0622052134087,75.7258723238834)) ;
#6439=CARTESIAN_POINT('Ctrl Pts',(22.3520474097712,51.9208269928421,75.7390707771187)) ;
#6440=CARTESIAN_POINT('Ctrl Pts',(22.4342964226827,51.7794019307305,75.7509296129456)) ;
#6441=CARTESIAN_POINT('Ctrl Pts',(22.5967815632748,51.5007457293469,75.771639396698)) ;
#6442=CARTESIAN_POINT('Ctrl Pts',(22.6770361509753,51.3634912127619,75.78057154529)) ;
#6443=CARTESIAN_POINT('Ctrl Pts',(22.7597670886974,51.2220958064525,75.7884495916514)) ;
#6444=CARTESIAN_POINT('Ctrl Pts',(22.7622797820233,51.2178014570273,75.7886875970111)) ;
#6445=CARTESIAN_POINT('Ctrl Pts',(22.9257038720592,50.9385050159947,75.8040850008551)) ;
#6446=CARTESIAN_POINT('Ctrl Pts',(23.086725596493,50.6639128622994,75.8140826595182)) ;
#6447=CARTESIAN_POINT('Ctrl Pts',(23.2523504566757,50.3820631700578,75.8190937592362)) ;
#6448=CARTESIAN_POINT('Ctrl Pts',(23.2568647833541,50.3743814380103,75.8192263195284)) ;
#6449=CARTESIAN_POINT('Ctrl Pts',(23.4204965142258,50.0959566887354,75.8238854423506)) ;
#6450=CARTESIAN_POINT('Ctrl Pts',(23.5795129674232,49.8255092946031,75.8234106193621)) ;
#6451=CARTESIAN_POINT('Ctrl Pts',(23.7446641392626,49.5442578124114,75.8177458049129)) ;
#6452=CARTESIAN_POINT('Ctrl Pts',(23.7511093894287,49.5332810359241,75.8175165139986)) ;
#6453=CARTESIAN_POINT('Ctrl Pts',(23.9142921362852,49.2553528965747,75.811503314341)) ;
#6454=CARTESIAN_POINT('Ctrl Pts',(24.0708864491977,48.98866325171,75.8008683437293)) ;
#6455=CARTESIAN_POINT('Ctrl Pts',(24.2351543527481,48.7077521761783,75.7845970632484)) ;
#6456=CARTESIAN_POINT('Ctrl Pts',(24.2434556053485,48.693553349306,75.7837609781587)) ;
#6457=CARTESIAN_POINT('Ctrl Pts',(24.4159169080327,48.3985015698049,75.76610381207)) ;
#6458=CARTESIAN_POINT('Ctrl Pts',(24.5794785726484,48.1176788676782,75.7439585036729)) ;
#6459=CARTESIAN_POINT('Ctrl Pts',(24.893278591109,47.5765229673886,75.6910036441987)) ;
#6460=CARTESIAN_POINT('Ctrl Pts',(25.0433627192943,47.3160356130354,75.6609909283725)) ;
#6461=CARTESIAN_POINT('Ctrl Pts',(25.2043244250407,47.0348519182514,75.6237088019572)) ;
#6462=CARTESIAN_POINT('Ctrl Pts',(25.2160651257732,47.0143316503714,75.6209599752349)) ;
#6463=CARTESIAN_POINT('Ctrl Pts',(25.3750924094244,46.7362435810525,75.5833281382101)) ;
#6464=CARTESIAN_POINT('Ctrl Pts',(25.5215593373602,46.4785159096822,75.5440171080885)) ;
#6465=CARTESIAN_POINT('Ctrl Pts',(25.6801153443456,46.196731899966,75.4963258590251)) ;
#6466=CARTESIAN_POINT('Ctrl Pts',(25.6934180364662,46.1730689511987,75.4922847556223)) ;
#6467=CARTESIAN_POINT('Ctrl Pts',(25.8499884991378,45.894298120883,75.444251460025)) ;
#6468=CARTESIAN_POINT('Ctrl Pts',(25.9921937549264,45.638879820774,75.3959895020703)) ;
#6469=CARTESIAN_POINT('Ctrl Pts',(26.1331741609196,45.3830586252743,75.3434163707842)) ;
#6470=CARTESIAN_POINT('Origin',(23.47768801576,45.3830586252741,68.2224337400009)) ;
#6471=CARTESIAN_POINT('Origin',(58.47768801576,45.3830586252741,68.1724337400008)) ;
#6472=CARTESIAN_POINT('',(31.2758081909614,45.3830610445957,68.222429730099)) ;
#6473=CARTESIAN_POINT('',(51.7933248065259,45.3830586252741,68.2224337400008)) ;
#6474=CARTESIAN_POINT('',(31.2758081909603,45.3830586252741,68.2224337400009)) ;
#6475=CARTESIAN_POINT('Ctrl Pts',(31.2758081909618,45.3830586252741,68.2224282704332)) ;
#6476=CARTESIAN_POINT('Ctrl Pts',(31.2619815052159,45.3830586252741,68.2224282693451)) ;
#6477=CARTESIAN_POINT('Ctrl Pts',(31.248244467626,45.3830586252741,68.2241023785107)) ;
#6478=CARTESIAN_POINT('Ctrl Pts',(31.2203040134215,45.3830586252741,68.23092080966)) ;
#6479=CARTESIAN_POINT('Ctrl Pts',(31.2063378307747,45.3830586252741,68.2362851030096)) ;
#6480=CARTESIAN_POINT('Ctrl Pts',(31.1691061004754,45.3830586252741,68.2559255255466)) ;
#6481=CARTESIAN_POINT('Ctrl Pts',(31.1481050711888,45.3830586252741,68.2736067598549)) ;
#6482=CARTESIAN_POINT('Ctrl Pts',(31.1120389980945,45.3830586252741,68.3173139549359)) ;
#6483=CARTESIAN_POINT('Ctrl Pts',(31.097829072345,45.3830586252736,68.3436048263349)) ;
#6484=CARTESIAN_POINT('Ctrl Pts',(31.0797781562955,45.3830586252736,68.3967923257375)) ;
#6485=CARTESIAN_POINT('Ctrl Pts',(31.0750788916455,45.3830586252741,68.4233474108136)) ;
#6486=CARTESIAN_POINT('Ctrl Pts',(31.0742802400156,45.3830586252741,68.4500085087909)) ;
#6487=CARTESIAN_POINT('',(31.2729697953901,45.3830674541112,68.1224191093439)) ;
#6488=CARTESIAN_POINT('Ctrl Pts',(31.0707352963726,45.3830586252741,67.897420987276)) ;
#6489=CARTESIAN_POINT('Ctrl Pts',(31.0718578683993,45.3830586252741,67.9236365013638)) ;
#6490=CARTESIAN_POINT('Ctrl Pts',(31.0767528122927,45.3830586252745,67.9497000931763)) ;
#6491=CARTESIAN_POINT('Ctrl Pts',(31.0950990117691,45.3830586252745,68.0023971425259)) ;
#6492=CARTESIAN_POINT('Ctrl Pts',(31.1095495115892,45.3830586252741,68.0286334382962)) ;
#6493=CARTESIAN_POINT('Ctrl Pts',(31.1460384959778,45.3830586252741,68.0721480965577)) ;
#6494=CARTESIAN_POINT('Ctrl Pts',(31.1672243458983,45.3830586252741,68.0897024121122)) ;
#6495=CARTESIAN_POINT('Ctrl Pts',(31.2044592007308,45.3830586252741,68.1089700371596)) ;
#6496=CARTESIAN_POINT('Ctrl Pts',(31.2182435715767,45.3830586252741,68.1141717381528)) ;
#6497=CARTESIAN_POINT('Ctrl Pts',(31.2457964764012,45.3830586252741,68.1207877758046)) ;
#6498=CARTESIAN_POINT('Ctrl Pts',(31.2593403999271,45.3830586252741,68.1224138614655)) ;
#6499=CARTESIAN_POINT('Ctrl Pts',(31.2729697270889,45.3830586252741,68.1224137848817)) ;
#6500=CARTESIAN_POINT('',(50.6143421942707,45.3830586252741,68.1224337400008)) ;
#6501=CARTESIAN_POINT('',(50.6143421942707,45.3830586252741,68.1224337400008)) ;
#6502=CARTESIAN_POINT('Origin',(50.6143421942707,45.3830586252741,75.1224337400008)) ;
#6503=CARTESIAN_POINT('Ctrl Pts',(30.9776880157584,45.3830502402145,68.2224288733178)) ;
#6504=CARTESIAN_POINT('Ctrl Pts',(30.9776882407603,45.980480894371,68.5691772383443)) ;
#6505=CARTESIAN_POINT('Ctrl Pts',(30.9456943379727,46.5779115664506,68.9144464359756)) ;
#6506=CARTESIAN_POINT('Ctrl Pts',(30.9137006601855,47.1753380370388,69.2597132054666)) ;
#6507=CARTESIAN_POINT('Ctrl Pts',(30.8499862633892,47.772764507627,69.6005551236251)) ;
#6508=CARTESIAN_POINT('Ctrl Pts',(30.786271866593,48.3701909782152,69.9413970417837)) ;
#6509=CARTESIAN_POINT('Ctrl Pts',(30.6913803395561,48.9676174488035,70.2749061655415)) ;
#6510=CARTESIAN_POINT('Ctrl Pts',(30.5964888125192,49.5650439193917,70.6084152892993)) ;
#6511=CARTESIAN_POINT('Ctrl Pts',(30.4712297362926,50.16247038998,70.9317462364045)) ;
#6512=CARTESIAN_POINT('Ctrl Pts',(30.345970660066,50.7598968605682,71.2550771835097)) ;
#6513=CARTESIAN_POINT('Ctrl Pts',(30.1914127009229,51.3573233311564,71.5654714083249)) ;
#6514=CARTESIAN_POINT('Ctrl Pts',(30.0368547417798,51.9547498017447,71.8758656331401)) ;
#6515=CARTESIAN_POINT('Ctrl Pts',(29.8543165337321,52.5521762723329,72.170674961581)) ;
#6516=CARTESIAN_POINT('Ctrl Pts',(29.6717783256843,53.1496027429211,72.465484290022)) ;
#6517=CARTESIAN_POINT('Ctrl Pts',(29.4628172203617,53.7470292135094,72.7421935128453)) ;
#6518=CARTESIAN_POINT('Ctrl Pts',(29.2538561150392,54.3444556840976,73.0189027356686)) ;
#6519=CARTESIAN_POINT('Ctrl Pts',(29.0202548949149,54.9418821546858,73.27515106735)) ;
#6520=CARTESIAN_POINT('Ctrl Pts',(28.7866536747906,55.5393086252741,73.5313993990315)) ;
#6521=CARTESIAN_POINT('Ctrl Pts',(28.5304053431091,56.1367350958623,73.7650006191558)) ;
#6522=CARTESIAN_POINT('Ctrl Pts',(28.2741570114277,56.7341615664505,73.9986018392801)) ;
#6523=CARTESIAN_POINT('Ctrl Pts',(27.9974477886044,57.3315880370388,74.2075629446027)) ;
#6524=CARTESIAN_POINT('Ctrl Pts',(27.7539946265433,57.8572133193466,74.3914102385941)) ;
#6525=CARTESIAN_POINT('Ctrl Pts',(27.4964139865824,58.3830758086166,74.5548773103327)) ;
#6526=CARTESIAN_POINT('Ctrl Pts',(58.4776880157526,45.3830502402145,68.2224110288131)) ;
#6527=CARTESIAN_POINT('Ctrl Pts',(58.4776890657616,45.980480894371,69.8405700656033)) ;
#6528=CARTESIAN_POINT('Ctrl Pts',(58.3283841860862,46.5779115664505,71.4518263212164)) ;
#6529=CARTESIAN_POINT('Ctrl Pts',(58.1790803564124,47.1753380370388,73.0630712455076)) ;
#6530=CARTESIAN_POINT('Ctrl Pts',(57.8817465046965,47.772764507627,74.6536668635808)) ;
#6531=CARTESIAN_POINT('Ctrl Pts',(57.5844126529807,48.3701909782152,76.2442624816539)) ;
#6532=CARTESIAN_POINT('Ctrl Pts',(57.1415855268086,48.9676174488035,77.8006383925237)) ;
#6533=CARTESIAN_POINT('Ctrl Pts',(56.6987584006366,49.5650439193917,79.3570143033935)) ;
#6534=CARTESIAN_POINT('Ctrl Pts',(56.1142160449124,50.16247038998,80.8658920565512)) ;
#6535=CARTESIAN_POINT('Ctrl Pts',(55.5296736891883,50.7598968605682,82.3747698097088)) ;
#6536=CARTESIAN_POINT('Ctrl Pts',(54.8084032131872,51.3573233311564,83.8232761921796)) ;
#6537=CARTESIAN_POINT('Ctrl Pts',(54.0871327371861,51.9547498017447,85.2717825746505)) ;
#6538=CARTESIAN_POINT('Ctrl Pts',(53.2352877662965,52.5521762723329,86.6475594407083)) ;
#6539=CARTESIAN_POINT('Ctrl Pts',(52.3834427954069,53.1496027429211,88.023336306766)) ;
#6540=CARTESIAN_POINT('Ctrl Pts',(51.4082909705684,53.7470292135094,89.3146460132748)) ;
#6541=CARTESIAN_POINT('Ctrl Pts',(50.4331391457298,54.3444556840976,90.6059557197835)) ;
#6542=CARTESIAN_POINT('Ctrl Pts',(49.3430001184831,54.9418821546858,91.8017812676303)) ;
#6543=CARTESIAN_POINT('Ctrl Pts',(48.2528610912363,55.5393086252741,92.9976068154771)) ;
#6544=CARTESIAN_POINT('Ctrl Pts',(47.0570355433895,56.1367350958623,94.0877458427239)) ;
#6545=CARTESIAN_POINT('Ctrl Pts',(45.8612099955427,56.7341615664505,95.1778848699707)) ;
#6546=CARTESIAN_POINT('Ctrl Pts',(44.569900289034,57.3315880370388,96.1530366948092)) ;
#6547=CARTESIAN_POINT('Ctrl Pts',(43.4337855327491,57.8572133193466,97.010990733436)) ;
#6548=CARTESIAN_POINT('Ctrl Pts',(42.2317425462647,58.3830758086166,97.7738370682162)) ;
#6549=CARTESIAN_POINT('',(38.075012827077,58.3353824278239,91.0374682134905)) ;
#6550=CARTESIAN_POINT('',(27.7402393245935,58.2172712656981,74.7524658824537)) ;
#6551=CARTESIAN_POINT('Ctrl Pts',(38.075012827077,58.3353824278239,91.0374682134905)) ;
#6552=CARTESIAN_POINT('Ctrl Pts',(36.6930174593637,58.3308357083915,88.859791972123)) ;
#6553=CARTESIAN_POINT('Ctrl Pts',(35.1441429605084,58.3244410146232,86.4191562972014)) ;
#6554=CARTESIAN_POINT('Ctrl Pts',(32.4831083179517,58.3066351812267,82.2260366573432)) ;
#6555=CARTESIAN_POINT('Ctrl Pts',(29.560342929611,58.2895264404741,77.6204953552679)) ;
#6556=CARTESIAN_POINT('Ctrl Pts',(27.7402370295205,58.2172696107898,74.7524673806459)) ;
#6557=CARTESIAN_POINT('Ctrl Pts',(27.7402393245935,58.2172712656981,74.7524658824537)) ;
#6558=CARTESIAN_POINT('Ctrl Pts',(27.8754462121168,57.9495340002387,74.6642065097652)) ;
#6559=CARTESIAN_POINT('Ctrl Pts',(28.0078544340238,57.681908404589,74.5717785787589)) ;
#6560=CARTESIAN_POINT('Ctrl Pts',(28.1371412783914,57.4145313636563,74.4754405303686)) ;
#6561=CARTESIAN_POINT('Ctrl Pts',(28.2571575918273,57.1663266301653,74.3860104149692)) ;
#6562=CARTESIAN_POINT('Ctrl Pts',(28.3745205791364,56.9182638872705,74.2931869169747)) ;
#6563=CARTESIAN_POINT('Ctrl Pts',(28.489080577214,56.6702295478714,74.1970972024028)) ;
#6564=CARTESIAN_POINT('Ctrl Pts',(28.4979296409396,56.6510704023379,74.189674855843)) ;
#6565=CARTESIAN_POINT('Ctrl Pts',(28.5067626169521,56.6319118940954,74.1822324995112)) ;
#6566=CARTESIAN_POINT('Ctrl Pts',(28.5155794125353,56.6127538456679,74.1747702096408)) ;
#6567=CARTESIAN_POINT('Ctrl Pts',(28.6312140508663,56.3614909032359,74.0769002769485)) ;
#6568=CARTESIAN_POINT('Ctrl Pts',(28.7440516725572,56.1103350670436,73.9756114424237)) ;
#6569=CARTESIAN_POINT('Ctrl Pts',(28.8538256281834,55.8590202585562,73.8711333467298)) ;
#6570=CARTESIAN_POINT('Ctrl Pts',(28.8607788186558,55.8431017310512,73.8645156012417)) ;
#6571=CARTESIAN_POINT('Ctrl Pts',(28.8677195431166,55.8271830724928,73.857885278296)) ;
#6572=CARTESIAN_POINT('Ctrl Pts',(28.8746477921954,55.8112643008986,73.8512423838609)) ;
#6573=CARTESIAN_POINT('Ctrl Pts',(28.9854377430074,55.5567064895583,73.7450155523287)) ;
#6574=CARTESIAN_POINT('Ctrl Pts',(29.0930908521726,55.3019957844142,73.6355216404124)) ;
#6575=CARTESIAN_POINT('Ctrl Pts',(29.1975705510464,55.0471908391174,73.5227738207595)) ;
#6576=CARTESIAN_POINT('Ctrl Pts',(29.202774724961,55.034498906963,73.5171578085745)) ;
#6577=CARTESIAN_POINT('Ctrl Pts',(29.2079709717293,55.0218058655745,73.5115337104615)) ;
#6578=CARTESIAN_POINT('Ctrl Pts',(29.2131592267093,55.0091118266697,73.5059016032595)) ;
#6579=CARTESIAN_POINT('Ctrl Pts',(29.3186566481837,54.7509925981975,73.3913789382059)) ;
#6580=CARTESIAN_POINT('Ctrl Pts',(29.420791245856,54.4926055130969,73.2736094403093)) ;
#6581=CARTESIAN_POINT('Ctrl Pts',(29.5191454608939,54.2345762733043,73.1530981676337)) ;
#6582=CARTESIAN_POINT('Ctrl Pts',(29.5227356562035,54.2251575070004,73.1486991796925)) ;
#6583=CARTESIAN_POINT('Ctrl Pts',(29.5263211032666,54.2157389752755,73.144296194541)) ;
#6584=CARTESIAN_POINT('Ctrl Pts',(29.5299017952159,54.2063206495465,73.139889221293)) ;
#6585=CARTESIAN_POINT('Ctrl Pts',(29.6292306159036,53.9450551732692,73.0176392590708)) ;
#6586=CARTESIAN_POINT('Ctrl Pts',(29.7248575150048,53.6840579939705,72.8923709682529)) ;
#6587=CARTESIAN_POINT('Ctrl Pts',(29.8165233971548,53.4230444575825,72.76444089322)) ;
#6588=CARTESIAN_POINT('Ctrl Pts',(29.8186881695431,53.4168803877749,72.7614197092465)) ;
#6589=CARTESIAN_POINT('Ctrl Pts',(29.8208507289346,53.4107163827,72.758397056665)) ;
#6590=CARTESIAN_POINT('Ctrl Pts',(29.8230110750717,53.4045524432164,72.7553729359249)) ;
#6591=CARTESIAN_POINT('Ctrl Pts',(29.9156335453573,53.1402803009608,72.6257170772735)) ;
#6592=CARTESIAN_POINT('Ctrl Pts',(30.0042142732511,52.8760533725719,72.493325654808)) ;
#6593=CARTESIAN_POINT('Ctrl Pts',(30.0887477381456,52.6118787196959,72.3581998849054)) ;
#6594=CARTESIAN_POINT('Ctrl Pts',(30.175136346897,52.3419065760271,72.2201086889169)) ;
#6595=CARTESIAN_POINT('Ctrl Pts',(30.2572393512457,52.0715787920594,72.0792347687965)) ;
#6596=CARTESIAN_POINT('Ctrl Pts',(30.3348641568369,51.8011908422986,71.9358954676151)) ;
#6597=CARTESIAN_POINT('Ctrl Pts',(30.3349616095944,51.8008513882913,71.9357155146984)) ;
#6598=CARTESIAN_POINT('Ctrl Pts',(30.3350590552918,51.8005119341973,71.9355355579006)) ;
#6599=CARTESIAN_POINT('Ctrl Pts',(30.3351564939286,51.8001724800173,71.9353555972221)) ;
#6600=CARTESIAN_POINT('Ctrl Pts',(30.4118392607038,51.5330270582815,71.7937292035196)) ;
#6601=CARTESIAN_POINT('Ctrl Pts',(30.4842968674352,51.2655853544539,71.6493926137567)) ;
#6602=CARTESIAN_POINT('Ctrl Pts',(30.552072420951,50.998401550286,71.503248573748)) ;
#6603=CARTESIAN_POINT('Ctrl Pts',(30.5529834678514,50.9948100344075,71.5012840885058)) ;
#6604=CARTESIAN_POINT('Ctrl Pts',(30.5538936734284,50.991218547496,71.499319267114)) ;
#6605=CARTESIAN_POINT('Ctrl Pts',(30.5548030365843,50.9876270907846,71.4973541116952)) ;
#6606=CARTESIAN_POINT('Ctrl Pts',(30.6216299293917,50.723699647588,71.3529396061481)) ;
#6607=CARTESIAN_POINT('Ctrl Pts',(30.6839607896437,50.4599498020534,71.2066569873818)) ;
#6608=CARTESIAN_POINT('Ctrl Pts',(30.7418017309264,50.1963788513667,71.0585096581505)) ;
#6609=CARTESIAN_POINT('Ctrl Pts',(30.7432971955163,50.1895642834339,71.0546793421142)) ;
#6610=CARTESIAN_POINT('Ctrl Pts',(30.7447896214764,50.1827500045963,71.0508478748386)) ;
#6611=CARTESIAN_POINT('Ctrl Pts',(30.746279010706,50.175936008737,71.0470152531297)) ;
#6612=CARTESIAN_POINT('Ctrl Pts',(30.8031794696593,49.9156148757636,70.9005942035517)) ;
#6613=CARTESIAN_POINT('Ctrl Pts',(30.8555919805957,49.6552611188171,70.7526177854089)) ;
#6614=CARTESIAN_POINT('Ctrl Pts',(30.9035138752949,49.3948957256021,70.6031422004369)) ;
#6615=CARTESIAN_POINT('Ctrl Pts',(30.90537060004,49.3848079176934,70.5973507971724)) ;
#6616=CARTESIAN_POINT('Ctrl Pts',(30.9072205375093,49.3747203101763,70.5915572664575)) ;
#6617=CARTESIAN_POINT('Ctrl Pts',(30.9090636830444,49.3646329259559,70.5857616238384)) ;
#6618=CARTESIAN_POINT('Ctrl Pts',(30.9560371523614,49.1075509841657,70.4380568248653)) ;
#6619=CARTESIAN_POINT('Ctrl Pts',(30.9986538215556,48.8504690628026,70.2887840081728)) ;
#6620=CARTESIAN_POINT('Ctrl Pts',(31.0367725700753,48.5931578990174,70.1383929388844)) ;
#6621=CARTESIAN_POINT('Ctrl Pts',(31.0387501111437,48.5798089981879,70.1305908853705)) ;
#6622=CARTESIAN_POINT('Ctrl Pts',(31.040715607705,48.5664590689811,70.1227855817124)) ;
#6623=CARTESIAN_POINT('Ctrl Pts',(31.0426690346055,48.553108105864,70.1149771058549)) ;
#6624=CARTESIAN_POINT('Ctrl Pts',(31.0798470008467,48.2990102146502,69.9663648123762)) ;
#6625=CARTESIAN_POINT('Ctrl Pts',(31.1126813517942,48.0446012919295,69.8165063124975)) ;
#6626=CARTESIAN_POINT('Ctrl Pts',(31.1410716961609,47.7903648312086,69.6657693769311)) ;
#6627=CARTESIAN_POINT('Ctrl Pts',(31.142923648441,47.7737805380755,69.6559365405302)) ;
#6628=CARTESIAN_POINT('Ctrl Pts',(31.1447567589066,47.7571963611374,69.6460996001179)) ;
#6629=CARTESIAN_POINT('Ctrl Pts',(31.1465710087748,47.7406123516808,69.6362586086441)) ;
#6630=CARTESIAN_POINT('Ctrl Pts',(31.1740304610611,47.4896062337396,69.4873109688723)) ;
#6631=CARTESIAN_POINT('Ctrl Pts',(31.1971065359107,47.2387261489801,69.3378286203306)) ;
#6632=CARTESIAN_POINT('Ctrl Pts',(31.2158269587204,46.9878897404752,69.1877652509507)) ;
#6633=CARTESIAN_POINT('Ctrl Pts',(31.217300311963,46.9681481652134,69.1759548151439)) ;
#6634=CARTESIAN_POINT('Ctrl Pts',(31.218746628802,46.9484074501539,69.1641411312535)) ;
#6635=CARTESIAN_POINT('Ctrl Pts',(31.2201659213531,46.9286675886395,69.152324196894)) ;
#6636=CARTESIAN_POINT('Ctrl Pts',(31.2379716343071,46.6810214584577,69.0040750279415)) ;
#6637=CARTESIAN_POINT('Ctrl Pts',(31.2515255162978,46.4334531760662,68.8552127523791)) ;
#6638=CARTESIAN_POINT('Ctrl Pts',(31.2607899566468,46.1857600468478,68.70614811867)) ;
#6639=CARTESIAN_POINT('Ctrl Pts',(31.2616415494885,46.1629919477682,68.6924460092887)) ;
#6640=CARTESIAN_POINT('Ctrl Pts',(31.2624569163218,46.1402223084086,68.678741898586)) ;
#6641=CARTESIAN_POINT('Ctrl Pts',(31.2632360228334,46.1174510138863,68.6650361315705)) ;
#6642=CARTESIAN_POINT('Ctrl Pts',(31.271608391925,45.8727480373429,68.517752366864)) ;
#6643=CARTESIAN_POINT('Ctrl Pts',(31.2758073873136,45.6279743432133,68.3701949493187)) ;
#6644=CARTESIAN_POINT('Ctrl Pts',(31.2758081909614,45.3830610445957,68.222429730099)) ;
#6645=CARTESIAN_POINT('',(57.4106193181313,48.5844537758935,76.7989233032516)) ;
#6646=CARTESIAN_POINT('Ctrl Pts',(51.7933248065259,45.3830586252741,68.2224337400008)) ;
#6647=CARTESIAN_POINT('Ctrl Pts',(52.308018473855,45.4231928758842,68.3103779261485)) ;
#6648=CARTESIAN_POINT('Ctrl Pts',(52.8090405407003,45.4870033972977,68.4552855869039)) ;
#6649=CARTESIAN_POINT('Ctrl Pts',(53.7748388026689,45.6539797372435,68.8542815132844)) ;
#6650=CARTESIAN_POINT('Ctrl Pts',(54.2353699749147,45.7573388893141,69.1091189365817)) ;
#6651=CARTESIAN_POINT('Ctrl Pts',(55.4095055664222,46.0833507061677,69.9408962356853)) ;
#6652=CARTESIAN_POINT('Ctrl Pts',(56.0396012667916,46.333687722769,70.6083832653474)) ;
#6653=CARTESIAN_POINT('Ctrl Pts',(57.0466870536474,46.9107591797132,72.1931483430176)) ;
#6654=CARTESIAN_POINT('Ctrl Pts',(57.3887715545277,47.2383195349501,73.1130504687389)) ;
#6655=CARTESIAN_POINT('Ctrl Pts',(57.673423309298,47.9083523080808,74.9787376424982)) ;
#6656=CARTESIAN_POINT('Ctrl Pts',(57.6305961076901,48.2450338483643,75.907165158477)) ;
#6657=CARTESIAN_POINT('Ctrl Pts',(57.4106193181313,48.5844537758935,76.7989233032516)) ;
#6658=CARTESIAN_POINT('',(57.3984019004021,48.6029307720944,76.8474073371282)) ;
#6659=CARTESIAN_POINT('Origin',(92.1683318818475,48.3646139793373,85.6889926784978)) ;
#6660=CARTESIAN_POINT('',(49.1121349038258,55.0677871747466,92.0526694236409)) ;
#6661=CARTESIAN_POINT('Ctrl Pts',(57.3984019004021,48.6029307720944,76.8474073371282)) ;
#6662=CARTESIAN_POINT('Ctrl Pts',(57.2766816661225,48.785356686239,77.3258247136573)) ;
#6663=CARTESIAN_POINT('Ctrl Pts',(57.1415855268086,48.9676174488035,77.8006383925237)) ;
#6664=CARTESIAN_POINT('Ctrl Pts',(56.6987584006366,49.5650439193917,79.3570143033935)) ;
#6665=CARTESIAN_POINT('Ctrl Pts',(56.1142160449124,50.16247038998,80.8658920565512)) ;
#6666=CARTESIAN_POINT('Ctrl Pts',(55.5296736891883,50.7598968605682,82.3747698097088)) ;
#6667=CARTESIAN_POINT('Ctrl Pts',(54.8084032131872,51.3573233311564,83.8232761921796)) ;
#6668=CARTESIAN_POINT('Ctrl Pts',(54.0871327371861,51.9547498017447,85.2717825746505)) ;
#6669=CARTESIAN_POINT('Ctrl Pts',(53.2352877662965,52.5521762723329,86.6475594407083)) ;
#6670=CARTESIAN_POINT('Ctrl Pts',(52.3834427954069,53.1496027429211,88.023336306766)) ;
#6671=CARTESIAN_POINT('Ctrl Pts',(51.4082909705684,53.7470292135094,89.3146460132748)) ;
#6672=CARTESIAN_POINT('Ctrl Pts',(50.4331391457298,54.3444556840976,90.6059557197835)) ;
#6673=CARTESIAN_POINT('Ctrl Pts',(49.3430001184831,54.9418821546858,91.8017812676303)) ;
#6674=CARTESIAN_POINT('Ctrl Pts',(49.2281522354556,55.0048219850164,91.9277633939534)) ;
#6675=CARTESIAN_POINT('Ctrl Pts',(49.1121349038258,55.0677871747466,92.0526694236409)) ;
#6676=CARTESIAN_POINT('',(49.0780136113479,55.0862551252693,92.0892167113166)) ;
#6677=CARTESIAN_POINT('Origin',(75.4923509619182,55.5526174178892,116.574769538313)) ;
#6678=CARTESIAN_POINT('Ctrl Pts',(49.0780136113479,55.0862551252693,92.0892167113166)) ;
#6679=CARTESIAN_POINT('Ctrl Pts',(48.7067240185058,55.2861476427455,92.4829396223812)) ;
#6680=CARTESIAN_POINT('Ctrl Pts',(48.2907363800878,55.4856144064204,92.8325865509095)) ;
#6681=CARTESIAN_POINT('Ctrl Pts',(47.3532876815545,55.8948727823201,93.4506135013496)) ;
#6682=CARTESIAN_POINT('Ctrl Pts',(46.8292280164247,56.1030297966033,93.709526588545)) ;
#6683=CARTESIAN_POINT('Ctrl Pts',(45.3720572721415,56.6395229540349,94.2145561773987)) ;
#6684=CARTESIAN_POINT('Ctrl Pts',(44.4045376611851,56.955307721454,94.3415217577794)) ;
#6685=CARTESIAN_POINT('Ctrl Pts',(42.541193176401,57.5027528833962,94.1944856565899)) ;
#6686=CARTESIAN_POINT('Ctrl Pts',(41.6597611935,57.735639297119,93.9520695669813)) ;
#6687=CARTESIAN_POINT('Ctrl Pts',(40.24270309089,58.0583687617077,93.2401772744575)) ;
#6688=CARTESIAN_POINT('Ctrl Pts',(39.6843220177388,58.1679507457141,92.8513543260053)) ;
#6689=CARTESIAN_POINT('Ctrl Pts',(38.7635710417162,58.3023925284601,91.9849192838713)) ;
#6690=CARTESIAN_POINT('Ctrl Pts',(38.3891340647941,58.3364158763933,91.5324440811863)) ;
#6691=CARTESIAN_POINT('Ctrl Pts',(38.075012827077,58.3353824278239,91.0374682134905)) ;
#6692=CARTESIAN_POINT('Ctrl Pts',(58.4776880737725,45.3830585852922,68.1224336317086)) ;
#6693=CARTESIAN_POINT('Ctrl Pts',(58.482311357954,45.9804850758286,69.7405813455768)) ;
#6694=CARTESIAN_POINT('Ctrl Pts',(58.3376110801056,46.5779115664505,71.3522529089681)) ;
#6695=CARTESIAN_POINT('Ctrl Pts',(58.1929108071096,47.1753380370388,72.9639244183148)) ;
#6696=CARTESIAN_POINT('Ctrl Pts',(57.9001215138071,47.772764507627,74.555369564329)) ;
#6697=CARTESIAN_POINT('Ctrl Pts',(57.6073322205045,48.3701909782153,76.1468147103432)) ;
#6698=CARTESIAN_POINT('Ctrl Pts',(57.1689518819114,48.9676174488035,77.704455844167)) ;
#6699=CARTESIAN_POINT('Ctrl Pts',(56.7305715433182,49.5650439193917,79.2620969779907)) ;
#6700=CARTESIAN_POINT('Ctrl Pts',(56.1503402659147,50.16247038998,80.772644854679)) ;
#6701=CARTESIAN_POINT('Ctrl Pts',(55.5701089885112,50.7598968605682,82.2831927313673)) ;
#6702=CARTESIAN_POINT('Ctrl Pts',(54.8529771009725,51.3573233311564,83.7337598890405)) ;
#6703=CARTESIAN_POINT('Ctrl Pts',(54.1358452134337,51.9547498017447,85.1843270467136)) ;
#6704=CARTESIAN_POINT('Ctrl Pts',(53.2879310321705,52.5521762723329,86.5625377578378)) ;
#6705=CARTESIAN_POINT('Ctrl Pts',(52.4400168509074,53.1496027429211,87.9407484689621)) ;
#6706=CARTESIAN_POINT('Ctrl Pts',(51.4685544807482,53.7470292135094,89.2348443256936)) ;
#6707=CARTESIAN_POINT('Ctrl Pts',(50.497092110589,54.3444556840976,90.5289401824251)) ;
#6708=CARTESIAN_POINT('Ctrl Pts',(49.4103697259481,54.9418821546858,91.7278804151995)) ;
#6709=CARTESIAN_POINT('Ctrl Pts',(48.3236473413072,55.5393086252741,92.9268206479739)) ;
#6710=CARTESIAN_POINT('Ctrl Pts',(47.1309364744028,56.1367350958623,94.0203763214597)) ;
#6711=CARTESIAN_POINT('Ctrl Pts',(45.9382256074983,56.7341615664505,95.1139319949454)) ;
#6712=CARTESIAN_POINT('Ctrl Pts',(44.6497020469088,57.3315880370388,96.0927732777132)) ;
#6713=CARTESIAN_POINT('Ctrl Pts',(43.5159923066831,57.8572347768351,96.9540085165172)) ;
#6714=CARTESIAN_POINT('Ctrl Pts',(42.3160773566393,58.3831186720347,97.7203165644338)) ;
#6715=CARTESIAN_POINT('Ctrl Pts',(30.9776880154505,45.3830585852922,68.1224337167953)) ;
#6716=CARTESIAN_POINT('Ctrl Pts',(30.9823112956982,45.9804850758286,68.4691796548923)) ;
#6717=CARTESIAN_POINT('Ctrl Pts',(30.954921173919,46.5779115664506,68.8148730183461)) ;
#6718=CARTESIAN_POINT('Ctrl Pts',(30.9275310530584,47.1753380370388,69.1605663702075)) ;
#6719=CARTESIAN_POINT('Ctrl Pts',(30.8683612151709,47.772764507627,69.5022578136567)) ;
#6720=CARTESIAN_POINT('Ctrl Pts',(30.8091913772834,48.3701909782152,69.8439492571058)) ;
#6721=CARTESIAN_POINT('Ctrl Pts',(30.7187466385633,48.9676174488035,70.1787236012241)) ;
#6722=CARTESIAN_POINT('Ctrl Pts',(30.6283018998432,49.5650439193917,70.5134979453425)) ;
#6723=CARTESIAN_POINT('Ctrl Pts',(30.5073539029114,50.16247038998,70.838499013464)) ;
#6724=CARTESIAN_POINT('Ctrl Pts',(30.3864059059795,50.7598968605682,71.1635000815856)) ;
#6725=CARTESIAN_POINT('Ctrl Pts',(30.2359865365006,51.3573233311564,71.4759550791893)) ;
#6726=CARTESIAN_POINT('Ctrl Pts',(30.0855671670217,51.9547498017447,71.7884100767931)) ;
#6727=CARTESIAN_POINT('Ctrl Pts',(29.9069597500198,52.5521762723329,72.085653248008)) ;
#6728=CARTESIAN_POINT('Ctrl Pts',(29.7283523330179,53.1496027429211,72.3828964192229)) ;
#6729=CARTESIAN_POINT('Ctrl Pts',(29.5230806839997,53.7470292135094,72.6623917901172)) ;
#6730=CARTESIAN_POINT('Ctrl Pts',(29.3178090349815,54.3444556840976,72.9418871610115)) ;
#6731=CARTESIAN_POINT('Ctrl Pts',(29.0876244592796,54.9418821546858,73.2012501756279)) ;
#6732=CARTESIAN_POINT('Ctrl Pts',(28.8574398835777,55.5393086252741,73.4606131902444)) ;
#6733=CARTESIAN_POINT('Ctrl Pts',(28.6043062348312,56.1367350958623,73.6976310547911)) ;
#6734=CARTESIAN_POINT('Ctrl Pts',(28.3511725860848,56.7341615664505,73.9346489193378)) ;
#6735=CARTESIAN_POINT('Ctrl Pts',(28.0772495113324,57.3315880370388,74.1472994809647)) ;
#6736=CARTESIAN_POINT('Ctrl Pts',(27.8362378081571,57.857234776835,74.3344004547882)) ;
#6737=CARTESIAN_POINT('Ctrl Pts',(27.5808257495764,58.3831186720347,74.5013079016107)) ;
#6738=CARTESIAN_POINT('',(27.7390441888434,58.3830537363181,74.7506193750977)) ;
#6739=CARTESIAN_POINT('Ctrl Pts',(31.2729697953901,45.3830674541112,68.1224191093439)) ;
#6740=CARTESIAN_POINT('Ctrl Pts',(31.2731002040288,45.3999249614352,68.1325854719125)) ;
#6741=CARTESIAN_POINT('Ctrl Pts',(31.2732122621832,45.4170195560987,68.1428947122456)) ;
#6742=CARTESIAN_POINT('Ctrl Pts',(31.2733941703955,45.4509660823354,68.1633665015427)) ;
#6743=CARTESIAN_POINT('Ctrl Pts',(31.2734649447084,45.467937485669,68.1736011010902)) ;
#6744=CARTESIAN_POINT('Ctrl Pts',(31.2736167856114,45.5188462146266,68.2043008651703)) ;
#6745=CARTESIAN_POINT('Ctrl Pts',(31.2736373705305,45.5527780591987,68.224761995133)) ;
#6746=CARTESIAN_POINT('Ctrl Pts',(31.2734576427624,45.6545524513432,68.2861280505301)) ;
#6747=CARTESIAN_POINT('Ctrl Pts',(31.2730158320587,45.7223738576057,68.3270156411209)) ;
#6748=CARTESIAN_POINT('Ctrl Pts',(31.2712928003503,45.8755455989765,68.4193346417184)) ;
#6749=CARTESIAN_POINT('Ctrl Pts',(31.2698234610056,45.9608834226846,68.4707523146004)) ;
#6750=CARTESIAN_POINT('Ctrl Pts',(31.2666852108686,46.0963466756237,68.5523307651114)) ;
#6751=CARTESIAN_POINT('Ctrl Pts',(31.2653472956213,46.1464973799214,68.5825318896186)) ;
#6752=CARTESIAN_POINT('Ctrl Pts',(31.2568446873907,46.4282028809672,68.7521513571258)) ;
#6753=CARTESIAN_POINT('Ctrl Pts',(31.2461154561705,46.6594344485716,68.8912820844549)) ;
#6754=CARTESIAN_POINT('Ctrl Pts',(31.2292419752858,46.9296827699017,69.053312093353)) ;
#6755=CARTESIAN_POINT('Ctrl Pts',(31.2266938785506,46.9687950424149,69.0767488265404)) ;
#6756=CARTESIAN_POINT('Ctrl Pts',(31.2076132849116,47.2499758749323,69.2451407456555)) ;
#6757=CARTESIAN_POINT('Ctrl Pts',(31.187138450914,47.4918541916759,69.3894818460527)) ;
#6758=CARTESIAN_POINT('Ctrl Pts',(31.134152559873,48.0143150857869,69.7001535512841)) ;
#6759=CARTESIAN_POINT('Ctrl Pts',(31.1002399082149,48.2952954282261,69.8661264207476)) ;
#6760=CARTESIAN_POINT('Ctrl Pts',(31.0586022138039,48.5931204307081,70.0407394220474)) ;
#6761=CARTESIAN_POINT('Ctrl Pts',(31.0562056645437,48.6101204742725,70.0507024497919)) ;
#6762=CARTESIAN_POINT('Ctrl Pts',(31.0162768638686,48.891036215033,70.2152669033389)) ;
#6763=CARTESIAN_POINT('Ctrl Pts',(30.97399601099,49.1549226796806,70.3688528007291)) ;
#6764=CARTESIAN_POINT('Ctrl Pts',(30.926014393781,49.4249376060053,70.5243549547346)) ;
#6765=CARTESIAN_POINT('Ctrl Pts',(30.9249701498923,49.4308011237537,70.5277310753253)) ;
#6766=CARTESIAN_POINT('Ctrl Pts',(30.8757301114589,49.7066812295574,70.6865457989593)) ;
#6767=CARTESIAN_POINT('Ctrl Pts',(30.8226320620207,49.9768666464287,70.8406088060635)) ;
#6768=CARTESIAN_POINT('Ctrl Pts',(30.763508756557,50.2527043291673,70.996102876115)) ;
#6769=CARTESIAN_POINT('Ctrl Pts',(30.7623588146578,50.2580605419639,70.9991215703048)) ;
#6770=CARTESIAN_POINT('Ctrl Pts',(30.7041887220664,50.5285623062296,71.1515381204764)) ;
#6771=CARTESIAN_POINT('Ctrl Pts',(30.6425647115896,50.794089282034,71.2992229922643)) ;
#6772=CARTESIAN_POINT('Ctrl Pts',(30.572121971017,51.0767673302899,71.4543847718665)) ;
#6773=CARTESIAN_POINT('Ctrl Pts',(30.5679317898639,51.0935097128498,71.4635669735966)) ;
#6774=CARTESIAN_POINT('Ctrl Pts',(30.5281873953612,51.2516332986662,71.5502158138466)) ;
#6775=CARTESIAN_POINT('Ctrl Pts',(30.4913068609656,51.3931664825954,71.6272604837886)) ;
#6776=CARTESIAN_POINT('Ctrl Pts',(30.4227007802738,51.6479675595822,71.764730378545)) ;
#6777=CARTESIAN_POINT('Ctrl Pts',(30.3914137616775,51.7612319406863,71.8254116450958)) ;
#6778=CARTESIAN_POINT('Ctrl Pts',(30.3513694705723,51.9026374456283,71.9006379050749)) ;
#6779=CARTESIAN_POINT('Ctrl Pts',(30.3433428020212,51.9308091085123,71.9155985690478)) ;
#6780=CARTESIAN_POINT('Ctrl Pts',(30.254218376761,52.2417252333148,72.0804209027061)) ;
#6781=CARTESIAN_POINT('Ctrl Pts',(30.1682727980748,52.524119549272,72.2276169079598)) ;
#6782=CARTESIAN_POINT('Ctrl Pts',(30.0033152730407,53.0381974993267,72.4899907921184)) ;
#6783=CARTESIAN_POINT('Ctrl Pts',(29.9259031671205,53.2697333986821,72.6060846287223)) ;
#6784=CARTESIAN_POINT('Ctrl Pts',(29.8276482002984,53.5522259966914,72.7451927295007)) ;
#6785=CARTESIAN_POINT('Ctrl Pts',(29.8097755308276,53.6031771340237,72.7701819457636)) ;
#6786=CARTESIAN_POINT('Ctrl Pts',(29.7138859105828,53.8742457620993,72.9025930757515)) ;
#6787=CARTESIAN_POINT('Ctrl Pts',(29.6332371813762,54.0945463050599,73.0081686491436)) ;
#6788=CARTESIAN_POINT('Ctrl Pts',(29.526309645954,54.3774106831913,73.1409687184945)) ;
#6789=CARTESIAN_POINT('Ctrl Pts',(29.5024838913393,54.4398806254194,73.1701248283594)) ;
#6790=CARTESIAN_POINT('Ctrl Pts',(29.398005894515,54.7114321392953,73.2961024622914)) ;
#6791=CARTESIAN_POINT('Ctrl Pts',(29.3151050184895,54.9205828276713,73.3912609624358)) ;
#6792=CARTESIAN_POINT('Ctrl Pts',(29.200017146324,55.203368432956,73.5170824558052)) ;
#6793=CARTESIAN_POINT('Ctrl Pts',(29.1696780956447,55.2772338818111,73.5496854174052)) ;
#6794=CARTESIAN_POINT('Ctrl Pts',(29.0572712397692,55.5485088102172,73.6684197231037)) ;
#6795=CARTESIAN_POINT('Ctrl Pts',(28.9735572714829,55.7457837763595,73.752890529924)) ;
#6796=CARTESIAN_POINT('Ctrl Pts',(28.85093682095,56.0282588904742,73.8710838626765)) ;
#6797=CARTESIAN_POINT('Ctrl Pts',(28.8135798522358,56.1134884206095,73.9063851924763)) ;
#6798=CARTESIAN_POINT('Ctrl Pts',(28.6936894265498,56.3844426291116,74.0174544380719)) ;
#6799=CARTESIAN_POINT('Ctrl Pts',(28.6099617745652,56.5701302611217,74.0917343757168)) ;
#6800=CARTESIAN_POINT('Ctrl Pts',(28.4801870114973,56.8526653482997,74.20196576487)) ;
#6801=CARTESIAN_POINT('Ctrl Pts',(28.4352967717226,56.9494716030796,74.2392362716071)) ;
#6802=CARTESIAN_POINT('Ctrl Pts',(28.3084560784753,57.220441360115,74.3421652352563)) ;
#6803=CARTESIAN_POINT('Ctrl Pts',(28.2255259009952,57.3946576755337,74.4067251242961)) ;
#6804=CARTESIAN_POINT('Ctrl Pts',(28.0888919857564,57.6774250653642,74.5087254230024)) ;
#6805=CARTESIAN_POINT('Ctrl Pts',(28.0359724099055,57.7859396412659,74.5472038149203)) ;
#6806=CARTESIAN_POINT('Ctrl Pts',(27.9692360255816,57.9216227418851,74.5944549811629)) ;
#6807=CARTESIAN_POINT('Ctrl Pts',(27.9558731511316,57.9487278912592,74.603853248453)) ;
#6808=CARTESIAN_POINT('Ctrl Pts',(27.9089544007098,58.0436810159811,74.6366316934481)) ;
#6809=CARTESIAN_POINT('Ctrl Pts',(27.8752324837114,58.1115399743052,74.6597974493204)) ;
#6810=CARTESIAN_POINT('Ctrl Pts',(27.8243671241468,58.2133484522819,74.6941541076358)) ;
#6811=CARTESIAN_POINT('Ctrl Pts',(27.8073663790787,58.2472850649056,74.7055400425132)) ;
#6812=CARTESIAN_POINT('Ctrl Pts',(27.7817951862796,58.2981973836578,74.722520540854)) ;
#6813=CARTESIAN_POINT('Ctrl Pts',(27.7732597760152,58.3151693899102,74.7281643060626)) ;
#6814=CARTESIAN_POINT('Ctrl Pts',(27.762384280287,58.3367668565644,74.7353246686243)) ;
#6815=CARTESIAN_POINT('Ctrl Pts',(27.7600504741546,58.3413999128692,74.736859442133)) ;
#6816=CARTESIAN_POINT('Ctrl Pts',(27.7514785817235,58.3584108602027,74.742489946245)) ;
#6817=CARTESIAN_POINT('Ctrl Pts',(27.7452310605373,58.3707975233385,74.7465807676633)) ;
#6818=CARTESIAN_POINT('Ctrl Pts',(27.7390451836026,58.3830508753326,74.7506187222499)) ;
#6819=CARTESIAN_POINT('',(38.075012827077,58.3831162793798,91.0374682134904)) ;
#6820=CARTESIAN_POINT('Ctrl Pts',(27.739058487419,58.3830900980199,74.7506102954531)) ;
#6821=CARTESIAN_POINT('Ctrl Pts',(29.4617175445255,58.3831052593851,77.4650866159089)) ;
#6822=CARTESIAN_POINT('Ctrl Pts',(31.1843766016598,58.3831073991803,80.1795629364082)) ;
#6823=CARTESIAN_POINT('Ctrl Pts',(34.6296947148817,58.3831134572106,85.6085155757581)) ;
#6824=CARTESIAN_POINT('Ctrl Pts',(36.3523537709793,58.383115023513,88.3229918946244)) ;
#6825=CARTESIAN_POINT('Ctrl Pts',(38.0750128270769,58.3831162793798,91.0374682134904)) ;
#6826=CARTESIAN_POINT('',(49.11218721881,55.104724217109,92.0527180565764)) ;
#6827=CARTESIAN_POINT('Ctrl Pts',(38.075012827077,58.3831162793798,91.0374682134904)) ;
#6828=CARTESIAN_POINT('Ctrl Pts',(38.3910170362888,58.3831165097557,91.535411169487)) ;
#6829=CARTESIAN_POINT('Ctrl Pts',(38.7680285100977,58.3477204189414,91.990287868787)) ;
#6830=CARTESIAN_POINT('Ctrl Pts',(39.6959726062055,58.2097833704152,92.8609217685079)) ;
#6831=CARTESIAN_POINT('Ctrl Pts',(40.2592080825518,58.0979491851445,93.251035058612)) ;
#6832=CARTESIAN_POINT('Ctrl Pts',(41.6832452702688,57.7707078254697,93.9602870316529)) ;
#6833=CARTESIAN_POINT('Ctrl Pts',(42.5660592155094,57.5360202457533,94.199694127608)) ;
#6834=CARTESIAN_POINT('Ctrl Pts',(44.4307136974944,56.9856758817168,94.3399656139212)) ;
#6835=CARTESIAN_POINT('Ctrl Pts',(45.3981702829227,56.6687344805943,94.2093431307212)) ;
#6836=CARTESIAN_POINT('Ctrl Pts',(46.8577625330414,56.1294192803767,93.6971962023311)) ;
#6837=CARTESIAN_POINT('Ctrl Pts',(47.384386064077,55.9194276565171,93.4339192562471)) ;
#6838=CARTESIAN_POINT('Ctrl Pts',(48.3247863893035,55.5068628236253,92.8063316588796)) ;
#6839=CARTESIAN_POINT('Ctrl Pts',(48.7412751267391,55.3059550653476,92.4517122776391)) ;
#6840=CARTESIAN_POINT('Ctrl Pts',(49.11218721881,55.104724217109,92.0527180565764)) ;
#6841=CARTESIAN_POINT('',(57.3984711260663,48.6398835186857,76.8474249390433)) ;
#6842=CARTESIAN_POINT('Ctrl Pts',(57.3984711260663,48.6398835186857,76.8474249390432)) ;
#6843=CARTESIAN_POINT('Ctrl Pts',(57.2891432146506,48.8038201453524,77.2773950439918)) ;
#6844=CARTESIAN_POINT('Ctrl Pts',(57.1689518258159,48.9676174488035,77.7044558282064)) ;
#6845=CARTESIAN_POINT('Ctrl Pts',(56.7305714879606,49.5650439193917,79.2620969594367)) ;
#6846=CARTESIAN_POINT('Ctrl Pts',(56.1503402115311,50.16247038998,80.7726448336107)) ;
#6847=CARTESIAN_POINT('Ctrl Pts',(55.5701089351017,50.7598968605682,82.2831927077847)) ;
#6848=CARTESIAN_POINT('Ctrl Pts',(54.8529770487648,51.3573233311564,83.7337598630442)) ;
#6849=CARTESIAN_POINT('Ctrl Pts',(54.1358451624279,51.9547498017447,85.1843270183036)) ;
#6850=CARTESIAN_POINT('Ctrl Pts',(53.2879309825842,52.5521762723329,86.5625377271353)) ;
#6851=CARTESIAN_POINT('Ctrl Pts',(52.4400168027405,53.1496027429211,87.9407484359671)) ;
#6852=CARTESIAN_POINT('Ctrl Pts',(51.4685544342063,53.7470292135094,89.2348442905468)) ;
#6853=CARTESIAN_POINT('Ctrl Pts',(50.4970920656721,54.3444556840976,90.5289401451265)) ;
#6854=CARTESIAN_POINT('Ctrl Pts',(49.4103696828477,54.9418821546858,91.7278803759083)) ;
#6855=CARTESIAN_POINT('Ctrl Pts',(49.262301577525,55.0232827101246,91.8912383881963)) ;
#6856=CARTESIAN_POINT('Ctrl Pts',(49.11218721881,55.104724217109,92.0527180565764)) ;
#6857=CARTESIAN_POINT('Ctrl Pts',(57.3984711260663,48.6398835186857,76.8474249390433)) ;
#6858=CARTESIAN_POINT('Ctrl Pts',(57.5318809087092,48.4398362531007,76.3227444846068)) ;
#6859=CARTESIAN_POINT('Ctrl Pts',(57.6040805147783,48.2402511664186,75.7839347717915)) ;
#6860=CARTESIAN_POINT('Ctrl Pts',(57.6232176241361,47.8311033708304,74.6615809415638)) ;
#6861=CARTESIAN_POINT('Ctrl Pts',(57.5609538539119,47.6231195575042,74.0809852902915)) ;
#6862=CARTESIAN_POINT('Ctrl Pts',(57.2066131255233,47.0862679673289,72.5806485964983)) ;
#6863=CARTESIAN_POINT('Ctrl Pts',(56.7952723804051,46.7703269230099,71.6955878783151)) ;
#6864=CARTESIAN_POINT('Ctrl Pts',(55.6718207466244,46.2216256025066,70.200388721669)) ;
#6865=CARTESIAN_POINT('Ctrl Pts',(54.9943545947592,45.987905739686,69.5859906898853)) ;
#6866=CARTESIAN_POINT('Ctrl Pts',(53.6339893980261,45.6640068127921,68.7717169071534)) ;
#6867=CARTESIAN_POINT('Ctrl Pts',(53.0073921260216,45.5539383581279,68.5091118556871)) ;
#6868=CARTESIAN_POINT('Ctrl Pts',(51.7834240894348,45.4179657700952,68.1961600284618)) ;
#6869=CARTESIAN_POINT('Ctrl Pts',(51.2006845491435,45.3830585853871,68.1224336562375)) ;
#6870=CARTESIAN_POINT('Ctrl Pts',(50.6143411942707,45.3830586252741,68.1224337400008)) ;
#6871=CARTESIAN_POINT('Origin',(50.6143421942707,45.3822493559848,75.1224337400008)) ;
#6872=CARTESIAN_POINT('',(57.3984711260663,45.3822493559848,76.8474249390433)) ;
#6873=CARTESIAN_POINT('Origin',(23.47768801576,45.3822493559848,68.2224337400008)) ;
#6874=CARTESIAN_POINT('',(49.11218721881,45.3822493559848,92.0527180565764)) ;
#6875=CARTESIAN_POINT('Origin',(43.9853083041937,45.3822493559848,87.2866806464355)) ;
#6876=CARTESIAN_POINT('',(38.075012827077,45.3822493559848,91.0374682134905)) ;
#6877=CARTESIAN_POINT('Origin',(27.5808403303614,45.3822493559848,74.5012983732667)) ;
#6878=CARTESIAN_POINT('Ctrl Pts',(27.6340699934267,57.8265499701676,74.5851749008597)) ;
#6879=CARTESIAN_POINT('Ctrl Pts',(27.6340965843113,57.8721147554955,74.585216801389)) ;
#6880=CARTESIAN_POINT('Ctrl Pts',(27.6363074785453,57.9184467890563,74.5887006131945)) ;
#6881=CARTESIAN_POINT('Ctrl Pts',(27.6453547210266,58.0066958708245,74.6029567861613)) ;
#6882=CARTESIAN_POINT('Ctrl Pts',(27.6523019245548,58.0508719524288,74.6139038272942)) ;
#6883=CARTESIAN_POINT('Ctrl Pts',(27.671671280061,58.1278680023598,74.6444250477569)) ;
#6884=CARTESIAN_POINT('Ctrl Pts',(27.6828616512215,58.1579990080347,74.6620582511416)) ;
#6885=CARTESIAN_POINT('Ctrl Pts',(27.7020567681637,58.1911673828821,74.6923049155601)) ;
#6886=CARTESIAN_POINT('Ctrl Pts',(27.7096119577989,58.201115371274,74.7042099894589)) ;
#6887=CARTESIAN_POINT('Ctrl Pts',(27.7250554624726,58.2136587167095,74.7285450588789)) ;
#6888=CARTESIAN_POINT('Ctrl Pts',(27.7325146430327,58.2169692427633,74.740298846674)) ;
#6889=CARTESIAN_POINT('Ctrl Pts',(27.7402369588892,58.217275807636,74.7524672693487)) ;
#6890=CARTESIAN_POINT('Ctrl Pts',(27.7390583718472,58.3830247512584,74.7506101133411)) ;
#6891=CARTESIAN_POINT('Ctrl Pts',(27.7352912521335,58.3830247228386,74.7446740825189)) ;
#6892=CARTESIAN_POINT('Ctrl Pts',(27.7315547998714,58.3837424765073,74.7387863758678)) ;
#6893=CARTESIAN_POINT('Ctrl Pts',(27.7239251145917,58.3866521090709,74.726763915626)) ;
#6894=CARTESIAN_POINT('Ctrl Pts',(27.720097441989,58.3889169428631,74.7207324687187)) ;
#6895=CARTESIAN_POINT('Ctrl Pts',(27.707904199704,58.398544443072,74.7015189932978)) ;
#6896=CARTESIAN_POINT('Ctrl Pts',(27.7002505376832,58.4085611720351,74.689458751802)) ;
#6897=CARTESIAN_POINT('Ctrl Pts',(27.68144026452,58.4411881110121,74.659818504144)) ;
#6898=CARTESIAN_POINT('Ctrl Pts',(27.6706669109948,58.470179097251,74.6428424153515)) ;
#6899=CARTESIAN_POINT('Ctrl Pts',(27.6518069653766,58.5450324120644,74.613123896429)) ;
#6900=CARTESIAN_POINT('Ctrl Pts',(27.645027480032,58.5884045335157,74.6024411370552)) ;
#6901=CARTESIAN_POINT('Ctrl Pts',(27.6361980719596,58.6752752681755,74.5885282161917)) ;
#6902=CARTESIAN_POINT('Ctrl Pts',(27.6340701087039,58.7210386854942,74.5851750825074)) ;
#6903=CARTESIAN_POINT('Ctrl Pts',(27.6340702593408,58.7660385537336,74.5851753198732)) ;
#6904=CARTESIAN_POINT('Origin',(23.47768801576,43.8830586252741,68.2224337400009)) ;
#6905=CARTESIAN_POINT('Ctrl Pts',(27.701230891149,58.2943663992286,74.7777638904556)) ;
#6906=CARTESIAN_POINT('Ctrl Pts',(27.5958999514269,58.2924602039142,74.6121580162595)) ;
#6907=CARTESIAN_POINT('Ctrl Pts',(27.4526548484823,58.191081348463,74.7000597463983)) ;
#6908=CARTESIAN_POINT('Ctrl Pts',(27.9760338094669,57.7522999681945,74.6007093188303)) ;
#6909=CARTESIAN_POINT('Ctrl Pts',(27.8637630679054,57.7503889242577,74.4395201306975)) ;
#6910=CARTESIAN_POINT('Ctrl Pts',(27.7242147844289,57.6489874075334,74.5334181808899)) ;
#6911=CARTESIAN_POINT('Ctrl Pts',(28.2392666218688,57.2111033102745,74.4066346294935)) ;
#6912=CARTESIAN_POINT('Ctrl Pts',(28.120340108254,57.2091968026367,74.2502911525297)) ;
#6913=CARTESIAN_POINT('Ctrl Pts',(27.9848160276798,57.1078632090985,74.3499766830414)) ;
#6914=CARTESIAN_POINT('Ctrl Pts',(28.6139877302149,56.3997926693382,74.0923287003896)) ;
#6915=CARTESIAN_POINT('Ctrl Pts',(28.4855837933368,56.3978864499605,73.9438397893937)) ;
#6916=CARTESIAN_POINT('Ctrl Pts',(28.3566661229263,56.2965290899915,74.0517406446381)) ;
#6917=CARTESIAN_POINT('Ctrl Pts',(28.7356674654984,56.1295297083681,73.9835911448773)) ;
#6918=CARTESIAN_POINT('Ctrl Pts',(28.6041845210826,56.1276240321417,73.8378196428817)) ;
#6919=CARTESIAN_POINT('Ctrl Pts',(28.4775758252667,56.0262125668428,73.9483736489995)) ;
#6920=CARTESIAN_POINT('Ctrl Pts',(28.9719840952407,55.5885108130589,73.7586758721593)) ;
#6921=CARTESIAN_POINT('Ctrl Pts',(28.8345207694355,55.5866055506407,73.6185325946753)) ;
#6922=CARTESIAN_POINT('Ctrl Pts',(28.7126128644989,55.485272016298,73.7343143425878)) ;
#6923=CARTESIAN_POINT('Ctrl Pts',(29.0865699779388,55.3179011606642,73.6425604457781)) ;
#6924=CARTESIAN_POINT('Ctrl Pts',(28.9462064140221,55.3159940909988,73.505321568464)) ;
#6925=CARTESIAN_POINT('Ctrl Pts',(28.8267510070548,55.2146518759856,73.6236251304476)) ;
#6926=CARTESIAN_POINT('Ctrl Pts',(29.3085722187904,54.7764805321466,73.4029882220714)) ;
#6927=CARTESIAN_POINT('Ctrl Pts',(29.1625852444779,54.774572825861,73.2717424098044)) ;
#6928=CARTESIAN_POINT('Ctrl Pts',(29.0482354201187,54.673110454093,73.3948939802413)) ;
#6929=CARTESIAN_POINT('Ctrl Pts',(29.4159635790958,54.5052712784355,73.2795250922713)) ;
#6930=CARTESIAN_POINT('Ctrl Pts',(29.2672561254484,54.5033650628135,73.15137495925)) ;
#6931=CARTESIAN_POINT('Ctrl Pts',(29.1554659475733,54.4020271817646,73.2769499969672)) ;
#6932=CARTESIAN_POINT('Ctrl Pts',(29.6223275764867,53.9638812711181,73.0266714360963)) ;
#6933=CARTESIAN_POINT('Ctrl Pts',(29.4683889353564,53.9619749130608,72.904853826243)) ;
#6934=CARTESIAN_POINT('Ctrl Pts',(29.3619600045789,53.8606102461995,73.0349839991175)) ;
#6935=CARTESIAN_POINT('Ctrl Pts',(29.7215414387002,53.6935003224137,72.8969989184745)) ;
#6936=CARTESIAN_POINT('Ctrl Pts',(29.5650860546413,53.6915946088719,72.7784296249195)) ;
#6937=CARTESIAN_POINT('Ctrl Pts',(29.4614165662687,53.5901950776532,72.9107431890366)) ;
#6938=CARTESIAN_POINT('Ctrl Pts',(29.9115055718179,53.1525885953454,72.6318830248109)) ;
#6939=CARTESIAN_POINT('Ctrl Pts',(29.7502308147021,53.1506832357955,72.519960101264)) ;
#6940=CARTESIAN_POINT('Ctrl Pts',(29.6521604773189,53.0493503316648,72.6565224488048)) ;
#6941=CARTESIAN_POINT('Ctrl Pts',(30.0022476308534,52.8821999703571,72.4964697871063)) ;
#6942=CARTESIAN_POINT('Ctrl Pts',(29.8386696042462,52.8802927777291,72.3879401740398)) ;
#6943=CARTESIAN_POINT('Ctrl Pts',(29.7434802703421,52.7789455602736,72.5265162325635)) ;
#6944=CARTESIAN_POINT('Ctrl Pts',(30.1752481522115,52.3415574725627,72.2199301771275)) ;
#6945=CARTESIAN_POINT('Ctrl Pts',(30.0072737051043,52.3396495857223,72.1183311368414)) ;
#6946=CARTESIAN_POINT('Ctrl Pts',(29.9180030493363,52.238171223764,72.2607032887875)) ;
#6947=CARTESIAN_POINT('Ctrl Pts',(30.2574477094345,52.0708923183366,72.0788769583042)) ;
#6948=CARTESIAN_POINT('Ctrl Pts',(30.0873852279632,52.0689860211252,71.9808203864691)) ;
#6949=CARTESIAN_POINT('Ctrl Pts',(30.0010696677543,51.9676510264301,72.1250989973514)) ;
#6950=CARTESIAN_POINT('Ctrl Pts',(30.4128652817387,51.5294526417347,71.7918342379605)) ;
#6951=CARTESIAN_POINT('Ctrl Pts',(30.2388484777668,51.5275461441316,71.7009779039191)) ;
#6952=CARTESIAN_POINT('Ctrl Pts',(30.1586558523266,51.4261734609838,71.8487228977031)) ;
#6953=CARTESIAN_POINT('Ctrl Pts',(30.4862356409264,51.2584285629312,71.6455299256122)) ;
#6954=CARTESIAN_POINT('Ctrl Pts',(30.3103502329215,51.2565228089169,71.5583449567437)) ;
#6955=CARTESIAN_POINT('Ctrl Pts',(30.2332792416858,51.1551340723184,71.7077317483349)) ;
#6956=CARTESIAN_POINT('Ctrl Pts',(30.623370841369,50.7168256230282,71.349178490017)) ;
#6957=CARTESIAN_POINT('Ctrl Pts',(30.4439912380647,50.7149201642829,71.2694333365719)) ;
#6958=CARTESIAN_POINT('Ctrl Pts',(30.3732265233668,50.613586979054,71.4219436569748)) ;
#6959=CARTESIAN_POINT('Ctrl Pts',(30.6871919121486,50.4462620313546,71.1990637682367)) ;
#6960=CARTESIAN_POINT('Ctrl Pts',(30.5061840531774,50.4443547062135,71.1230856787473)) ;
#6961=CARTESIAN_POINT('Ctrl Pts',(30.4386300692504,50.343001553274,71.2770326034523)) ;
#6962=CARTESIAN_POINT('Ctrl Pts',(30.8053663173622,49.9056099882931,70.8949668202972)) ;
#6963=CARTESIAN_POINT('Ctrl Pts',(30.6213369332285,49.9037019096529,70.8266210208818)) ;
#6964=CARTESIAN_POINT('Ctrl Pts',(30.5603112897766,49.8022062837453,70.9831829221991)) ;
#6965=CARTESIAN_POINT('Ctrl Pts',(30.8596553784308,49.635040821774,70.7411227832435)) ;
#6966=CARTESIAN_POINT('Ctrl Pts',(30.6742396913967,49.6331344367333,70.6766456166729)) ;
#6967=CARTESIAN_POINT('Ctrl Pts',(30.6164673707908,49.5318014383246,70.8345361175774)) ;
#6968=CARTESIAN_POINT('Ctrl Pts',(30.9584720415982,49.0942250306884,70.4304004819357)) ;
#6969=CARTESIAN_POINT('Ctrl Pts',(30.7705226537011,49.0923183862279,70.3737276915643)) ;
#6970=CARTESIAN_POINT('Ctrl Pts',(30.7194087768269,48.9909365753838,70.5338683441997)) ;
#6971=CARTESIAN_POINT('Ctrl Pts',(31.0030604905696,48.8238179925337,70.2733051326608)) ;
#6972=CARTESIAN_POINT('Ctrl Pts',(30.8139656641572,48.8219121926088,70.2205800897392)) ;
#6973=CARTESIAN_POINT('Ctrl Pts',(30.7662145198663,48.720533172951,70.3817571390707)) ;
#6974=CARTESIAN_POINT('Ctrl Pts',(31.0822781893569,48.2823982253176,69.9566492356375)) ;
#6975=CARTESIAN_POINT('Ctrl Pts',(30.8911438797355,48.2804926625113,69.9118831048759)) ;
#6976=CARTESIAN_POINT('Ctrl Pts',(30.8501713843621,48.1791582421951,70.0749415328362)) ;
#6977=CARTESIAN_POINT('Ctrl Pts',(31.1169423489645,48.0114576298754,69.7969790787265)) ;
#6978=CARTESIAN_POINT('Ctrl Pts',(30.9249086717214,48.009552069648,69.756223244743)) ;
#6979=CARTESIAN_POINT('Ctrl Pts',(30.8873821347699,47.9080609643586,69.9200170457096)) ;
#6980=CARTESIAN_POINT('Ctrl Pts',(31.1762008520855,47.4697670851897,69.475538363929)) ;
#6981=CARTESIAN_POINT('Ctrl Pts',(30.9826313664683,47.4678622558982,69.4428669398108)) ;
#6982=CARTESIAN_POINT('Ctrl Pts',(30.9519839904029,47.3665093096401,69.6081666509721)) ;
#6983=CARTESIAN_POINT('Ctrl Pts',(31.2007210276185,47.1991192501307,69.3142255810316)) ;
#6984=CARTESIAN_POINT('Ctrl Pts',(31.0065113086846,47.1972127705462,69.2856097758525)) ;
#6985=CARTESIAN_POINT('Ctrl Pts',(30.9793273889069,47.0958808569866,69.4515263244446)) ;
#6986=CARTESIAN_POINT('Ctrl Pts',(31.2396113270229,46.6582159321595,68.9904228772838)) ;
#6987=CARTESIAN_POINT('Ctrl Pts',(31.0443737081918,46.6563091332066,68.9699494408894)) ;
#6988=CARTESIAN_POINT('Ctrl Pts',(31.0241543176845,46.5549171221787,69.136823273953)) ;
#6989=CARTESIAN_POINT('Ctrl Pts',(31.2539830666496,46.3878930438546,68.82781193536)) ;
#6990=CARTESIAN_POINT('Ctrl Pts',(31.0583602495382,46.3859871917592,68.8114299191662)) ;
#6991=CARTESIAN_POINT('Ctrl Pts',(31.0416355352769,46.2846172014713,68.9787027814551)) ;
#6992=CARTESIAN_POINT('Ctrl Pts',(31.2724899758963,45.847008993619,68.5022603903092)) ;
#6993=CARTESIAN_POINT('Ctrl Pts',(31.0763542296701,45.8451033188908,68.4940696998761)) ;
#6994=CARTESIAN_POINT('Ctrl Pts',(31.0666340319201,45.7437666877133,68.6619144618478)) ;
#6995=CARTESIAN_POINT('Ctrl Pts',(31.276642725521,45.576594876658,68.3392191581406)) ;
#6996=CARTESIAN_POINT('Ctrl Pts',(31.0803756867806,45.5746876691305,68.335128608911)) ;
#6997=CARTESIAN_POINT('Ctrl Pts',(31.0741702161106,45.4732994150359,68.5031114092514)) ;
#6998=CARTESIAN_POINT('Ctrl Pts',(31.2756697210528,45.3060601767044,68.1759683239932)) ;
#6999=CARTESIAN_POINT('Ctrl Pts',(31.079403573458,45.3041537286489,68.1759873411111)) ;
#7000=CARTESIAN_POINT('Ctrl Pts',(31.0767156357415,45.2027271666488,68.3440035995781)) ;
#7001=CARTESIAN_POINT('Ctrl Pts',(31.2707596705055,45.1993067880441,68.0115966179513)) ;
#7002=CARTESIAN_POINT('Ctrl Pts',(31.0767059192039,45.2022941676425,68.0161583317382)) ;
#7003=CARTESIAN_POINT('Ctrl Pts',(31.0685647903147,45.3026134137914,67.8501572385602)) ;
#7004=CARTESIAN_POINT('Ctrl Pts',(31.2753738913076,45.4820412744326,68.1821045031859)) ;
#7005=CARTESIAN_POINT('Ctrl Pts',(31.0812188154374,45.485027067948,68.1824209119147)) ;
#7006=CARTESIAN_POINT('Ctrl Pts',(31.0767098704522,45.5853439255345,68.0162388993778)) ;
#7007=CARTESIAN_POINT('Ctrl Pts',(31.2743767150006,45.7643410734729,68.3523909127677)) ;
#7008=CARTESIAN_POINT('Ctrl Pts',(31.0802656447196,45.7673274764098,68.3484647485212)) ;
#7009=CARTESIAN_POINT('Ctrl Pts',(31.0793851694405,45.8675609241944,68.182178381083)) ;
#7010=CARTESIAN_POINT('Ctrl Pts',(31.2613182473705,46.3280183066973,68.6918476698476)) ;
#7011=CARTESIAN_POINT('Ctrl Pts',(31.0675617987265,46.3310049156009,68.6794713223723)) ;
#7012=CARTESIAN_POINT('Ctrl Pts',(31.0739245141333,46.4312549192508,68.5133137341179)) ;
#7013=CARTESIAN_POINT('Ctrl Pts',(31.2492433795396,46.6093355962432,68.8612448090648)) ;
#7014=CARTESIAN_POINT('Ctrl Pts',(31.0558010086264,46.6123217179656,68.844652477278)) ;
#7015=CARTESIAN_POINT('Ctrl Pts',(31.0657791914954,46.7126174787595,68.6786988015514)) ;
#7016=CARTESIAN_POINT('Ctrl Pts',(31.2141263134973,47.1717937444718,69.1984722106304)) ;
#7017=CARTESIAN_POINT('Ctrl Pts',(31.0215907151539,47.1747789756108,69.1734846605815)) ;
#7018=CARTESIAN_POINT('Ctrl Pts',(31.0387767823933,47.2750030883528,69.0080813459652)) ;
#7019=CARTESIAN_POINT('Ctrl Pts',(31.1911024008108,47.4527838882087,69.3662496718402)) ;
#7020=CARTESIAN_POINT('Ctrl Pts',(30.9991541250229,47.4557718391023,69.3370888215369)) ;
#7021=CARTESIAN_POINT('Ctrl Pts',(31.019928636683,47.5560106521893,69.1721061379612)) ;
#7022=CARTESIAN_POINT('Ctrl Pts',(31.1341568670205,48.0142871287658,69.7001372321145)) ;
#7023=CARTESIAN_POINT('Ctrl Pts',(30.9436506057594,48.0172768213744,69.6626716706322)) ;
#7024=CARTESIAN_POINT('Ctrl Pts',(30.9715585882536,48.1176560532481,69.4988251729331)) ;
#7025=CARTESIAN_POINT('Ctrl Pts',(31.1002449637116,48.295266819104,69.8661099004534)) ;
#7026=CARTESIAN_POINT('Ctrl Pts',(30.910603800394,48.2982535237946,69.8245104998946)) ;
#7027=CARTESIAN_POINT('Ctrl Pts',(30.942078500755,48.3984774868501,69.6612225081025)) ;
#7028=CARTESIAN_POINT('Ctrl Pts',(31.0217140098796,48.8569739450444,70.1954351770645)) ;
#7029=CARTESIAN_POINT('Ctrl Pts',(30.8340552348197,48.8599612930095,70.1456443070115)) ;
#7030=CARTESIAN_POINT('Ctrl Pts',(30.872582034942,48.9602369846067,69.9839049650751)) ;
#7031=CARTESIAN_POINT('Ctrl Pts',(30.9770284257322,49.1378578224526,70.3590251080683)) ;
#7032=CARTESIAN_POINT('Ctrl Pts',(30.7904973368589,49.1408439739939,70.3051641970359)) ;
#7033=CARTESIAN_POINT('Ctrl Pts',(30.8325331930582,49.2411084827197,70.1442945851104)) ;
#7034=CARTESIAN_POINT('Ctrl Pts',(30.8770845405165,49.7002903800716,70.6829312861811)) ;
#7035=CARTESIAN_POINT('Ctrl Pts',(30.6930720380202,49.7032760750572,70.6210138296207)) ;
#7036=CARTESIAN_POINT('Ctrl Pts',(30.742065302515,49.8035038746341,70.4621032079514)) ;
#7037=CARTESIAN_POINT('Ctrl Pts',(30.8218159490199,49.9815741041477,70.8433329295991)) ;
#7038=CARTESIAN_POINT('Ctrl Pts',(30.6391884935956,49.9845603797238,70.7774284628369)) ;
#7039=CARTESIAN_POINT('Ctrl Pts',(30.6916049557576,50.084920629536,70.6196923965754)) ;
#7040=CARTESIAN_POINT('Ctrl Pts',(30.7005980268366,50.5452598054567,71.1609464797428)) ;
#7041=CARTESIAN_POINT('Ctrl Pts',(30.5210220118427,50.5482445256766,71.0871424982923)) ;
#7042=CARTESIAN_POINT('Ctrl Pts',(30.5802875368357,50.6484794514056,70.9317743843129)) ;
#7043=CARTESIAN_POINT('Ctrl Pts',(30.6347845222986,50.8275371605558,71.3178190881531)) ;
#7044=CARTESIAN_POINT('Ctrl Pts',(30.4568608995758,50.8305243023805,71.2401164427609)) ;
#7045=CARTESIAN_POINT('Ctrl Pts',(30.5195054534064,50.9307473367164,71.0860721504808)) ;
#7046=CARTESIAN_POINT('Ctrl Pts',(30.5281930551463,51.2516112326399,71.5502037790437)) ;
#7047=CARTESIAN_POINT('Ctrl Pts',(30.3529412567396,51.2545984104442,71.4667251371801)) ;
#7048=CARTESIAN_POINT('Ctrl Pts',(30.4205752839267,51.3548887142843,71.3148795074004)) ;
#7049=CARTESIAN_POINT('Ctrl Pts',(30.4913107555821,51.3931523912117,71.6272529315444)) ;
#7050=CARTESIAN_POINT('Ctrl Pts',(30.3169834983725,51.3961391935532,71.5418590470166)) ;
#7051=CARTESIAN_POINT('Ctrl Pts',(30.3862730556347,51.4964465474926,71.3907722579837)) ;
#7052=CARTESIAN_POINT('Ctrl Pts',(30.4151092402135,51.6761627264651,71.7799422493361)) ;
#7053=CARTESIAN_POINT('Ctrl Pts',(30.242695078949,51.6791488679195,71.6907527013559)) ;
#7054=CARTESIAN_POINT('Ctrl Pts',(30.3152873232083,51.7794030062388,71.5411913280897)) ;
#7055=CARTESIAN_POINT('Ctrl Pts',(30.3757935636177,51.8176028378213,71.8555858876626)) ;
#7056=CARTESIAN_POINT('Ctrl Pts',(30.2043654786474,51.8205891355611,71.7645164524545)) ;
#7057=CARTESIAN_POINT('Ctrl Pts',(30.2785921329714,51.9208298261689,71.6157510097026)) ;
#7058=CARTESIAN_POINT('Ctrl Pts',(30.2542175154657,52.2417288193145,72.0804228994921)) ;
#7059=CARTESIAN_POINT('Ctrl Pts',(30.0858363153209,52.2447151365677,71.9837662267925)) ;
#7060=CARTESIAN_POINT('Ctrl Pts',(30.1649131134242,52.3449566194198,71.8374878351155)) ;
#7061=CARTESIAN_POINT('Ctrl Pts',(30.1682702114188,52.5241300049717,72.22762270877)) ;
#7062=CARTESIAN_POINT('Ctrl Pts',(30.00203922285,52.5271161388606,72.1273087609404)) ;
#7063=CARTESIAN_POINT('Ctrl Pts',(30.0842751721127,52.6274277787848,71.9828283867849)) ;
#7064=CARTESIAN_POINT('Ctrl Pts',(29.9869590883597,53.0891744812326,72.5160091947715)) ;
#7065=CARTESIAN_POINT('Ctrl Pts',(29.8252717919771,53.0921595377507,72.4085302103788)) ;
#7066=CARTESIAN_POINT('Ctrl Pts',(29.9137644892835,53.1923844744817,72.267737360374)) ;
#7067=CARTESIAN_POINT('Ctrl Pts',(29.8916728500753,53.371665470285,72.6570941471294)) ;
#7068=CARTESIAN_POINT('Ctrl Pts',(29.7323692115319,53.3746531996403,72.5461122770274)) ;
#7069=CARTESIAN_POINT('Ctrl Pts',(29.8239134874277,53.4748857690477,72.4072892427669)) ;
#7070=CARTESIAN_POINT('Ctrl Pts',(29.6918335619832,53.9365848433157,72.9330442939948)) ;
#7071=CARTESIAN_POINT('Ctrl Pts',(29.5375242163636,53.9395741566825,72.8152101149305)) ;
#7072=CARTESIAN_POINT('Ctrl Pts',(29.6350044013411,54.0399343658719,72.6805777758222)) ;
#7073=CARTESIAN_POINT('Ctrl Pts',(29.5873107371871,54.2194050938079,73.067842310348)) ;
#7074=CARTESIAN_POINT('Ctrl Pts',(29.4356221911967,54.2223916876785,72.9466599778714)) ;
#7075=CARTESIAN_POINT('Ctrl Pts',(29.5360678154317,54.3226177650003,72.8141303651837)) ;
#7076=CARTESIAN_POINT('Ctrl Pts',(29.3695790835415,54.7853172886214,73.3303792062082)) ;
#7077=CARTESIAN_POINT('Ctrl Pts',(29.2233330805696,54.7883043794011,73.2026795844699)) ;
#7078=CARTESIAN_POINT('Ctrl Pts',(29.329464103686,54.888570414198,73.0746868570139)) ;
#7079=CARTESIAN_POINT('Ctrl Pts',(29.2562377433629,55.0683374452758,73.4582537530578)) ;
#7080=CARTESIAN_POINT('Ctrl Pts',(29.1128251734266,55.0713235720022,73.3273798129575)) ;
#7081=CARTESIAN_POINT('Ctrl Pts',(29.221732199964,55.1715968138862,73.2017461799581)) ;
#7082=CARTESIAN_POINT('Ctrl Pts',(29.0219184628403,55.6338317485941,73.7057667733599)) ;
#7083=CARTESIAN_POINT('Ctrl Pts',(28.884364077656,55.6368172834005,73.5687509636409)) ;
#7084=CARTESIAN_POINT('Ctrl Pts',(28.9986751021317,55.7370429277092,73.4479765402196)) ;
#7085=CARTESIAN_POINT('Ctrl Pts',(28.9008692462189,55.9162154787378,73.8255204414319)) ;
#7086=CARTESIAN_POINT('Ctrl Pts',(28.7663331269695,55.9192018042793,73.6855329720701)) ;
#7087=CARTESIAN_POINT('Ctrl Pts',(28.8831959257244,56.0195762764982,73.5673440006423)) ;
#7088=CARTESIAN_POINT('Ctrl Pts',(28.6508660111268,56.4812254904529,74.0571282289314)) ;
#7089=CARTESIAN_POINT('Ctrl Pts',(28.5225811568725,56.484210134814,73.9113965902898)) ;
#7090=CARTESIAN_POINT('Ctrl Pts',(28.6445514045126,56.5844490941092,73.798373497653)) ;
#7091=CARTESIAN_POINT('Ctrl Pts',(28.522236149594,56.7637439358821,74.1686873940088)) ;
#7092=CARTESIAN_POINT('Ctrl Pts',(28.3971633157449,56.7667309512438,74.0201907033106)) ;
#7093=CARTESIAN_POINT('Ctrl Pts',(28.5215800577612,56.8669533046419,73.9098522901186)) ;
#7094=CARTESIAN_POINT('Ctrl Pts',(28.2577296814636,57.3288079962307,74.38332865809)) ;
#7095=CARTESIAN_POINT('Ctrl Pts',(28.1392580206003,57.3317959921775,74.2295107078863)) ;
#7096=CARTESIAN_POINT('Ctrl Pts',(28.2683410236814,57.4320972449965,74.1247401072848)) ;
#7097=CARTESIAN_POINT('Ctrl Pts',(28.1217698050726,57.611503670377,74.4864574136107)) ;
#7098=CARTESIAN_POINT('Ctrl Pts',(28.0066954436726,57.614489922013,74.3300837580924)) ;
#7099=CARTESIAN_POINT('Ctrl Pts',(28.1380642361742,57.71473561364,74.2281426830806)) ;
#7100=CARTESIAN_POINT('Ctrl Pts',(27.843365296793,58.1775332619195,74.6835750662936)) ;
#7101=CARTESIAN_POINT('Ctrl Pts',(27.735240524604,58.1805194049571,74.5223182830966)) ;
#7102=CARTESIAN_POINT('Ctrl Pts',(27.8709460181227,58.2807563670581,74.4262173072657)) ;
#7103=CARTESIAN_POINT('Ctrl Pts',(27.7007840548285,58.4605262973727,74.7776533339454)) ;
#7104=CARTESIAN_POINT('Ctrl Pts',(27.5962147138393,58.4635110441087,74.614065002193)) ;
#7105=CARTESIAN_POINT('Ctrl Pts',(27.7339403582833,58.5638587343234,74.5209942372437)) ;
#7106=CARTESIAN_POINT('Ctrl Pts',(27.5556022785721,58.7433256931628,74.8667534769041)) ;
#7107=CARTESIAN_POINT('Ctrl Pts',(27.4546609736715,58.7463119239391,74.7009621614397)) ;
#7108=CARTESIAN_POINT('Ctrl Pts',(27.5944222023064,58.846513767945,74.6108998812056)) ;
#7109=CARTESIAN_POINT('Origin',(34.2457299930682,45.3830586252741,34.9200048199517)) ;
#7110=CARTESIAN_POINT('',(25.8874358604319,45.3830610445957,60.805979493395)) ;
#7111=CARTESIAN_POINT('',(32.227700990655,45.3830586252741,41.2926628570961)) ;
#7112=CARTESIAN_POINT('',(25.887439674075,45.3830586252741,60.8059807325238)) ;
#7113=CARTESIAN_POINT('Ctrl Pts',(25.8874344722073,45.3830586252741,60.805979042333)) ;
#7114=CARTESIAN_POINT('Ctrl Pts',(25.8831617902991,45.3830586252741,60.8191290015772)) ;
#7115=CARTESIAN_POINT('Ctrl Pts',(25.8805089846612,45.3830586252741,60.8327110288752)) ;
#7116=CARTESIAN_POINT('Ctrl Pts',(25.8783596228545,45.3830586252741,60.861390991021)) ;
#7117=CARTESIAN_POINT('Ctrl Pts',(25.8791455812147,45.3830586252741,60.876331277846)) ;
#7118=CARTESIAN_POINT('Ctrl Pts',(25.8863194956573,45.3830586252741,60.9178099819017)) ;
#7119=CARTESIAN_POINT('Ctrl Pts',(25.8966456738107,45.3830586252741,60.9432469495347)) ;
#7120=CARTESIAN_POINT('Ctrl Pts',(25.9270686569879,45.3830586252741,60.9910540894173)) ;
#7121=CARTESIAN_POINT('Ctrl Pts',(25.9476816529992,45.3830586252736,61.0126928579513)) ;
#7122=CARTESIAN_POINT('Ctrl Pts',(25.9926879310718,45.3830586252736,61.0462961404911)) ;
#7123=CARTESIAN_POINT('Ctrl Pts',(26.0164911651481,45.3830586252741,61.0589713793357)) ;
#7124=CARTESIAN_POINT('Ctrl Pts',(26.0416005791977,45.3830586252741,61.0679696745342)) ;
#7125=CARTESIAN_POINT('',(25.7914429954097,45.3830674541108,60.7777739865218)) ;
#7126=CARTESIAN_POINT('Ctrl Pts',(25.5149631682037,45.3830586252741,60.9005821812565)) ;
#7127=CARTESIAN_POINT('Ctrl Pts',(25.540242497525,45.3830586252741,60.9076155911763)) ;
#7128=CARTESIAN_POINT('Ctrl Pts',(25.5665430671899,45.3830586252745,60.9110143156868)) ;
#7129=CARTESIAN_POINT('Ctrl Pts',(25.6223302267837,45.3830586252745,60.9098503269198)) ;
#7130=CARTESIAN_POINT('Ctrl Pts',(25.651747876875,45.3830586252741,60.9042145461539)) ;
#7131=CARTESIAN_POINT('Ctrl Pts',(25.7044084924816,45.3830586252741,60.8829582286584)) ;
#7132=CARTESIAN_POINT('Ctrl Pts',(25.7276504263598,45.3830586252741,60.8682338698508)) ;
#7133=CARTESIAN_POINT('Ctrl Pts',(25.7574812296411,45.3830586252741,60.8387754420949)) ;
#7134=CARTESIAN_POINT('Ctrl Pts',(25.7666879461075,45.3830586252741,60.8272731403928)) ;
#7135=CARTESIAN_POINT('Ctrl Pts',(25.7814944876552,45.3830586252741,60.8031132388058)) ;
#7136=CARTESIAN_POINT('Ctrl Pts',(25.787226289558,45.3830586252741,60.7907346901948)) ;
#7137=CARTESIAN_POINT('Ctrl Pts',(25.7914379104393,45.3830586252741,60.7777724061309)) ;
#7138=CARTESIAN_POINT('',(31.768269675766,45.3830586252741,42.3830402536426)) ;
#7139=CARTESIAN_POINT('',(31.768269675766,45.3830586252741,42.3830402536426)) ;
#7140=CARTESIAN_POINT('Origin',(38.4256652898321,45.3830586252741,44.5461592142672)) ;
#7141=CARTESIAN_POINT('Ctrl Pts',(25.7953108450845,45.383050240221,61.0895083639021)) ;
#7142=CARTESIAN_POINT('Ctrl Pts',(26.1250882066852,45.9804808943743,61.1966592874771)) ;
#7143=CARTESIAN_POINT('Ctrl Pts',(26.443572067289,46.5779115664506,61.3337813469064)) ;
#7144=CARTESIAN_POINT('Ctrl Pts',(26.7620536881248,47.1753380370388,61.4709024420119)) ;
#7145=CARTESIAN_POINT('Ctrl Pts',(27.0665247840196,47.772764507627,61.6368243793731)) ;
#7146=CARTESIAN_POINT('Ctrl Pts',(27.3709958799144,48.3701909782152,61.8027463167343)) ;
#7147=CARTESIAN_POINT('Ctrl Pts',(27.6588588108316,48.9676174488035,61.9960535088842)) ;
#7148=CARTESIAN_POINT('Ctrl Pts',(27.9467217417488,49.5650439193917,62.1893607010341)) ;
#7149=CARTESIAN_POINT('Ctrl Pts',(28.2155205626593,50.16247038998,62.4084039191674)) ;
#7150=CARTESIAN_POINT('Ctrl Pts',(28.4843193835699,50.7598968605682,62.6274471373006)) ;
#7151=CARTESIAN_POINT('Ctrl Pts',(28.7317607977096,51.3573233311564,62.8703575819127)) ;
#7152=CARTESIAN_POINT('Ctrl Pts',(28.9792022118494,51.9547498017447,63.1132680265248)) ;
#7153=CARTESIAN_POINT('Ctrl Pts',(29.2031751363182,52.5521762723329,63.3779732713499)) ;
#7154=CARTESIAN_POINT('Ctrl Pts',(29.4271480607871,53.1496027429211,63.6426785161751)) ;
#7155=CARTESIAN_POINT('Ctrl Pts',(29.6257416375641,53.7470292135094,63.9269201893971)) ;
#7156=CARTESIAN_POINT('Ctrl Pts',(29.8243352143411,54.3444556840976,64.211161862619)) ;
#7157=CARTESIAN_POINT('Ctrl Pts',(29.9958551130514,54.9418821546858,64.5125149145025)) ;
#7158=CARTESIAN_POINT('Ctrl Pts',(30.1673750117617,55.5393086252741,64.813867966386)) ;
#7159=CARTESIAN_POINT('Ctrl Pts',(30.3103578851056,56.1367350958623,65.1297613589466)) ;
#7160=CARTESIAN_POINT('Ctrl Pts',(30.4533407584495,56.7341615664506,65.4456547515071)) ;
#7161=CARTESIAN_POINT('Ctrl Pts',(30.5665667269661,57.3315880370388,65.7733933937002)) ;
#7162=CARTESIAN_POINT('Ctrl Pts',(30.6661847295087,57.8572133193466,66.0617430481042)) ;
#7163=CARTESIAN_POINT('Ctrl Pts',(30.7420543581155,58.3830758086166,66.3572308973985)) ;
#7164=CARTESIAN_POINT('Ctrl Pts',(34.2932612192744,45.383050240221,34.9354486515399)) ;
#7165=CARTESIAN_POINT('Ctrl Pts',(35.8322222400776,45.9804808943743,35.4354862948897)) ;
#7166=CARTESIAN_POINT('Ctrl Pts',(37.3184802562288,46.5779115664506,36.0753892388935)) ;
#7167=CARTESIAN_POINT('Ctrl Pts',(38.804727820129,47.1753380370388,36.7152876827189)) ;
#7168=CARTESIAN_POINT('Ctrl Pts',(40.2255929343049,47.772764507627,37.4895900570713)) ;
#7169=CARTESIAN_POINT('Ctrl Pts',(41.6464580484807,48.3701909782152,38.2638924314238)) ;
#7170=CARTESIAN_POINT('Ctrl Pts',(42.9898183927608,48.9676174488035,39.1659926614565)) ;
#7171=CARTESIAN_POINT('Ctrl Pts',(44.333178737041,49.5650439193917,40.0680928914892)) ;
#7172=CARTESIAN_POINT('Ctrl Pts',(45.5875732346236,50.16247038998,41.0902945761112)) ;
#7173=CARTESIAN_POINT('Ctrl Pts',(46.8419677322063,50.7598968605682,42.1124962607332)) ;
#7174=CARTESIAN_POINT('Ctrl Pts',(47.996694331525,51.3573233311564,43.2460783355894)) ;
#7175=CARTESIAN_POINT('Ctrl Pts',(49.1514209308438,51.9547498017447,44.3796604104456)) ;
#7176=CARTESIAN_POINT('Ctrl Pts',(50.1966279116985,52.5521762723329,45.6149515529632)) ;
#7177=CARTESIAN_POINT('Ctrl Pts',(51.2418348925531,53.1496027429211,46.8502426954807)) ;
#7178=CARTESIAN_POINT('Ctrl Pts',(52.1686049175126,53.7470292135094,48.176703837183)) ;
#7179=CARTESIAN_POINT('Ctrl Pts',(53.0953749424721,54.3444556840976,49.5031649788854)) ;
#7180=CARTESIAN_POINT('Ctrl Pts',(53.8958011364534,54.9418821546858,50.9094792210085)) ;
#7181=CARTESIAN_POINT('Ctrl Pts',(54.6962273304346,55.5393086252741,52.3157934631316)) ;
#7182=CARTESIAN_POINT('Ctrl Pts',(55.363480739373,56.1367350958623,53.7899626284141)) ;
#7183=CARTESIAN_POINT('Ctrl Pts',(56.0307341483113,56.7341615664505,55.2641317936966)) ;
#7184=CARTESIAN_POINT('Ctrl Pts',(56.5591220013886,57.3315880370388,56.7935787905978)) ;
#7185=CARTESIAN_POINT('Ctrl Pts',(57.0240060132542,57.8572133193466,58.1392105111498)) ;
#7186=CARTESIAN_POINT('Ctrl Pts',(57.3780642800859,58.3830758086166,59.5181538078565)) ;
#7187=CARTESIAN_POINT('',(49.6868966603788,58.3353824278239,61.3897862372794)) ;
#7188=CARTESIAN_POINT('',(31.0053184302396,58.2172712656978,66.1863974475356)) ;
#7189=CARTESIAN_POINT('Ctrl Pts',(49.6868966603788,58.3353824278239,61.3897862372794)) ;
#7190=CARTESIAN_POINT('Ctrl Pts',(47.1887437966009,58.3308357090662,62.0312028752173)) ;
#7191=CARTESIAN_POINT('Ctrl Pts',(44.3889324086846,58.3244410141137,62.7500722580065)) ;
#7192=CARTESIAN_POINT('Ctrl Pts',(39.5787343864927,58.306635184046,63.9851211967428)) ;
#7193=CARTESIAN_POINT('Ctrl Pts',(34.295419682726,58.2895264446021,65.3416458528576)) ;
#7194=CARTESIAN_POINT('Ctrl Pts',(31.0053191458883,58.2172696107889,66.1864000932465)) ;
#7195=CARTESIAN_POINT('Ctrl Pts',(31.0053184302396,58.2172712656978,66.1863974475356)) ;
#7196=CARTESIAN_POINT('Ctrl Pts',(30.9631600045902,57.9495340002377,66.0305344100695)) ;
#7197=CARTESIAN_POINT('Ctrl Pts',(30.916172209291,57.6819084045908,65.8760449063787)) ;
#7198=CARTESIAN_POINT('Ctrl Pts',(30.8645011127033,57.4145313636581,65.7233157164034)) ;
#7199=CARTESIAN_POINT('Ctrl Pts',(30.816535099193,57.1663266301673,65.5815379939713)) ;
#7200=CARTESIAN_POINT('Ctrl Pts',(30.7645218642245,56.9182638872656,65.4412351217362)) ;
#7201=CARTESIAN_POINT('Ctrl Pts',(30.7085361013266,56.6702295478714,65.3025887342681)) ;
#7202=CARTESIAN_POINT('Ctrl Pts',(30.7042115413412,56.6510704023381,65.2918791433234)) ;
#7203=CARTESIAN_POINT('Ctrl Pts',(30.6998629795545,56.6319118940957,65.2811786693435)) ;
#7204=CARTESIAN_POINT('Ctrl Pts',(30.6954904598184,56.612753845668,65.2704874240641)) ;
#7205=CARTESIAN_POINT('Ctrl Pts',(30.6381436909714,56.3614909032359,65.1302688753267)) ;
#7206=CARTESIAN_POINT('Ctrl Pts',(30.576681027564,56.1103350670457,64.9916539487321)) ;
#7207=CARTESIAN_POINT('Ctrl Pts',(30.5112384716708,55.8590202585562,64.8549672058044)) ;
#7208=CARTESIAN_POINT('Ctrl Pts',(30.5070932757221,55.8431017310512,64.8463093328762)) ;
#7209=CARTESIAN_POINT('Ctrl Pts',(30.5029322656911,55.8271830724927,64.8376594291815)) ;
#7210=CARTESIAN_POINT('Ctrl Pts',(30.4987554443582,55.8112643008985,64.8290175054764)) ;
#7211=CARTESIAN_POINT('Ctrl Pts',(30.4319637016308,55.5567064895581,64.6908241046145)) ;
#7212=CARTESIAN_POINT('Ctrl Pts',(30.3610954434403,55.3019957844227,64.5546044340852)) ;
#7213=CARTESIAN_POINT('Ctrl Pts',(30.286151897374,55.0471908391173,64.420397343297)) ;
#7214=CARTESIAN_POINT('Ctrl Pts',(30.2824189305709,55.0344989069627,64.4137124365778)) ;
#7215=CARTESIAN_POINT('Ctrl Pts',(30.2786758239704,55.0218058655742,64.4070325703337)) ;
#7216=CARTESIAN_POINT('Ctrl Pts',(30.2749226306752,55.0091118266697,64.4003578297875)) ;
#7217=CARTESIAN_POINT('Ctrl Pts',(30.1986055999066,54.7509925981972,64.2646343699017)) ;
#7218=CARTESIAN_POINT('Ctrl Pts',(30.1181614779075,54.4926055131012,64.1311058189801)) ;
#7219=CARTESIAN_POINT('Ctrl Pts',(30.0339415706751,54.2345762733045,64.0003253705781)) ;
#7220=CARTESIAN_POINT('Ctrl Pts',(30.030867315893,54.2251575070005,63.9955515299017)) ;
#7221=CARTESIAN_POINT('Ctrl Pts',(30.027787792249,54.2157389752755,63.9907809698703)) ;
#7222=CARTESIAN_POINT('Ctrl Pts',(30.0247030062888,54.2063206495465,63.9860136998315)) ;
#7223=CARTESIAN_POINT('Ctrl Pts',(29.9391306767364,53.9450551732693,63.8537690617642)) ;
#7224=CARTESIAN_POINT('Ctrl Pts',(29.8495437893631,53.6840579939692,63.7241124455533)) ;
#7225=CARTESIAN_POINT('Ctrl Pts',(29.7562013732715,53.4230444575823,63.5974004437296)) ;
#7226=CARTESIAN_POINT('Ctrl Pts',(29.7539970080238,53.4168803877747,63.5944080256523)) ;
#7227=CARTESIAN_POINT('Ctrl Pts',(29.7517905621932,53.4107163826998,63.5914172584352)) ;
#7228=CARTESIAN_POINT('Ctrl Pts',(29.7495820361275,53.4045524432162,63.5884281424623)) ;
#7229=CARTESIAN_POINT('Ctrl Pts',(29.6548939042669,53.1402803009606,63.4602730747941)) ;
#7230=CARTESIAN_POINT('Ctrl Pts',(29.5563551294916,52.8760533725781,63.3351165968918)) ;
#7231=CARTESIAN_POINT('Ctrl Pts',(29.4539651627725,52.6118787196958,63.2129643349594)) ;
#7232=CARTESIAN_POINT('Ctrl Pts',(29.34932817923,52.3419065760205,63.0881313593168)) ;
#7233=CARTESIAN_POINT('Ctrl Pts',(29.2407203431504,52.0715787920593,62.966514326652)) ;
#7234=CARTESIAN_POINT('Ctrl Pts',(29.1283839508344,51.8011908422986,62.8483944694407)) ;
#7235=CARTESIAN_POINT('Ctrl Pts',(29.1282429199986,51.8008513882913,62.8482461778511)) ;
#7236=CARTESIAN_POINT('Ctrl Pts',(29.1281018832898,51.8005119341973,62.8480978917768)) ;
#7237=CARTESIAN_POINT('Ctrl Pts',(29.1279608407085,51.8001724800172,62.8479496112184)) ;
#7238=CARTESIAN_POINT('Ctrl Pts',(29.0169624142087,51.5330270582816,62.7312550036823)) ;
#7239=CARTESIAN_POINT('Ctrl Pts',(28.9020807918313,51.265585354454,62.6177412654934)) ;
#7240=CARTESIAN_POINT('Ctrl Pts',(28.7840333481004,50.998401550286,62.5081218916898)) ;
#7241=CARTESIAN_POINT('Ctrl Pts',(28.7824465405845,50.9948100344075,62.5066483752736)) ;
#7242=CARTESIAN_POINT('Ctrl Pts',(28.7808591533881,50.9912185474961,62.5051755551275)) ;
#7243=CARTESIAN_POINT('Ctrl Pts',(28.7792711881907,50.9876270907846,62.5037034329515)) ;
#7244=CARTESIAN_POINT('Ctrl Pts',(28.6625754771975,50.723699647587,62.395520744638)) ;
#7245=CARTESIAN_POINT('Ctrl Pts',(28.5427137344922,50.4599498020535,62.2910367586478)) ;
#7246=CARTESIAN_POINT('Ctrl Pts',(28.4196910854721,50.1963788513665,62.190246712141)) ;
#7247=CARTESIAN_POINT('Ctrl Pts',(28.4165103624189,50.1895642834337,62.1876408080492)) ;
#7248=CARTESIAN_POINT('Ctrl Pts',(28.4133276054837,50.1827500045962,62.1850374381137)) ;
#7249=CARTESIAN_POINT('Ctrl Pts',(28.4101428122157,50.1759360087369,62.1824365995409)) ;
#7250=CARTESIAN_POINT('Ctrl Pts',(28.2884713276816,49.9156148757614,62.0830744546357)) ;
#7251=CARTESIAN_POINT('Ctrl Pts',(28.1639337475715,49.6552611188173,61.9874999665714)) ;
#7252=CARTESIAN_POINT('Ctrl Pts',(28.036582698318,49.394895725602,61.8957330403494)) ;
#7253=CARTESIAN_POINT('Ctrl Pts',(28.0316485060048,49.3848079176934,61.8921775481519)) ;
#7254=CARTESIAN_POINT('Ctrl Pts',(28.0267101929823,49.3747203101762,61.8886278536189)) ;
#7255=CARTESIAN_POINT('Ctrl Pts',(28.0217677725964,49.3646329259557,61.885083965985)) ;
#7256=CARTESIAN_POINT('Ctrl Pts',(27.8958077613399,49.1075509841625,61.7947662488741)) ;
#7257=CARTESIAN_POINT('Ctrl Pts',(27.7670101513391,48.8504690628023,61.7081075507894)) ;
#7258=CARTESIAN_POINT('Ctrl Pts',(27.6357590860055,48.5931578990173,61.6253810703911)) ;
#7259=CARTESIAN_POINT('Ctrl Pts',(27.6289499859684,48.579808998188,61.6210893499443)) ;
#7260=CARTESIAN_POINT('Ctrl Pts',(27.6221340729031,48.5664590689812,61.6168080801546)) ;
#7261=CARTESIAN_POINT('Ctrl Pts',(27.6153114131665,48.5531081058638,61.6125373090307)) ;
#7262=CARTESIAN_POINT('Ctrl Pts',(27.4854613464429,48.299010214641,61.5312552376969)) ;
#7263=CARTESIAN_POINT('Ctrl Pts',(27.3530838160539,48.0446012919298,61.4537190910644)) ;
#7264=CARTESIAN_POINT('Ctrl Pts',(27.2184975701169,47.7903648312084,61.380137994295)) ;
#7265=CARTESIAN_POINT('Ctrl Pts',(27.2097182717112,47.7737805380754,61.375338169461)) ;
#7266=CARTESIAN_POINT('Ctrl Pts',(27.2009292477176,47.7571963611374,61.3705549960484)) ;
#7267=CARTESIAN_POINT('Ctrl Pts',(27.1921305426904,47.7406123516807,61.3657885082833)) ;
#7268=CARTESIAN_POINT('Ctrl Pts',(27.0589583567007,47.4896062337362,61.293645665307)) ;
#7269=CARTESIAN_POINT('Ctrl Pts',(26.9239230943588,47.2387261489803,61.2255064278626)) ;
#7270=CARTESIAN_POINT('Ctrl Pts',(26.7869892778423,46.9878897404753,61.161330116392)) ;
#7271=CARTESIAN_POINT('Ctrl Pts',(26.7762121770987,46.9681481652137,61.1562792488147)) ;
#7272=CARTESIAN_POINT('Ctrl Pts',(26.7654236325356,46.9484074501541,61.1512530906726)) ;
#7273=CARTESIAN_POINT('Ctrl Pts',(26.7546236456281,46.9286675886394,61.1462516297055)) ;
#7274=CARTESIAN_POINT('Ctrl Pts',(26.6191325753522,46.6810214584507,61.0835058777729)) ;
#7275=CARTESIAN_POINT('Ctrl Pts',(26.4817445180494,46.4334531760671,61.0246143969619)) ;
#7276=CARTESIAN_POINT('Ctrl Pts',(26.3428384963142,46.1857600468481,60.9697398855416)) ;
#7277=CARTESIAN_POINT('Ctrl Pts',(26.3300701725596,46.1629919477681,60.9646957879644)) ;
#7278=CARTESIAN_POINT('Ctrl Pts',(26.3172887509827,46.1402223084084,60.9596855249274)) ;
#7279=CARTESIAN_POINT('Ctrl Pts',(26.304494549103,46.1174510138865,60.9547092356778)) ;
#7280=CARTESIAN_POINT('Ctrl Pts',(26.1670065692551,45.8727480373512,60.9012334532495)) ;
#7281=CARTESIAN_POINT('Ctrl Pts',(26.0279686867119,45.6279743432132,60.8516422216231)) ;
#7282=CARTESIAN_POINT('Ctrl Pts',(25.8874358604319,45.3830610445957,60.805979493395)) ;
#7283=CARTESIAN_POINT('',(42.1202667432172,48.5844537758935,38.6005793350086)) ;
#7284=CARTESIAN_POINT('Ctrl Pts',(32.227700990655,45.383058625274,41.2926628570961)) ;
#7285=CARTESIAN_POINT('Ctrl Pts',(32.4703899720628,45.4231928758841,40.830336338963)) ;
#7286=CARTESIAN_POINT('Ctrl Pts',(32.7630296802974,45.4870033972977,40.3986149672707)) ;
#7287=CARTESIAN_POINT('Ctrl Pts',(33.4409454321429,45.6539797372435,39.6033827587367)) ;
#7288=CARTESIAN_POINT('Ctrl Pts',(33.825622182829,45.7573388893141,39.2441406810169)) ;
#7289=CARTESIAN_POINT('Ctrl Pts',(34.9795172547242,46.0833507061678,38.384504696658)) ;
#7290=CARTESIAN_POINT('Ctrl Pts',(35.8090454233237,46.3336877227691,37.9915129106226)) ;
#7291=CARTESIAN_POINT('Ctrl Pts',(37.6274532001708,46.9107591797132,37.5234367516571)) ;
#7292=CARTESIAN_POINT('Ctrl Pts',(38.6080420354761,47.2383195349501,37.482360447981)) ;
#7293=CARTESIAN_POINT('Ctrl Pts',(40.4703782091507,47.9083523080807,37.7881695846108)) ;
#7294=CARTESIAN_POINT('Ctrl Pts',(41.3401309150115,48.2450338483642,38.1158005542573)) ;
#7295=CARTESIAN_POINT('Ctrl Pts',(42.1202667432172,48.5844537758935,38.6005793350086)) ;
#7296=CARTESIAN_POINT('',(42.1626024098661,48.6029307720944,38.627181180176)) ;
#7297=CARTESIAN_POINT('Origin',(60.4279175216359,48.3752007879039,9.69543902564879)) ;
#7298=CARTESIAN_POINT('',(54.0630686773494,55.0677871747466,51.2065737916888)) ;
#7299=CARTESIAN_POINT('Ctrl Pts',(42.1626024098661,48.6029307720944,38.6271811801759)) ;
#7300=CARTESIAN_POINT('Ctrl Pts',(42.5799907523713,48.785356686239,38.8907831019043)) ;
#7301=CARTESIAN_POINT('Ctrl Pts',(42.9898183927608,48.9676174488035,39.1659926614565)) ;
#7302=CARTESIAN_POINT('Ctrl Pts',(44.333178737041,49.5650439193917,40.0680928914892)) ;
#7303=CARTESIAN_POINT('Ctrl Pts',(45.5875732346236,50.16247038998,41.0902945761112)) ;
#7304=CARTESIAN_POINT('Ctrl Pts',(46.8419677322063,50.7598968605682,42.1124962607332)) ;
#7305=CARTESIAN_POINT('Ctrl Pts',(47.996694331525,51.3573233311564,43.2460783355894)) ;
#7306=CARTESIAN_POINT('Ctrl Pts',(49.1514209308438,51.9547498017447,44.3796604104456)) ;
#7307=CARTESIAN_POINT('Ctrl Pts',(50.1966279116985,52.5521762723329,45.6149515529632)) ;
#7308=CARTESIAN_POINT('Ctrl Pts',(51.2418348925531,53.1496027429211,46.8502426954807)) ;
#7309=CARTESIAN_POINT('Ctrl Pts',(52.1686049175126,53.7470292135094,48.176703837183)) ;
#7310=CARTESIAN_POINT('Ctrl Pts',(53.0953749424721,54.3444556840976,49.5031649788854)) ;
#7311=CARTESIAN_POINT('Ctrl Pts',(53.8958011364534,54.9418821546858,50.9094792210085)) ;
#7312=CARTESIAN_POINT('Ctrl Pts',(53.9801273110062,55.0048219850164,51.0576366665657)) ;
#7313=CARTESIAN_POINT('Ctrl Pts',(54.0630686773494,55.0677871747466,51.2065737916888)) ;
#7314=CARTESIAN_POINT('',(54.0872831542006,55.0862551252693,51.2503188022344)) ;
#7315=CARTESIAN_POINT('Origin',(82.7833587713902,55.5110797216523,35.2300331498311)) ;
#7316=CARTESIAN_POINT('Ctrl Pts',(54.0872831542006,55.0862551252692,51.2503188022345)) ;
#7317=CARTESIAN_POINT('Ctrl Pts',(54.3470010643438,55.2861476150251,51.7251031936918)) ;
#7318=CARTESIAN_POINT('Ctrl Pts',(54.5509877839354,55.4856143511658,52.2287777171693)) ;
#7319=CARTESIAN_POINT('Ctrl Pts',(54.8490787537451,55.8948726679074,53.3113250710519)) ;
#7320=CARTESIAN_POINT('Ctrl Pts',(54.9333764062709,56.1030296514257,53.8897438782962)) ;
#7321=CARTESIAN_POINT('Ctrl Pts',(54.9633976722849,56.6395227887269,55.4316582479349)) ;
#7322=CARTESIAN_POINT('Ctrl Pts',(54.7851691784216,56.9553075668517,56.3910586193405)) ;
#7323=CARTESIAN_POINT('Ctrl Pts',(54.0695245392049,57.5027527547765,58.1177679371648)) ;
#7324=CARTESIAN_POINT('Ctrl Pts',(53.5665957257014,57.7356391827932,58.8811489132992)) ;
#7325=CARTESIAN_POINT('Ctrl Pts',(52.4516508982578,58.0583686966731,60.0088645791411)) ;
#7326=CARTESIAN_POINT('Ctrl Pts',(51.9093090058447,58.1679507066731,60.4197637200829)) ;
#7327=CARTESIAN_POINT('Ctrl Pts',(50.8007524922932,58.3023925205291,61.0277068918718)) ;
#7328=CARTESIAN_POINT('Ctrl Pts',(50.2547155520565,58.3364158765144,61.2439951250786)) ;
#7329=CARTESIAN_POINT('Ctrl Pts',(49.6868966603788,58.3353824278239,61.3897862372793)) ;
#7330=CARTESIAN_POINT('Ctrl Pts',(34.1981770821883,45.3830585852922,34.9045538815956)) ;
#7331=CARTESIAN_POINT('Ctrl Pts',(35.7385556831727,45.9804850758286,35.4001920200424)) ;
#7332=CARTESIAN_POINT('Ctrl Pts',(37.2266315807177,46.5779115664506,36.0358440646385)) ;
#7333=CARTESIAN_POINT('Ctrl Pts',(38.7147074283626,47.1753380370388,36.6714960879191)) ;
#7334=CARTESIAN_POINT('Ctrl Pts',(40.1377848374042,47.772764507627,37.4417388489498)) ;
#7335=CARTESIAN_POINT('Ctrl Pts',(41.5608622464458,48.3701909782153,38.2119816099806)) ;
#7336=CARTESIAN_POINT('Ctrl Pts',(42.9068000221931,48.9676174488035,39.1102436691043)) ;
#7337=CARTESIAN_POINT('Ctrl Pts',(44.2527377979404,49.5650439193917,40.008505728228)) ;
#7338=CARTESIAN_POINT('Ctrl Pts',(45.5100528738551,50.16247038998,41.0271234302745)) ;
#7339=CARTESIAN_POINT('Ctrl Pts',(46.7673679497698,50.7598968605682,42.045741132321)) ;
#7340=CARTESIAN_POINT('Ctrl Pts',(47.9253333569409,51.3573233311564,43.176023990211)) ;
#7341=CARTESIAN_POINT('Ctrl Pts',(49.083298764112,51.9547498017447,44.3063068481009)) ;
#7342=CARTESIAN_POINT('Ctrl Pts',(50.1320351499726,52.5521762723329,45.5386116870173)) ;
#7343=CARTESIAN_POINT('Ctrl Pts',(51.1807715358333,53.1496027429211,46.7709165259337)) ;
#7344=CARTESIAN_POINT('Ctrl Pts',(52.1113314513134,53.7470292135094,48.0947297554893)) ;
#7345=CARTESIAN_POINT('Ctrl Pts',(53.0418913667935,54.3444556840976,49.4185429850449)) ;
#7346=CARTESIAN_POINT('Ctrl Pts',(53.8463356028003,54.9418821546858,50.8225702975286)) ;
#7347=CARTESIAN_POINT('Ctrl Pts',(54.6507798388072,55.5393086252741,52.2265976100123)) ;
#7348=CARTESIAN_POINT('Ctrl Pts',(55.3222451607582,56.1367350958623,53.6988603394401)) ;
#7349=CARTESIAN_POINT('Ctrl Pts',(55.9937104827092,56.7341615664505,55.1711230688678)) ;
#7350=CARTESIAN_POINT('Ctrl Pts',(56.5264681852295,57.3315880370388,56.6990603887373)) ;
#7351=CARTESIAN_POINT('Ctrl Pts',(56.9952159947389,57.857234776835,58.0434187497113)) ;
#7352=CARTESIAN_POINT('Ctrl Pts',(57.3532241458314,58.3831186720347,59.421407891683)) ;
#7353=CARTESIAN_POINT('Ctrl Pts',(25.7002097997771,45.3830585852922,61.058608161473)) ;
#7354=CARTESIAN_POINT('Ctrl Pts',(26.0314134558695,45.9804850758286,61.1613615482693)) ;
#7355=CARTESIAN_POINT('Ctrl Pts',(26.3517233687144,46.5779115664506,61.2942362262193)) ;
#7356=CARTESIAN_POINT('Ctrl Pts',(26.6720332708182,47.1753380370388,61.4271108997137)) ;
#7357=CARTESIAN_POINT('Ctrl Pts',(26.9787166592112,47.772764507627,61.588973222463)) ;
#7358=CARTESIAN_POINT('Ctrl Pts',(27.2854000476041,48.3701909782152,61.7508355452123)) ;
#7359=CARTESIAN_POINT('Ctrl Pts',(27.57584040775,48.9676174488035,61.9403045649499)) ;
#7360=CARTESIAN_POINT('Ctrl Pts',(27.8662807678958,49.5650439193917,62.1297735846875)) ;
#7361=CARTESIAN_POINT('Ctrl Pts',(28.1380001650482,50.16247038998,62.345232818542)) ;
#7362=CARTESIAN_POINT('Ctrl Pts',(28.4097195622005,50.7598968605682,62.5606920523965)) ;
#7363=CARTESIAN_POINT('Ctrl Pts',(28.6603997822684,51.3573233311564,62.8003032781533)) ;
#7364=CARTESIAN_POINT('Ctrl Pts',(28.9110800023363,51.9547498017447,63.0399145039102)) ;
#7365=CARTESIAN_POINT('Ctrl Pts',(29.1385823300695,52.5521762723329,63.3016334430758)) ;
#7366=CARTESIAN_POINT('Ctrl Pts',(29.3660846578027,53.1496027429211,63.5633523822414)) ;
#7367=CARTESIAN_POINT('Ctrl Pts',(29.568468123556,53.7470292135094,63.8449461411063)) ;
#7368=CARTESIAN_POINT('Ctrl Pts',(29.7708515893093,54.3444556840976,64.1265398999712)) ;
#7369=CARTESIAN_POINT('Ctrl Pts',(29.9463895287114,54.9418821546858,64.4256060198719)) ;
#7370=CARTESIAN_POINT('Ctrl Pts',(30.1219274681135,55.5393086252741,64.7246721397726)) ;
#7371=CARTESIAN_POINT('Ctrl Pts',(30.2691222533582,56.1367350958623,65.0386590940219)) ;
#7372=CARTESIAN_POINT('Ctrl Pts',(30.4163170386029,56.7341615664506,65.3526460482712)) ;
#7373=CARTESIAN_POINT('Ctrl Pts',(30.5339128556821,57.3315880370388,65.6788750108841)) ;
#7374=CARTESIAN_POINT('Ctrl Pts',(30.6373797439176,57.8572347768351,65.965908142268)) ;
#7375=CARTESIAN_POINT('Ctrl Pts',(30.7171914921666,58.3831186720347,66.2603966824774)) ;
#7376=CARTESIAN_POINT('',(31.0031929801423,58.3830537363178,66.1869634870219)) ;
#7377=CARTESIAN_POINT('Ctrl Pts',(25.7914429954097,45.3830674541108,60.7777739865218)) ;
#7378=CARTESIAN_POINT('Ctrl Pts',(25.8011520792638,45.3999249614349,60.7807915393391)) ;
#7379=CARTESIAN_POINT('Ctrl Pts',(25.810991377335,45.4170195560983,60.783870696162)) ;
#7380=CARTESIAN_POINT('Ctrl Pts',(25.8305174186758,45.4509660823352,60.7900238219679)) ;
#7381=CARTESIAN_POINT('Ctrl Pts',(25.8402729717326,45.4679374856688,60.793119176787)) ;
#7382=CARTESIAN_POINT('Ctrl Pts',(25.8695171038289,45.5188462146264,60.8024615163315)) ;
#7383=CARTESIAN_POINT('Ctrl Pts',(25.8889831559,45.5527780591986,60.8087647757947)) ;
#7384=CARTESIAN_POINT('Ctrl Pts',(25.9472902038144,45.6545524513439,60.8278988611025)) ;
#7385=CARTESIAN_POINT('Ctrl Pts',(25.9860400862657,45.7223738576064,60.8409540084028)) ;
#7386=CARTESIAN_POINT('Ctrl Pts',(26.073308227283,45.8755455989771,60.8711208490251)) ;
#7387=CARTESIAN_POINT('Ctrl Pts',(26.1217552892988,45.9608834226822,60.8884072085208)) ;
#7388=CARTESIAN_POINT('Ctrl Pts',(26.1983712336257,46.0963466756247,60.9166009893408)) ;
#7389=CARTESIAN_POINT('Ctrl Pts',(26.2266807713393,46.1464973799217,60.9272060830759)) ;
#7390=CARTESIAN_POINT('Ctrl Pts',(26.3853710207649,46.4282028809684,60.9877078420715)) ;
#7391=CARTESIAN_POINT('Ctrl Pts',(26.5143766908135,46.6594344485567,61.0409057065247)) ;
#7392=CARTESIAN_POINT('Ctrl Pts',(26.6632621942723,46.9296827699029,61.1070233668255)) ;
#7393=CARTESIAN_POINT('Ctrl Pts',(26.6847644468963,46.968795042416,61.1166890996772)) ;
#7394=CARTESIAN_POINT('Ctrl Pts',(26.8390184511679,47.2499758749385,61.1868717873152)) ;
#7395=CARTESIAN_POINT('Ctrl Pts',(26.969967923605,47.491854191672,61.2509483646101)) ;
#7396=CARTESIAN_POINT('Ctrl Pts',(27.2490607324932,48.0143150857781,61.397343778151)) ;
#7397=CARTESIAN_POINT('Ctrl Pts',(27.396430725844,48.2952954282289,61.4808850637674)) ;
#7398=CARTESIAN_POINT('Ctrl Pts',(27.5496308033829,48.5931204307081,61.5744432491943)) ;
#7399=CARTESIAN_POINT('Ctrl Pts',(27.5583656313921,48.6101204742725,61.5798012478732)) ;
#7400=CARTESIAN_POINT('Ctrl Pts',(27.7025370493161,48.891036215033,61.6686290067572)) ;
#7401=CARTESIAN_POINT('Ctrl Pts',(27.8355404157494,49.1549226796748,61.7563011398068)) ;
#7402=CARTESIAN_POINT('Ctrl Pts',(27.9686046174867,49.4249376060055,61.8499871777608)) ;
#7403=CARTESIAN_POINT('Ctrl Pts',(27.9714928098665,49.4308011237539,61.8520235913532)) ;
#7404=CARTESIAN_POINT('Ctrl Pts',(28.1073185789858,49.7066812295575,61.9479300993227)) ;
#7405=CARTESIAN_POINT('Ctrl Pts',(28.2374330061678,49.9768666464288,62.0460374326432)) ;
#7406=CARTESIAN_POINT('Ctrl Pts',(28.3670465485902,50.252704329167,62.150317347732)) ;
#7407=CARTESIAN_POINT('Ctrl Pts',(28.3695621457808,50.2580605419637,62.1523438352739)) ;
#7408=CARTESIAN_POINT('Ctrl Pts',(28.4965433518478,50.5285623062338,62.2547661851058)) ;
#7409=CARTESIAN_POINT('Ctrl Pts',(28.6179571450043,50.794089282034,62.3590112370404)) ;
#7410=CARTESIAN_POINT('Ctrl Pts',(28.7437567626043,51.0767673302899,62.4739538912658)) ;
#7411=CARTESIAN_POINT('Ctrl Pts',(28.7511947182076,51.0935097128497,62.4807764467365)) ;
#7412=CARTESIAN_POINT('Ctrl Pts',(28.8213209690217,51.2516332986659,62.5453515762971)) ;
#7413=CARTESIAN_POINT('Ctrl Pts',(28.8831980925262,51.3931664826133,62.6042351612115)) ;
#7414=CARTESIAN_POINT('Ctrl Pts',(28.9927392868846,51.6479675595721,62.7119639549746)) ;
#7415=CARTESIAN_POINT('Ctrl Pts',(29.0407823804013,51.761231940684,62.7604712205008)) ;
#7416=CARTESIAN_POINT('Ctrl Pts',(29.0999524386712,51.9026374456286,62.8218017972563)) ;
#7417=CARTESIAN_POINT('Ctrl Pts',(29.1117004986403,51.9308091085127,62.8340587121007)) ;
#7418=CARTESIAN_POINT('Ctrl Pts',(29.2409148910853,52.2417252333157,62.9697539796517)) ;
#7419=CARTESIAN_POINT('Ctrl Pts',(29.3543479666627,52.5241195492494,63.0969791494064)) ;
#7420=CARTESIAN_POINT('Ctrl Pts',(29.5529056802919,53.0381974993347,63.3349410676277)) ;
#7421=CARTESIAN_POINT('Ctrl Pts',(29.6393958238015,53.2697333986876,63.4444393238498)) ;
#7422=CARTESIAN_POINT('Ctrl Pts',(29.7413330349859,53.552225996692,63.5808721174967)) ;
#7423=CARTESIAN_POINT('Ctrl Pts',(29.7595762333489,53.6031771340243,63.6055921287614)) ;
#7424=CARTESIAN_POINT('Ctrl Pts',(29.8558751791141,53.8742457620922,63.7377058663455)) ;
#7425=CARTESIAN_POINT('Ctrl Pts',(29.9313616882554,54.0945463050605,63.8470320121601)) ;
#7426=CARTESIAN_POINT('Ctrl Pts',(30.0246196339593,54.3774106831917,63.9897636197812)) ;
#7427=CARTESIAN_POINT('Ctrl Pts',(30.044986179155,54.4398806254201,64.0214329924024)) ;
#7428=CARTESIAN_POINT('Ctrl Pts',(30.1325125522462,54.711432139291,64.1597267018904)) ;
#7429=CARTESIAN_POINT('Ctrl Pts',(30.197395884353,54.9205828276718,64.2679757139459)) ;
#7430=CARTESIAN_POINT('Ctrl Pts',(30.2814951271688,55.2033684329563,64.4163117644225)) ;
#7431=CARTESIAN_POINT('Ctrl Pts',(30.3031271039968,55.2772338818111,64.4552407854699)) ;
#7432=CARTESIAN_POINT('Ctrl Pts',(30.3813145103917,55.5485088102159,64.5988369765006)) ;
#7433=CARTESIAN_POINT('Ctrl Pts',(30.4357819827863,55.7457837763599,64.7045566063819)) ;
#7434=CARTESIAN_POINT('Ctrl Pts',(30.5102987190112,56.0282588904766,64.8576993333359)) ;
#7435=CARTESIAN_POINT('Ctrl Pts',(30.5323283405607,56.1134884206126,64.904136632693)) ;
#7436=CARTESIAN_POINT('Ctrl Pts',(30.6009132913455,56.3844426290971,65.0524814877124)) ;
#7437=CARTESIAN_POINT('Ctrl Pts',(30.6456844427088,56.5701302611241,65.1550649798116)) ;
#7438=CARTESIAN_POINT('Ctrl Pts',(30.7104181164342,56.8526653483016,65.3125514864397)) ;
#7439=CARTESIAN_POINT('Ctrl Pts',(30.7319926277606,56.9494716030842,65.3667618614678)) ;
#7440=CARTESIAN_POINT('Ctrl Pts',(30.7906879595627,57.2204413601012,65.5192013282813)) ;
#7441=CARTESIAN_POINT('Ctrl Pts',(30.8264612285573,57.3946576755349,65.6180227168432)) ;
#7442=CARTESIAN_POINT('Ctrl Pts',(30.8812470754923,57.6774250653632,65.7794891180073)) ;
#7443=CARTESIAN_POINT('Ctrl Pts',(30.9014891525821,57.78593964127,65.8417091024842)) ;
#7444=CARTESIAN_POINT('Ctrl Pts',(30.9258050052165,57.9216227418847,65.9197805890467)) ;
#7445=CARTESIAN_POINT('Ctrl Pts',(30.9306139332621,57.9487278912589,65.9353936621802)) ;
#7446=CARTESIAN_POINT('Ctrl Pts',(30.9472893957238,58.0436810159814,65.9901451420611)) ;
#7447=CARTESIAN_POINT('Ctrl Pts',(30.9589006933603,58.1115399743055,66.029375203218)) ;
#7448=CARTESIAN_POINT('Ctrl Pts',(30.9758575565952,58.2133484522822,66.0883678261757)) ;
#7449=CARTESIAN_POINT('Ctrl Pts',(30.981432705011,58.2472850649058,66.1080549429286)) ;
#7450=CARTESIAN_POINT('Ctrl Pts',(30.9896801854667,58.2981973836579,66.1376218550297)) ;
#7451=CARTESIAN_POINT('Ctrl Pts',(30.9924101383193,58.3151693899103,66.1474835319424)) ;
#7452=CARTESIAN_POINT('Ctrl Pts',(30.995859334791,58.3367668565652,66.1600394167404)) ;
#7453=CARTESIAN_POINT('Ctrl Pts',(30.9965978053812,58.3413999128707,66.1627332693675)) ;
#7454=CARTESIAN_POINT('Ctrl Pts',(30.9993038725722,58.3584108602041,66.1726255449783)) ;
#7455=CARTESIAN_POINT('Ctrl Pts',(31.0012638847202,58.370797523339,66.1798314240518)) ;
#7456=CARTESIAN_POINT('Ctrl Pts',(31.0031926666446,58.3830508753323,66.1869623392087)) ;
#7457=CARTESIAN_POINT('',(49.6868966603789,58.3831162793798,61.3897862372794)) ;
#7458=CARTESIAN_POINT('Ctrl Pts',(31.00318876339,58.3830900980198,66.1869470825038)) ;
#7459=CARTESIAN_POINT('Ctrl Pts',(34.1171400804529,58.383105259385,65.3874202747358)) ;
#7460=CARTESIAN_POINT('Ctrl Pts',(37.2310913975658,58.3831073991803,64.5878934669549)) ;
#7461=CARTESIAN_POINT('Ctrl Pts',(43.4589940299001,58.3831134572106,62.9888398518788)) ;
#7462=CARTESIAN_POINT('Ctrl Pts',(46.5729453451396,58.3831150235129,62.1893130445791)) ;
#7463=CARTESIAN_POINT('Ctrl Pts',(49.6868966603789,58.3831162793797,61.3897862372793)) ;
#7464=CARTESIAN_POINT('',(54.0631310962388,55.1047242171091,51.2065390655857)) ;
#7465=CARTESIAN_POINT('Ctrl Pts',(49.6868966603789,58.3831162793797,61.3897862372793)) ;
#7466=CARTESIAN_POINT('Ctrl Pts',(50.2581195512456,58.3831165097558,61.2431211266348)) ;
#7467=CARTESIAN_POINT('Ctrl Pts',(50.8072353354247,58.3477204548742,61.0251267819229)) ;
#7468=CARTESIAN_POINT('Ctrl Pts',(51.9220081649887,58.2097833704152,60.4116400136406)) ;
#7469=CARTESIAN_POINT('Ctrl Pts',(52.4670772856615,58.0979491851444,59.9965228800265)) ;
#7470=CARTESIAN_POINT('Ctrl Pts',(53.5816676879437,57.7707078254696,58.8613539461653)) ;
#7471=CARTESIAN_POINT('Ctrl Pts',(54.0821618785496,57.5360202457534,58.095728852092)) ;
#7472=CARTESIAN_POINT('Ctrl Pts',(54.7917779132289,56.9856758817168,56.3656833294583)) ;
#7473=CARTESIAN_POINT('Ctrl Pts',(54.9665090756242,56.6687344805943,55.4052128724977)) ;
#7474=CARTESIAN_POINT('Ctrl Pts',(54.9304672122228,56.1294192803767,53.8587960473992)) ;
#7475=CARTESIAN_POINT('Ctrl Pts',(54.8428115777871,55.9194276565172,53.2765902560065)) ;
#7476=CARTESIAN_POINT('Ctrl Pts',(54.5365399857756,55.5068628236254,52.1882811657281)) ;
#7477=CARTESIAN_POINT('Ctrl Pts',(54.3279790102755,55.3059550653477,51.6825934226883)) ;
#7478=CARTESIAN_POINT('Ctrl Pts',(54.0631310962388,55.104724217109,51.2065390655857)) ;
#7479=CARTESIAN_POINT('',(42.1626405421888,48.6398835186857,38.6271207819479)) ;
#7480=CARTESIAN_POINT('Ctrl Pts',(42.1626405421888,48.6398835186857,38.6271207819478)) ;
#7481=CARTESIAN_POINT('Ctrl Pts',(42.5377822297253,48.8038201453524,38.8639658740149)) ;
#7482=CARTESIAN_POINT('Ctrl Pts',(42.9067999896793,48.9676174488035,39.1102437175222)) ;
#7483=CARTESIAN_POINT('Ctrl Pts',(44.2527377631881,49.5650439193917,40.0085057751427)) ;
#7484=CARTESIAN_POINT('Ctrl Pts',(45.5100528370125,50.16247038998,41.0271234754859)) ;
#7485=CARTESIAN_POINT('Ctrl Pts',(46.7673679108369,50.7598968605682,42.0457411758291)) ;
#7486=CARTESIAN_POINT('Ctrl Pts',(47.9253333160839,51.3573233311564,43.1760240318301)) ;
#7487=CARTESIAN_POINT('Ctrl Pts',(49.0832987213308,51.9547498017447,44.3063068878311)) ;
#7488=CARTESIAN_POINT('Ctrl Pts',(50.1320351054498,52.5521762723329,45.5386117246891)) ;
#7489=CARTESIAN_POINT('Ctrl Pts',(51.1807714895688,53.1496027429211,46.770916561547)) ;
#7490=CARTESIAN_POINT('Ctrl Pts',(52.1113314035046,53.7470292135094,48.0947297888923)) ;
#7491=CARTESIAN_POINT('Ctrl Pts',(53.0418913174403,54.3444556840976,49.4185430162376)) ;
#7492=CARTESIAN_POINT('Ctrl Pts',(53.8463355521134,54.9418821546858,50.8225703263779)) ;
#7493=CARTESIAN_POINT('Ctrl Pts',(53.9559426933193,55.0232827101246,51.0138718647649)) ;
#7494=CARTESIAN_POINT('Ctrl Pts',(54.0631310962388,55.1047242171091,51.2065390655857)) ;
#7495=CARTESIAN_POINT('Ctrl Pts',(42.1626405421888,48.6398835186857,38.6271207819478)) ;
#7496=CARTESIAN_POINT('Ctrl Pts',(41.7048656670768,48.4398362531006,38.3381053617905)) ;
#7497=CARTESIAN_POINT('Ctrl Pts',(41.2147380839232,48.2402511664186,38.1029380979704)) ;
#7498=CARTESIAN_POINT('Ctrl Pts',(40.1532298521113,47.8311033708305,37.7379112181705)) ;
#7499=CARTESIAN_POINT('Ctrl Pts',(39.581810011503,47.6231195575043,37.6177136594679)) ;
#7500=CARTESIAN_POINT('Ctrl Pts',(38.0454077153629,47.0862679673289,37.4910821825243)) ;
#7501=CARTESIAN_POINT('Ctrl Pts',(37.0765536712975,46.7703269230101,37.6087916756144)) ;
#7502=CARTESIAN_POINT('Ctrl Pts',(35.3073691230138,46.2216256025067,38.2152157232851)) ;
#7503=CARTESIAN_POINT('Ctrl Pts',(34.5136933172468,45.987905739686,38.6696648884542)) ;
#7504=CARTESIAN_POINT('Ctrl Pts',(33.3188969657845,45.6640068127921,39.7118246364103)) ;
#7505=CARTESIAN_POINT('Ctrl Pts',(32.8755155146971,45.5539383581279,40.2266046313311)) ;
#7506=CARTESIAN_POINT('Ctrl Pts',(32.1996537162509,45.4179657700952,41.2939599752307)) ;
#7507=CARTESIAN_POINT('Ctrl Pts',(31.9494597369605,45.3830586252741,41.8253945852044)) ;
#7508=CARTESIAN_POINT('Ctrl Pts',(31.768269675766,45.3830586252741,42.3830402536426)) ;
#7509=CARTESIAN_POINT('Origin',(38.4256652898321,45.3822493559848,44.5461592142672)) ;
#7510=CARTESIAN_POINT('',(42.1626405421888,45.3822493559848,38.6271207819479)) ;
#7511=CARTESIAN_POINT('Origin',(23.47768801576,45.3822493559848,68.2224337400008)) ;
#7512=CARTESIAN_POINT('',(54.0631310962388,45.3822493559848,51.2065390655857)) ;
#7513=CARTESIAN_POINT('Origin',(47.9460674476988,45.3822493559848,54.6097041100275)) ;
#7514=CARTESIAN_POINT('',(49.6868966603788,45.3822493559848,61.3897862372794)) ;
#7515=CARTESIAN_POINT('Origin',(30.7171869358834,45.3822493559848,66.2603798709065)) ;
#7516=CARTESIAN_POINT('Ctrl Pts',(30.8134080024022,57.8271591829153,66.2356745000382)) ;
#7517=CARTESIAN_POINT('Ctrl Pts',(30.8134911684381,57.8726762309135,66.2356531466295)) ;
#7518=CARTESIAN_POINT('Ctrl Pts',(30.8175149348243,57.9189559198363,66.2346200189886)) ;
#7519=CARTESIAN_POINT('Ctrl Pts',(30.8339069695655,58.0070760891654,66.2304112598029)) ;
#7520=CARTESIAN_POINT('Ctrl Pts',(30.8464719817728,58.051172006285,66.2271851130226)) ;
#7521=CARTESIAN_POINT('Ctrl Pts',(30.8814813724371,58.1280396083484,66.2181962292831)) ;
#7522=CARTESIAN_POINT('Ctrl Pts',(30.9017034964742,58.1581206857625,66.2130040703033)) ;
#7523=CARTESIAN_POINT('Ctrl Pts',(30.9363795480004,58.1912258389426,66.2041007735077)) ;
#7524=CARTESIAN_POINT('Ctrl Pts',(30.9500225532736,58.2011509267379,66.200597845129)) ;
#7525=CARTESIAN_POINT('Ctrl Pts',(30.9779076696627,58.2136664809671,66.1934381641254)) ;
#7526=CARTESIAN_POINT('Ctrl Pts',(30.9913762520981,58.2169696033494,66.1899800199146)) ;
#7527=CARTESIAN_POINT('Ctrl Pts',(31.005319018212,58.2172758076354,66.1864001260282)) ;
#7528=CARTESIAN_POINT('Ctrl Pts',(31.0031885544775,58.3830247512579,66.1869471361434)) ;
#7529=CARTESIAN_POINT('Ctrl Pts',(30.9963789496716,58.3830247228379,66.1886955454916)) ;
#7530=CARTESIAN_POINT('Ctrl Pts',(30.9896247806473,58.3837424765067,66.1904297213503)) ;
#7531=CARTESIAN_POINT('Ctrl Pts',(30.9758330390786,58.3866521090712,66.1939708387241)) ;
#7532=CARTESIAN_POINT('Ctrl Pts',(30.9689139763115,58.3889169428641,66.1957473521001)) ;
#7533=CARTESIAN_POINT('Ctrl Pts',(30.9468729562285,58.3985444430763,66.2014065242041)) ;
#7534=CARTESIAN_POINT('Ctrl Pts',(30.9330378733326,58.4085611720431,66.2049587697639)) ;
#7535=CARTESIAN_POINT('Ctrl Pts',(30.8990356285796,58.4411881110303,66.2136890623845)) ;
#7536=CARTESIAN_POINT('Ctrl Pts',(30.8795612593899,58.4701790972771,66.2186892305213)) ;
#7537=CARTESIAN_POINT('Ctrl Pts',(30.8454692246162,58.5450324121023,66.2274425773009)) ;
#7538=CARTESIAN_POINT('Ctrl Pts',(30.8332143405224,58.5884045335537,66.2305890968203)) ;
#7539=CARTESIAN_POINT('Ctrl Pts',(30.8172539293367,58.675275268205,66.2346870339127)) ;
#7540=CARTESIAN_POINT('Ctrl Pts',(30.8134073328871,58.721038685519,66.2356746719405)) ;
#7541=CARTESIAN_POINT('Ctrl Pts',(30.8134076051844,58.7660385537515,66.2356746020264)) ;
#7542=CARTESIAN_POINT('Ctrl Pts',(31.0173239967825,58.2943663992286,66.2313141867391)) ;
#7543=CARTESIAN_POINT('Ctrl Pts',(30.8272744005839,58.2924602039142,66.2803148338344)) ;
#7544=CARTESIAN_POINT('Ctrl Pts',(30.8666087426552,58.191081348463,66.4437121508651)) ;
#7545=CARTESIAN_POINT('Ctrl Pts',(30.9338538642454,57.7522999682189,65.9152482091109)) ;
#7546=CARTESIAN_POINT('Ctrl Pts',(30.7458602690527,57.7503889246408,65.9722138304264)) ;
#7547=CARTESIAN_POINT('Ctrl Pts',(30.7920398310218,57.6489874077046,66.1339482282166)) ;
#7548=CARTESIAN_POINT('Ctrl Pts',(30.8306212790909,57.21110331024,65.6049265502847)) ;
#7549=CARTESIAN_POINT('Ctrl Pts',(30.6451794827466,57.2091968025836,65.6697195946995)) ;
#7550=CARTESIAN_POINT('Ctrl Pts',(30.6981068121273,57.1078632090985,65.8294151776596)) ;
#7551=CARTESIAN_POINT('Ctrl Pts',(30.6474937677951,56.3997926693554,65.1514197248828)) ;
#7552=CARTESIAN_POINT('Ctrl Pts',(30.4665934227563,56.3978864499735,65.227653528776)) ;
#7553=CARTESIAN_POINT('Ctrl Pts',(30.5293754831954,56.2965290899915,65.3836047172742)) ;
#7554=CARTESIAN_POINT('Ctrl Pts',(30.581679313116,56.1295297083734,65.0020936671592)) ;
#7555=CARTESIAN_POINT('Ctrl Pts',(30.4024119119524,56.1276240321184,65.0820955068002)) ;
#7556=CARTESIAN_POINT('Ctrl Pts',(30.4684307812205,56.0262125668428,65.2366705986467)) ;
#7557=CARTESIAN_POINT('Ctrl Pts',(30.4407980320214,55.5885108130536,64.7078405549652)) ;
#7558=CARTESIAN_POINT('Ctrl Pts',(30.2650353509719,55.5866055506174,64.7952692923242)) ;
#7559=CARTESIAN_POINT('Ctrl Pts',(30.3374787224399,55.485272016298,64.9469891274856)) ;
#7560=CARTESIAN_POINT('Ctrl Pts',(30.3657746842047,55.3179011606876,64.5629812644996)) ;
#7561=CARTESIAN_POINT('Ctrl Pts',(30.1918780290501,55.3159940909446,64.6540658012614)) ;
#7562=CARTESIAN_POINT('Ctrl Pts',(30.2674776517272,55.2146518759856,64.8042324556393)) ;
#7563=CARTESIAN_POINT('Ctrl Pts',(30.2065304249104,54.7764805321232,64.2778126981827)) ;
#7564=CARTESIAN_POINT('Ctrl Pts',(30.0365957838312,54.7745728258419,64.3760973749008)) ;
#7565=CARTESIAN_POINT('Ctrl Pts',(30.118383848403,54.673110454093,64.5229064486545)) ;
#7566=CARTESIAN_POINT('Ctrl Pts',(30.1222957661658,54.5052712784508,64.137525239918)) ;
#7567=CARTESIAN_POINT('Ctrl Pts',(29.954464616695,54.5033650628297,64.2393538637961)) ;
#7568=CARTESIAN_POINT('Ctrl Pts',(30.0393485098831,54.4020271817821,64.3844774616171)) ;
#7569=CARTESIAN_POINT('Ctrl Pts',(29.9455876310585,53.9638812711027,63.8631253385711)) ;
#7570=CARTESIAN_POINT('Ctrl Pts',(29.7821625432364,53.9619749130418,63.9718859746674)) ;
#7571=CARTESIAN_POINT('Ctrl Pts',(29.873035343762,53.860610246182,64.113318337735)) ;
#7572=CARTESIAN_POINT('Ctrl Pts',(29.8529205076406,53.6935003224001,63.7286963367937)) ;
#7573=CARTESIAN_POINT('Ctrl Pts',(29.691807035817,53.6915946088883,63.8408543226021)) ;
#7574=CARTESIAN_POINT('Ctrl Pts',(29.7856090795231,53.5901950776356,63.9803370049613)) ;
#7575=CARTESIAN_POINT('Ctrl Pts',(29.6594824549092,53.1525885953591,63.4661043934883)) ;
#7576=CARTESIAN_POINT('Ctrl Pts',(29.503200788466,53.1506832358119,63.5848997167274)) ;
#7577=CARTESIAN_POINT('Ctrl Pts',(29.6027738980047,53.0493503316824,63.7203702363143)) ;
#7578=CARTESIAN_POINT('Ctrl Pts',(29.5587376511048,52.8821999703706,63.3379585752569)) ;
#7579=CARTESIAN_POINT('Ctrl Pts',(29.4049714652684,52.8802927777264,63.4599930285515)) ;
#7580=CARTESIAN_POINT('Ctrl Pts',(29.5073500068726,52.7789455602911,63.5933458219226)) ;
#7581=CARTESIAN_POINT('Ctrl Pts',(29.3491929541791,52.3415574725492,63.0879698629551)) ;
#7582=CARTESIAN_POINT('Ctrl Pts',(29.2006595660773,52.3396495857196,63.216327225387)) ;
#7583=CARTESIAN_POINT('Ctrl Pts',(29.3084773791931,52.2381712237465,63.3452240787661)) ;
#7584=CARTESIAN_POINT('Ctrl Pts',(29.2404444313661,52.0708923183226,62.9662055967095)) ;
#7585=CARTESIAN_POINT('Ctrl Pts',(29.0946348929149,52.0689860210687,63.0976434808219)) ;
#7586=CARTESIAN_POINT('Ctrl Pts',(29.2051790309548,51.967651026395,63.2243189994837)) ;
#7587=CARTESIAN_POINT('Ctrl Pts',(29.0154772528091,51.5294526417487,62.7296936231344)) ;
#7588=CARTESIAN_POINT('Ctrl Pts',(28.8752935944966,51.5275461441804,62.8671172871891)) ;
#7589=CARTESIAN_POINT('Ctrl Pts',(28.9910265495215,51.4261734610189,62.9890407201091)) ;
#7590=CARTESIAN_POINT('Ctrl Pts',(28.8990062710636,51.2584285629436,62.6147037460552)) ;
#7591=CARTESIAN_POINT('Ctrl Pts',(28.761736858127,51.2565228089791,62.755039072442)) ;
#7592=CARTESIAN_POINT('Ctrl Pts',(28.8799958936779,51.155134072336,62.8745009981941)) ;
#7593=CARTESIAN_POINT('Ctrl Pts',(28.6595364145706,50.7168256230159,62.3927027901548)) ;
#7594=CARTESIAN_POINT('Ctrl Pts',(28.5282629209368,50.7149201642748,62.5386603231389)) ;
#7595=CARTESIAN_POINT('Ctrl Pts',(28.6514413554663,50.6135869790364,62.6530898469933)) ;
#7596=CARTESIAN_POINT('Ctrl Pts',(28.5364906257386,50.4462620313617,62.2856173447484)) ;
#7597=CARTESIAN_POINT('Ctrl Pts',(28.4082966641083,50.4443547062453,62.4342875276819)) ;
#7598=CARTESIAN_POINT('Ctrl Pts',(28.5338335609057,50.343001553274,62.5461074002847)) ;
#7599=CARTESIAN_POINT('Ctrl Pts',(28.283795141269,49.905609988286,62.0792556818166)) ;
#7600=CARTESIAN_POINT('Ctrl Pts',(28.1619262162133,49.9037019096497,62.2331580132732)) ;
#7601=CARTESIAN_POINT('Ctrl Pts',(28.291967471768,49.8022062837453,62.3395771372856)) ;
#7602=CARTESIAN_POINT('Ctrl Pts',(28.1542570098572,49.635040821776,61.9800832945457)) ;
#7603=CARTESIAN_POINT('Ctrl Pts',(28.0356389821241,49.6331344367361,62.1364995516978)) ;
#7604=CARTESIAN_POINT('Ctrl Pts',(28.167949142981,49.5318014383422,62.2402351417232)) ;
#7605=CARTESIAN_POINT('Ctrl Pts',(27.8892785686591,49.0942250306864,61.7900845915201)) ;
#7606=CARTESIAN_POINT('Ctrl Pts',(27.7772999871363,49.0923183862306,61.9513222262773)) ;
#7607=CARTESIAN_POINT('Ctrl Pts',(27.9138077417617,48.9909365753663,62.0494205950826)) ;
#7608=CARTESIAN_POINT('Ctrl Pts',(27.7536506015481,48.8238179925643,61.6991333239323)) ;
#7609=CARTESIAN_POINT('Ctrl Pts',(27.6450725909719,48.8219121926736,61.8626802565342)) ;
#7610=CARTESIAN_POINT('Ctrl Pts',(27.7836051589675,48.7205331729861,61.9579007407528)) ;
#7611=CARTESIAN_POINT('Ctrl Pts',(27.4769725624454,48.2823982252869,61.5259407616695)) ;
#7612=CARTESIAN_POINT('Ctrl Pts',(27.375333692239,48.2804926624883,61.6938867971212)) ;
#7613=CARTESIAN_POINT('Ctrl Pts',(27.5177502752558,48.17915824216,61.7832417812041)) ;
#7614=CARTESIAN_POINT('Ctrl Pts',(27.3358290336846,48.0114576298707,61.4436323948175)) ;
#7615=CARTESIAN_POINT('Ctrl Pts',(27.2377262624136,48.009552069624,61.6136730295645)) ;
#7616=CARTESIAN_POINT('Ctrl Pts',(27.381907086481,47.9080609643674,61.6999779551815)) ;
#7617=CARTESIAN_POINT('Ctrl Pts',(27.0484326317699,47.4697670851943,61.2879435657883)) ;
#7618=CARTESIAN_POINT('Ctrl Pts',(26.9575440003344,47.4678622559094,61.4619430611764)) ;
#7619=CARTESIAN_POINT('Ctrl Pts',(27.105282807758,47.3665093096313,61.542170867765)) ;
#7620=CARTESIAN_POINT('Ctrl Pts',(26.9025922094126,47.1991192501543,61.2147751017004)) ;
#7621=CARTESIAN_POINT('Ctrl Pts',(26.8153628578287,47.1972127705413,61.3906367503116)) ;
#7622=CARTESIAN_POINT('Ctrl Pts',(26.96475857933,47.0958808569866,61.4677612275413)) ;
#7623=CARTESIAN_POINT('Ctrl Pts',(26.6066553014126,46.6582159321358,61.0777276907649)) ;
#7624=CARTESIAN_POINT('Ctrl Pts',(26.5268521641293,46.6563091332017,61.2570830605992)) ;
#7625=CARTESIAN_POINT('Ctrl Pts',(26.6793104751995,46.5549171221787,61.3278796940087)) ;
#7626=CARTESIAN_POINT('Ctrl Pts',(26.4564442172867,46.3878930438346,61.0138098095528)) ;
#7627=CARTESIAN_POINT('Ctrl Pts',(26.3804132190556,46.3859871917477,61.1947958430729)) ;
#7628=CARTESIAN_POINT('Ctrl Pts',(26.5343309437764,46.284617201445,61.2623921487697)) ;
#7629=CARTESIAN_POINT('Ctrl Pts',(26.1525452484292,45.847008993639,60.8956077330631)) ;
#7630=CARTESIAN_POINT('Ctrl Pts',(26.0841461601336,45.8451033188968,61.0796128500728)) ;
#7631=CARTESIAN_POINT('Ctrl Pts',(26.2407723084679,45.7437666877396,61.1407241912794)) ;
#7632=CARTESIAN_POINT('Ctrl Pts',(25.9987670923634,45.5765948766442,60.8412757218746)) ;
#7633=CARTESIAN_POINT('Ctrl Pts',(25.9342268983673,45.5746876691494,61.0266727188793)) ;
#7634=CARTESIAN_POINT('Ctrl Pts',(26.0920704394477,45.4732994150099,61.0844840121749)) ;
#7635=CARTESIAN_POINT('Ctrl Pts',(25.8432056478439,45.3060601767044,60.7917538220346)) ;
#7636=CARTESIAN_POINT('Ctrl Pts',(25.7825741591705,45.3041537286489,60.9784198972454)) ;
#7637=CARTESIAN_POINT('Ctrl Pts',(25.9415364981948,45.2027271666488,61.0328961571237)) ;
#7638=CARTESIAN_POINT('Ctrl Pts',(25.6853615766559,45.1993067880442,60.7456299070416)) ;
#7639=CARTESIAN_POINT('Ctrl Pts',(25.629734117304,45.2022941676425,60.9315956388122)) ;
#7640=CARTESIAN_POINT('Ctrl Pts',(25.4693419487448,45.3026134137914,60.8880411536154)) ;
#7641=CARTESIAN_POINT('Ctrl Pts',(25.8489500846755,45.4820412744461,60.7939313563783)) ;
#7642=CARTESIAN_POINT('Ctrl Pts',(25.7892537891377,45.4850270680332,60.9786815820694)) ;
#7643=CARTESIAN_POINT('Ctrl Pts',(25.629811962671,45.5853439255465,60.9316167777176)) ;
#7644=CARTESIAN_POINT('Ctrl Pts',(26.0105939396619,45.7643410734543,60.8475011219934)) ;
#7645=CARTESIAN_POINT('Ctrl Pts',(25.9468763160639,45.7673274764264,61.0308984687925)) ;
#7646=CARTESIAN_POINT('Ctrl Pts',(25.7884565009027,45.8675609242035,60.9803505370629)) ;
#7647=CARTESIAN_POINT('Ctrl Pts',(26.3294012120924,46.3280183067159,60.9648183695104)) ;
#7648=CARTESIAN_POINT('Ctrl Pts',(26.2577565707799,46.3310049155992,61.1452672008741)) ;
#7649=CARTESIAN_POINT('Ctrl Pts',(26.1016975009351,46.4312549192417,61.0878703804171)) ;
#7650=CARTESIAN_POINT('Ctrl Pts',(26.4867761257954,46.6093355962199,61.0286488460598)) ;
#7651=CARTESIAN_POINT('Ctrl Pts',(26.411218900482,46.6123217179453,61.2074961609377)) ;
#7652=CARTESIAN_POINT('Ctrl Pts',(26.2564710038353,46.7126174787322,61.1467238390184)) ;
#7653=CARTESIAN_POINT('Ctrl Pts',(26.7966466733539,47.1717937444952,61.1662561586161)) ;
#7654=CARTESIAN_POINT('Ctrl Pts',(26.7133853291535,47.1747789756452,61.3416468164381)) ;
#7655=CARTESIAN_POINT('Ctrl Pts',(26.5613882158301,47.2750030883802,61.2741894600574)) ;
#7656=CARTESIAN_POINT('Ctrl Pts',(26.9490977408211,47.452783888214,61.2399992875839)) ;
#7657=CARTESIAN_POINT('Ctrl Pts',(26.8620488448114,47.4557718391357,61.4135417477089)) ;
#7658=CARTESIAN_POINT('Ctrl Pts',(26.7115606656982,47.5560106522166,61.3428015600556)) ;
#7659=CARTESIAN_POINT('Ctrl Pts',(27.2490465430224,48.0142871287605,61.3973346389138)) ;
#7660=CARTESIAN_POINT('Ctrl Pts',(27.1545450044284,48.0172768213532,61.5669393649232)) ;
#7661=CARTESIAN_POINT('Ctrl Pts',(27.0073417659582,48.1176560532207,61.4897659440178)) ;
#7662=CARTESIAN_POINT('Ctrl Pts',(27.3964165763424,48.2952668191079,61.4808751506582)) ;
#7663=CARTESIAN_POINT('Ctrl Pts',(27.2982508531111,48.298253523814,61.6483796930605)) ;
#7664=CARTESIAN_POINT('Ctrl Pts',(27.1526809617576,48.3984774868501,61.5679867097387)) ;
#7665=CARTESIAN_POINT('Ctrl Pts',(27.6853561273312,48.8569739450404,61.6573296331633)) ;
#7666=CARTESIAN_POINT('Ctrl Pts',(27.5800124452371,48.8599612929924,61.8204175090139)) ;
#7667=CARTESIAN_POINT('Ctrl Pts',(27.4380946261539,48.9602369846067,61.7337961393913)) ;
#7668=CARTESIAN_POINT('Ctrl Pts',(27.8271307922781,49.1378578224168,61.7503802179487)) ;
#7669=CARTESIAN_POINT('Ctrl Pts',(27.7182647454188,49.1408439739518,61.9111378886765)) ;
#7670=CARTESIAN_POINT('Ctrl Pts',(27.5782584466766,49.2411084826924,61.8214479697392)) ;
#7671=CARTESIAN_POINT('Ctrl Pts',(28.1042995146782,49.7002903801074,61.945525014867)) ;
#7672=CARTESIAN_POINT('Ctrl Pts',(27.988549523697,49.7032760750881,62.1013977581118)) ;
#7673=CARTESIAN_POINT('Ctrl Pts',(27.8525562927794,49.8035038746615,62.0056963119981)) ;
#7674=CARTESIAN_POINT('Ctrl Pts',(28.2397716087933,49.981574104122,62.0476554027074)) ;
#7675=CARTESIAN_POINT('Ctrl Pts',(28.1206577488799,49.9845603797024,62.2009788340381)) ;
#7676=CARTESIAN_POINT('Ctrl Pts',(27.9868394128148,50.0849206295178,62.1023846910028)) ;
#7677=CARTESIAN_POINT('Ctrl Pts',(28.5043816473993,50.5452598054824,62.2610884821112)) ;
#7678=CARTESIAN_POINT('Ctrl Pts',(28.3786978494748,50.5482445256917,62.4090687367887)) ;
#7679=CARTESIAN_POINT('Ctrl Pts',(28.2492480466419,50.6484794514239,62.3046924854854)) ;
#7680=CARTESIAN_POINT('Ctrl Pts',(28.6332388724747,50.8275371605559,62.3721571464137)) ;
#7681=CARTESIAN_POINT('Ctrl Pts',(28.5043578421195,50.8305243024046,62.5173611292313)) ;
#7682=CARTESIAN_POINT('Ctrl Pts',(28.3772112458526,50.9307473367347,62.4101803139267)) ;
#7683=CARTESIAN_POINT('Ctrl Pts',(28.821311272216,51.2516112326398,62.5453424745609)) ;
#7684=CARTESIAN_POINT('Ctrl Pts',(28.6877625818993,51.2545984104365,62.6862205204475)) ;
#7685=CARTESIAN_POINT('Ctrl Pts',(28.5642488700406,51.3548887142751,62.574973858029)) ;
#7686=CARTESIAN_POINT('Ctrl Pts',(28.8831921134199,51.3931523912284,62.6042291234362)) ;
#7687=CARTESIAN_POINT('Ctrl Pts',(28.748107618006,51.3961391935655,62.7436360358572)) ;
#7688=CARTESIAN_POINT('Ctrl Pts',(28.6258271935325,51.4964465475109,62.6310493654478)) ;
#7689=CARTESIAN_POINT('Ctrl Pts',(29.0048607208363,51.6761627264484,62.7238846652)) ;
#7690=CARTESIAN_POINT('Ctrl Pts',(28.8667575141589,51.679148867895,62.8602991907019)) ;
#7691=CARTESIAN_POINT('Ctrl Pts',(28.7469484326335,51.7794030062205,62.7450428577575)) ;
#7692=CARTESIAN_POINT('Ctrl Pts',(29.0646528837623,51.8176028378186,62.7846512653971)) ;
#7693=CARTESIAN_POINT('Ctrl Pts',(28.9250665124087,51.8205891355625,62.9195470595252)) ;
#7694=CARTESIAN_POINT('Ctrl Pts',(28.806519466295,51.9208298261689,62.8029822662677)) ;
#7695=CARTESIAN_POINT('Ctrl Pts',(29.240916523989,52.2417288193202,62.969755415835)) ;
#7696=CARTESIAN_POINT('Ctrl Pts',(29.096957913189,52.2447151365731,63.1000268989965)) ;
#7697=CARTESIAN_POINT('Ctrl Pts',(28.9822749700762,52.3449566194198,62.9796178859191)) ;
#7698=CARTESIAN_POINT('Ctrl Pts',(29.3543526842364,52.5241300049544,63.0969834020191)) ;
#7699=CARTESIAN_POINT('Ctrl Pts',(29.207580250032,52.5271161388288,63.2240797522907)) ;
#7700=CARTESIAN_POINT('Ctrl Pts',(29.0955835545825,52.6274277787482,63.1012218259211)) ;
#7701=CARTESIAN_POINT('Ctrl Pts',(29.5725963126369,53.0891744812499,63.3585368522534)) ;
#7702=CARTESIAN_POINT('Ctrl Pts',(29.4204136017986,53.0921595377921,63.4790977763337)) ;
#7703=CARTESIAN_POINT('Ctrl Pts',(29.3138573916988,53.1923844745183,63.3514288365555)) ;
#7704=CARTESIAN_POINT('Ctrl Pts',(29.6773310089795,53.3716654702982,63.492757098003)) ;
#7705=CARTESIAN_POINT('Ctrl Pts',(29.5225534466469,53.3746531996277,63.6099685775886)) ;
#7706=CARTESIAN_POINT('Ctrl Pts',(29.4188136322877,53.474885769066,63.4800061206353)) ;
#7707=CARTESIAN_POINT('Ctrl Pts',(29.8780214581697,53.9365848433025,63.7680888401132)) ;
#7708=CARTESIAN_POINT('Ctrl Pts',(29.7182702841382,53.9395741566699,63.8784329849204)) ;
#7709=CARTESIAN_POINT('Ctrl Pts',(29.6203503545103,54.0399343658536,63.7441201390589)) ;
#7710=CARTESIAN_POINT('Ctrl Pts',(29.9739226608531,54.2194050938164,63.9091508316086)) ;
#7711=CARTESIAN_POINT('Ctrl Pts',(29.811797075346,54.2223916876827,64.0159678115517)) ;
#7712=CARTESIAN_POINT('Ctrl Pts',(29.7167933284806,54.3226177650003,63.8794844435482)) ;
#7713=CARTESIAN_POINT('Ctrl Pts',(30.1563273052154,54.7853172886129,64.1973543020858)) ;
#7714=CARTESIAN_POINT('Ctrl Pts',(29.98968524754,54.7883043794054,64.2969811629213)) ;
#7715=CARTESIAN_POINT('Ctrl Pts',(29.9007532198412,54.888570414198,64.156492633824)) ;
#7716=CARTESIAN_POINT('Ctrl Pts',(30.2429188259929,55.0683374452683,64.3446637303482)) ;
#7717=CARTESIAN_POINT('Ctrl Pts',(30.0741333911327,55.0713235720091,64.4406149178796)) ;
#7718=CARTESIAN_POINT('Ctrl Pts',(29.9883028278047,55.1715968138862,64.2982152529656)) ;
#7719=CARTESIAN_POINT('Ctrl Pts',(30.4059090570349,55.6338317486017,64.6440003385919)) ;
#7720=CARTESIAN_POINT('Ctrl Pts',(30.2330926356945,55.6368172834075,64.7324821192857)) ;
#7721=CARTESIAN_POINT('Ctrl Pts',(30.1535533825065,55.7370429277092,64.5864445252369)) ;
#7722=CARTESIAN_POINT('Ctrl Pts',(30.4823952983082,55.916215478763,64.7961309034391)) ;
#7723=CARTESIAN_POINT('Ctrl Pts',(30.3076853561814,55.9192018042982,64.8808238492804)) ;
#7724=CARTESIAN_POINT('Ctrl Pts',(30.2313935555733,56.0195762764982,64.7331583223123)) ;
#7725=CARTESIAN_POINT('Ctrl Pts',(30.6254121455451,56.4812254904277,65.1054688516006)) ;
#7726=CARTESIAN_POINT('Ctrl Pts',(30.4471709208848,56.4842101347963,65.1824414452389)) ;
#7727=CARTESIAN_POINT('Ctrl Pts',(30.3773704514723,56.5844490941092,65.0315147900252)) ;
#7728=CARTESIAN_POINT('Ctrl Pts',(30.6917624032461,56.763743935905,65.2622767975204)) ;
#7729=CARTESIAN_POINT('Ctrl Pts',(30.5118840267287,56.7667309512707,65.3353401301383)) ;
#7730=CARTESIAN_POINT('Ctrl Pts',(30.4453928475244,56.8669533046602,65.1829163320907)) ;
#7731=CARTESIAN_POINT('Ctrl Pts',(30.8141613823402,57.3288079962077,65.5801651959044)) ;
#7732=CARTESIAN_POINT('Ctrl Pts',(30.6312620619075,57.3317959921678,65.6453060803128)) ;
#7733=CARTESIAN_POINT('Ctrl Pts',(30.5715081411308,57.4320972449782,65.4901649529916)) ;
#7734=CARTESIAN_POINT('Ctrl Pts',(30.8702287449917,57.6115036703986,65.7413392603775)) ;
#7735=CARTESIAN_POINT('Ctrl Pts',(30.6859486276515,57.614489922045,65.802459364614)) ;
#7736=CARTESIAN_POINT('Ctrl Pts',(30.6295920933399,57.7147356136583,65.6460186938791)) ;
#7737=CARTESIAN_POINT('Ctrl Pts',(30.9716670485772,58.1775332618979,66.0670303867177)) ;
#7738=CARTESIAN_POINT('Ctrl Pts',(30.7848903419995,58.1805194049524,66.1200320694339)) ;
#7739=CARTESIAN_POINT('Ctrl Pts',(30.7354281864928,58.2807563670397,65.9612716407878)) ;
#7740=CARTESIAN_POINT('Ctrl Pts',(31.0170807712485,58.4605262973882,66.2317049895088)) ;
#7741=CARTESIAN_POINT('Ctrl Pts',(30.8291853189397,58.4635110441295,66.2806047680588)) ;
#7742=CARTESIAN_POINT('Ctrl Pts',(30.7832293261232,58.5638587343566,66.1208594483691)) ;
#7743=CARTESIAN_POINT('Ctrl Pts',(31.0569564067032,58.7433256931628,66.3973145222243)) ;
#7744=CARTESIAN_POINT('Ctrl Pts',(30.868086917137,58.7463119239391,66.4420830740152)) ;
#7745=CARTESIAN_POINT('Ctrl Pts',(30.8256211934509,58.846513767945,66.281331471652)) ;
#7746=CARTESIAN_POINT('Origin',(23.47768801576,59.8830586252741,68.2224337400009)) ;
#7747=CARTESIAN_POINT('Origin',(-4.86729604997798,45.3830586252741,47.6904007594832)) ;
#7748=CARTESIAN_POINT('',(17.1688739128827,45.3830610445956,63.6388169494918)) ;
#7749=CARTESIAN_POINT('',(0.569856645481698,45.3830586252741,51.5789200251186)) ;
#7750=CARTESIAN_POINT('',(17.1688762698447,45.3830586252741,63.6388137054137)) ;
#7751=CARTESIAN_POINT('Ctrl Pts',(17.1688730549123,45.3830586252741,63.6388181303861)) ;
#7752=CARTESIAN_POINT('Ctrl Pts',(17.1800590780183,45.3830586252741,63.6469452532392)) ;
#7753=CARTESIAN_POINT('Ctrl Pts',(17.1921565915667,45.3830586252741,63.6536652985854)) ;
#7754=CARTESIAN_POINT('Ctrl Pts',(17.2187686671259,45.3830586252741,63.6645720588386)) ;
#7755=CARTESIAN_POINT('Ctrl Pts',(17.2332205987557,45.3830586252741,63.6684413705484)) ;
#7756=CARTESIAN_POINT('Ctrl Pts',(17.2748860520113,45.3830586252741,63.6744361969284)) ;
#7757=CARTESIAN_POINT('Ctrl Pts',(17.3022690103674,45.3830586252741,63.6724758731919)) ;
#7758=CARTESIAN_POINT('Ctrl Pts',(17.3571375210947,45.3830586252741,63.6583151154743)) ;
#7759=CARTESIAN_POINT('Ctrl Pts',(17.3840869789834,45.3830586252736,63.6453977385134)) ;
#7760=CARTESIAN_POINT('Ctrl Pts',(17.4299533045875,45.3830586252736,63.6129782098527)) ;
#7761=CARTESIAN_POINT('Ctrl Pts',(17.4493637769369,45.3830586252741,63.594256853187)) ;
#7762=CARTESIAN_POINT('Ctrl Pts',(17.4656808998813,45.3830586252741,63.5731570074722)) ;
#7763=CARTESIAN_POINT('',(17.1123854551458,45.3830674541108,63.721395608331)) ;
#7764=CARTESIAN_POINT('Ctrl Pts',(17.1437460237931,45.3830586252741,64.0222933688402)) ;
#7765=CARTESIAN_POINT('Ctrl Pts',(17.158246936494,45.3830586252741,64.000424741156)) ;
#7766=CARTESIAN_POINT('Ctrl Pts',(17.1696066385742,45.3830586252745,63.9764616766277)) ;
#7767=CARTESIAN_POINT('Ctrl Pts',(17.185738799857,45.3830586252745,63.9230452426601)) ;
#7768=CARTESIAN_POINT('Ctrl Pts',(17.1894694076506,45.3830586252741,63.8933258428105)) ;
#7769=CARTESIAN_POINT('Ctrl Pts',(17.1855264735452,45.3830586252741,63.8366740578439)) ;
#7770=CARTESIAN_POINT('Ctrl Pts',(17.1787049287075,45.3830586252741,63.8100195880785)) ;
#7771=CARTESIAN_POINT('Ctrl Pts',(17.1599065242039,45.3830586252741,63.7725456534273)) ;
#7772=CARTESIAN_POINT('Ctrl Pts',(17.1518122170667,45.3830586252741,63.7602351390352)) ;
#7773=CARTESIAN_POINT('Ctrl Pts',(17.1334102581903,45.3830586252741,63.7386874610371)) ;
#7774=CARTESIAN_POINT('Ctrl Pts',(17.123408783065,45.3830586252741,63.7294110116011)) ;
#7775=CARTESIAN_POINT('Ctrl Pts',(17.1123823807625,45.3830586252741,63.7213999560576)) ;
#7776=CARTESIAN_POINT('',(1.4648950896395,45.3830586252741,52.352810316749)) ;
#7777=CARTESIAN_POINT('',(1.4648950896395,45.3830586252741,52.352810316749)) ;
#7778=CARTESIAN_POINT('Origin',(5.57939185568678,45.3830586252741,46.6896913561244)) ;
#7779=CARTESIAN_POINT('Ctrl Pts',(17.4100576973813,45.383050240205,63.814048285042)) ;
#7780=CARTESIAN_POINT('Ctrl Pts',(17.6138710905714,45.9804808943662,63.5335228327087)) ;
#7781=CARTESIAN_POINT('Ctrl Pts',(17.8426988440834,46.5779115664506,63.2729997284105)) ;
#7782=CARTESIAN_POINT('Ctrl Pts',(18.0715249883393,47.1753380370388,63.0124784562693)) ;
#7783=CARTESIAN_POINT('Ctrl Pts',(18.3234128709904,47.772764507627,62.7741819348792)) ;
#7784=CARTESIAN_POINT('Ctrl Pts',(18.5753007536416,48.3701909782152,62.5358854134891)) ;
#7785=CARTESIAN_POINT('Ctrl Pts',(18.8481013560865,48.9676174488035,62.3218467047498)) ;
#7786=CARTESIAN_POINT('Ctrl Pts',(19.1209019585313,49.5650439193917,62.1078079960104)) ;
#7787=CARTESIAN_POINT('Ctrl Pts',(19.4122878422165,50.16247038998,61.9198532027167)) ;
#7788=CARTESIAN_POINT('Ctrl Pts',(19.7036737259018,50.7598968605682,61.731898409423)) ;
#7789=CARTESIAN_POINT('Ctrl Pts',(20.0111588892076,51.3573233311564,61.5716310956004)) ;
#7790=CARTESIAN_POINT('Ctrl Pts',(20.3186440525133,51.9547498017447,61.4113637817778)) ;
#7791=CARTESIAN_POINT('Ctrl Pts',(20.6396051404426,52.5521762723329,61.2801512916392)) ;
#7792=CARTESIAN_POINT('Ctrl Pts',(20.9605662283718,53.1496027429211,61.1489388015006)) ;
#7793=CARTESIAN_POINT('Ctrl Pts',(21.29226491409,53.7470292135094,61.0479005937476)) ;
#7794=CARTESIAN_POINT('Ctrl Pts',(21.6239635998081,54.3444556840976,60.9468623859946)) ;
#7795=CARTESIAN_POINT('Ctrl Pts',(21.9635699470823,54.9418821546858,60.8768604829906)) ;
#7796=CARTESIAN_POINT('Ctrl Pts',(22.3031762943565,55.5393086252741,60.8068585799867)) ;
#7797=CARTESIAN_POINT('Ctrl Pts',(22.6477929015737,56.1367350958623,60.7684902132863)) ;
#7798=CARTESIAN_POINT('Ctrl Pts',(22.9924095087908,56.7341615664506,60.7301218465859)) ;
#7799=CARTESIAN_POINT('Ctrl Pts',(23.3390962285664,57.3315880370388,60.7237143615655)) ;
#7800=CARTESIAN_POINT('Ctrl Pts',(23.6441167020902,57.8572133193466,60.71807695464)) ;
#7801=CARTESIAN_POINT('Ctrl Pts',(23.948587351244,58.3830758086166,60.7372314170278)) ;
#7802=CARTESIAN_POINT('Ctrl Pts',(-4.83792013667371,45.383050240205,47.6499682835265)) ;
#7803=CARTESIAN_POINT('Ctrl Pts',(-3.8867909684531,45.9804808943662,46.3408495059708)) ;
#7804=CARTESIAN_POINT('Ctrl Pts',(-2.81892811873079,46.5779115664506,45.1250750192457)) ;
#7805=CARTESIAN_POINT('Ctrl Pts',(-1.75107277886993,47.1753380370388,43.9093090825868)) ;
#7806=CARTESIAN_POINT('Ctrl Pts',(-0.575595993164432,47.772764507627,42.7972586494332)) ;
#7807=CARTESIAN_POINT('Ctrl Pts',(0.599880792541069,48.3701909782152,41.6852082162796)) ;
#7808=CARTESIAN_POINT('Ctrl Pts',(1.872950270617,48.9676174488035,40.6863609088291)) ;
#7809=CARTESIAN_POINT('Ctrl Pts',(3.14601974869293,49.5650439193917,39.6875136013786)) ;
#7810=CARTESIAN_POINT('Ctrl Pts',(4.50582053922401,50.16247038998,38.8103912326747)) ;
#7811=CARTESIAN_POINT('Ctrl Pts',(5.86562132975509,50.7598968605682,37.9332688639709)) ;
#7812=CARTESIAN_POINT('Ctrl Pts',(7.30055209184877,51.3573233311564,37.1853547327988)) ;
#7813=CARTESIAN_POINT('Ctrl Pts',(8.73548285394244,51.9547498017447,36.4374406016267)) ;
#7814=CARTESIAN_POINT('Ctrl Pts',(10.2333012642789,52.5521762723329,35.8251156476465)) ;
#7815=CARTESIAN_POINT('Ctrl Pts',(11.7311196746153,53.1496027429212,35.2127906936662)) ;
#7816=CARTESIAN_POINT('Ctrl Pts',(13.2790468746333,53.7470292135094,34.7412790574855)) ;
#7817=CARTESIAN_POINT('Ctrl Pts',(14.8269740746514,54.3444556840976,34.2697674213048)) ;
#7818=CARTESIAN_POINT('Ctrl Pts',(16.4118036952644,54.9418821546858,33.9430918739531)) ;
#7819=CARTESIAN_POINT('Ctrl Pts',(17.9966333158773,55.5393086252741,33.6164163266014)) ;
#7820=CARTESIAN_POINT('Ctrl Pts',(19.6048441495572,56.1367350958623,33.4373639486663)) ;
#7821=CARTESIAN_POINT('Ctrl Pts',(21.2130549832371,56.7341615664506,33.2583115707312)) ;
#7822=CARTESIAN_POINT('Ctrl Pts',(22.8309263421902,57.3315880370388,33.228409973969)) ;
#7823=CARTESIAN_POINT('Ctrl Pts',(24.2543552186343,57.8572133193466,33.2021020749834)) ;
#7824=CARTESIAN_POINT('Ctrl Pts',(25.6752182480186,58.3830758086166,33.2914895661267)) ;
#7825=CARTESIAN_POINT('',(25.0785449650548,58.3353824278239,41.1845908766823)) ;
#7826=CARTESIAN_POINT('',(23.8674681578449,58.2172712656977,60.4340619665212)) ;
#7827=CARTESIAN_POINT('Ctrl Pts',(25.0785449650548,58.3353824278239,41.1845908766823)) ;
#7828=CARTESIAN_POINT('Ctrl Pts',(24.9165967247392,58.3308357083915,43.7586844600685)) ;
#7829=CARTESIAN_POINT('Ctrl Pts',(24.7350928605288,58.3244410146232,46.6436057862439)) ;
#7830=CARTESIAN_POINT('Ctrl Pts',(24.423261223575,58.3066351812269,51.6000277530103)) ;
#7831=CARTESIAN_POINT('Ctrl Pts',(24.0807588371245,58.2895264404745,57.0439473259468)) ;
#7832=CARTESIAN_POINT('Ctrl Pts',(23.8674708952131,58.2172696107887,60.4340621034685)) ;
#7833=CARTESIAN_POINT('Ctrl Pts',(23.8674681578449,58.2172712656977,60.4340619665212)) ;
#7834=CARTESIAN_POINT('Ctrl Pts',(23.7062059304299,57.9495340002374,60.4259926846083)) ;
#7835=CARTESIAN_POINT('Ctrl Pts',(23.544757653971,57.6819084045905,60.4229408514303)) ;
#7836=CARTESIAN_POINT('Ctrl Pts',(23.3835363156539,57.4145313636579,60.4248870693006)) ;
#7837=CARTESIAN_POINT('Ctrl Pts',(23.233875375543,57.166326630167,60.4266937333512)) ;
#7838=CARTESIAN_POINT('Ctrl Pts',(23.0843664411127,56.9182638872676,60.4328052874967)) ;
#7839=CARTESIAN_POINT('Ctrl Pts',(22.9352053386692,56.6702295478715,60.4432068221641)) ;
#7840=CARTESIAN_POINT('Ctrl Pts',(22.9236835498855,56.6510704023381,60.444010277512)) ;
#7841=CARTESIAN_POINT('Ctrl Pts',(22.9121630148862,56.6319118940957,60.4448393772268)) ;
#7842=CARTESIAN_POINT('Ctrl Pts',(22.9006438534892,56.6127538456681,60.4456941141314)) ;
#7843=CARTESIAN_POINT('Ctrl Pts',(22.7495669628603,56.3614909032359,60.4569042178363)) ;
#7844=CARTESIAN_POINT('Ctrl Pts',(22.5987433261589,56.1103350670462,60.4725243164303)) ;
#7845=CARTESIAN_POINT('Ctrl Pts',(22.4485236466779,55.8590202585561,60.4925253591705)) ;
#7846=CARTESIAN_POINT('Ctrl Pts',(22.439008584219,55.8431017310511,60.4937922449179)) ;
#7847=CARTESIAN_POINT('Ctrl Pts',(22.4294962141314,55.8271830724926,60.4950766333802)) ;
#7848=CARTESIAN_POINT('Ctrl Pts',(22.419986547504,55.8112643008984,60.4963785252368)) ;
#7849=CARTESIAN_POINT('Ctrl Pts',(22.267917029518,55.5567064895583,60.5171971380081)) ;
#7850=CARTESIAN_POINT('Ctrl Pts',(22.1164649280643,55.3019957844117,60.5425026636)) ;
#7851=CARTESIAN_POINT('Ctrl Pts',(21.9656675704896,55.0471908391173,60.5723059396156)) ;
#7852=CARTESIAN_POINT('Ctrl Pts',(21.9581562962121,55.034498906963,60.5737904522365)) ;
#7853=CARTESIAN_POINT('Ctrl Pts',(21.9506466823413,55.0218058655745,60.5752861659703)) ;
#7854=CARTESIAN_POINT('Ctrl Pts',(21.9431388263387,55.0091118266697,60.5767930566487)) ;
#7855=CARTESIAN_POINT('Ctrl Pts',(21.7904748859319,54.7509925981975,60.6074340104226)) ;
#7856=CARTESIAN_POINT('Ctrl Pts',(21.6386230866642,54.4926055130901,60.6426783253807)) ;
#7857=CARTESIAN_POINT('Ctrl Pts',(21.4882181064184,54.2345762733044,60.6823628358805)) ;
#7858=CARTESIAN_POINT('Ctrl Pts',(21.482727917163,54.2251575070006,60.6838114280269)) ;
#7859=CARTESIAN_POINT('Ctrl Pts',(21.4772392198183,54.2157389752756,60.6852660449337)) ;
#7860=CARTESIAN_POINT('Ctrl Pts',(21.4717520252972,54.2063206495464,60.6867266832642)) ;
#7861=CARTESIAN_POINT('Ctrl Pts',(21.3195365964412,53.9450551732692,60.7272449643323)) ;
#7862=CARTESIAN_POINT('Ctrl Pts',(21.1685419560353,53.6840579939663,60.7723810594839)) ;
#7863=CARTESIAN_POINT('Ctrl Pts',(21.019187288141,53.4230444575823,60.8219988105976)) ;
#7864=CARTESIAN_POINT('Ctrl Pts',(21.0156601431058,53.4168803877747,60.8231705784906)) ;
#7865=CARTESIAN_POINT('Ctrl Pts',(21.0121339251964,53.4107163826998,60.8243448352793)) ;
#7866=CARTESIAN_POINT('Ctrl Pts',(21.0086086348855,53.4045524432161,60.8255215807517)) ;
#7867=CARTESIAN_POINT('Ctrl Pts',(20.8574656807716,53.1402803009587,60.8759732517481)) ;
#7868=CARTESIAN_POINT('Ctrl Pts',(20.7079846408797,52.8760533725429,60.9310137169923)) ;
#7869=CARTESIAN_POINT('Ctrl Pts',(20.560170696436,52.6118787196957,60.9906452371905)) ;
#7870=CARTESIAN_POINT('Ctrl Pts',(20.4091128753672,52.3419065760602,61.0515854112862)) ;
#7871=CARTESIAN_POINT('Ctrl Pts',(20.2598865368533,52.0715787920577,61.1172958715969)) ;
#7872=CARTESIAN_POINT('Ctrl Pts',(20.112834022644,51.8011908422988,61.1876330862895)) ;
#7873=CARTESIAN_POINT('Ctrl Pts',(20.1126494080365,51.8008513882915,61.1877213899636)) ;
#7874=CARTESIAN_POINT('Ctrl Pts',(20.1124647968594,51.8005119341975,61.1878097009275)) ;
#7875=CARTESIAN_POINT('Ctrl Pts',(20.1122801891135,51.8001724800175,61.187898019181)) ;
#7876=CARTESIAN_POINT('Ctrl Pts',(19.9669966220693,51.5330270582816,61.2574031791369)) ;
#7877=CARTESIAN_POINT('Ctrl Pts',(19.8235382680195,51.265585354454,61.3315844205049)) ;
#7878=CARTESIAN_POINT('Ctrl Pts',(19.6828053819963,50.998401550286,61.4099799616795)) ;
#7879=CARTESIAN_POINT('Ctrl Pts',(19.6809136341175,50.9948100344075,61.4110337636935)) ;
#7880=CARTESIAN_POINT('Ctrl Pts',(19.6790223692999,50.9912185474961,61.4120883321757)) ;
#7881=CARTESIAN_POINT('Ctrl Pts',(19.6771315896791,50.9876270907846,61.4131436660542)) ;
#7882=CARTESIAN_POINT('Ctrl Pts',(19.5381827811403,50.7236996475845,61.4906975932342)) ;
#7883=CARTESIAN_POINT('Ctrl Pts',(19.401773289945,50.4599498020535,61.5724055573758)) ;
#7884=CARTESIAN_POINT('Ctrl Pts',(19.2679001702012,50.1963788513665,61.6582612121504)) ;
#7885=CARTESIAN_POINT('Ctrl Pts',(19.2644389106561,50.1895642834336,61.6604809908868)) ;
#7886=CARTESIAN_POINT('Ctrl Pts',(19.2609794327328,50.1827500045961,61.6627034870573)) ;
#7887=CARTESIAN_POINT('Ctrl Pts',(19.2575217330171,50.1759360087368,61.6649287021295)) ;
#7888=CARTESIAN_POINT('Ctrl Pts',(19.1254241611857,49.9156148757619,61.7499405689775)) ;
#7889=CARTESIAN_POINT('Ctrl Pts',(18.9960431928179,49.6552611188173,61.8388487050089)) ;
#7890=CARTESIAN_POINT('Ctrl Pts',(18.8694140211807,49.3948957256021,61.9316092105309)) ;
#7891=CARTESIAN_POINT('Ctrl Pts',(18.8645077978792,49.3848079176935,61.9352031987705)) ;
#7892=CARTESIAN_POINT('Ctrl Pts',(18.8596058151151,49.3747203101763,61.9388028976143)) ;
#7893=CARTESIAN_POINT('Ctrl Pts',(18.8547080857952,49.3646329259558,61.9424082972234)) ;
#7894=CARTESIAN_POINT('Ctrl Pts',(18.7298870483059,49.1075509841603,62.0342936772381)) ;
#7895=CARTESIAN_POINT('Ctrl Pts',(18.6076690784898,48.8504690628021,62.1300084731121)) ;
#7896=CARTESIAN_POINT('Ctrl Pts',(18.4884327105145,48.5931578990172,62.229271765735)) ;
#7897=CARTESIAN_POINT('Ctrl Pts',(18.4822469141894,48.5798089981879,62.234421390142)) ;
#7898=CARTESIAN_POINT('Ctrl Pts',(18.4760689516882,48.5664590689812,62.2395807235543)) ;
#7899=CARTESIAN_POINT('Ctrl Pts',(18.4698988891753,48.5531081058639,62.2447497176984)) ;
#7900=CARTESIAN_POINT('Ctrl Pts',(18.3524691682294,48.2990102146422,62.3431269284067)) ;
#7901=CARTESIAN_POINT('Ctrl Pts',(18.2378210041666,48.0446012919297,62.4450654543122)) ;
#7902=CARTESIAN_POINT('Ctrl Pts',(18.1262517854023,47.7903648312084,62.550326771146)) ;
#7903=CARTESIAN_POINT('Ctrl Pts',(18.1189739283107,47.7737805380753,62.5571931526595)) ;
#7904=CARTESIAN_POINT('Ctrl Pts',(18.11170890229,47.7571963611373,62.5640739293288)) ;
#7905=CARTESIAN_POINT('Ctrl Pts',(18.104456753659,47.7406123516807,62.5709690693567)) ;
#7906=CARTESIAN_POINT('Ctrl Pts',(17.9946923640913,47.4896062337403,62.6753299801235)) ;
#7907=CARTESIAN_POINT('Ctrl Pts',(17.8881599074056,47.2387261489802,62.7826999639579)) ;
#7908=CARTESIAN_POINT('Ctrl Pts',(17.7848097317844,46.9878897404752,62.893100191579)) ;
#7909=CARTESIAN_POINT('Ctrl Pts',(17.7766757639826,46.9681481652137,62.9017890195504)) ;
#7910=CARTESIAN_POINT('Ctrl Pts',(17.7685617599153,46.9484074501541,62.9104963668765)) ;
#7911=CARTESIAN_POINT('Ctrl Pts',(17.7604677083785,46.9286675886393,62.9192222283657)) ;
#7912=CARTESIAN_POINT('Ctrl Pts',(17.6589239088363,46.6810214584483,63.0286923899853)) ;
#7913=CARTESIAN_POINT('Ctrl Pts',(17.5604595377658,46.4334531760664,63.1411577287807)) ;
#7914=CARTESIAN_POINT('Ctrl Pts',(17.4653464547407,46.1857600468477,63.256308049298)) ;
#7915=CARTESIAN_POINT('Ctrl Pts',(17.4566036038392,46.162991947768,63.2668927349324)) ;
#7916=CARTESIAN_POINT('Ctrl Pts',(17.4478888840466,46.1402223084084,63.277500332783)) ;
#7917=CARTESIAN_POINT('Ctrl Pts',(17.4392025259141,46.1174510138862,63.288130583901)) ;
#7918=CARTESIAN_POINT('Ctrl Pts',(17.3458579122278,45.8727480373453,63.4023644974539)) ;
#7919=CARTESIAN_POINT('Ctrl Pts',(17.2557287797025,45.627974343213,63.5192728483348)) ;
#7920=CARTESIAN_POINT('Ctrl Pts',(17.1688739128827,45.3830610445956,63.6388169494918)) ;
#7921=CARTESIAN_POINT('',(1.06650400490287,48.5844537758935,41.3386313446643)) ;
#7922=CARTESIAN_POINT('Ctrl Pts',(0.569856645481657,45.3830586252741,51.5789200251186)) ;
#7923=CARTESIAN_POINT('Ctrl Pts',(0.205152783399156,45.4231929016304,51.2052420971489)) ;
#7924=CARTESIAN_POINT('Ctrl Pts',(-0.115007591050823,45.4870033446877,50.7935164752995)) ;
#7925=CARTESIAN_POINT('Ctrl Pts',(-0.66183104916004,45.6539797372435,49.9030397345301)) ;
#7926=CARTESIAN_POINT('Ctrl Pts',(-0.884618914799949,45.7573388893142,49.4261784970127)) ;
#7927=CARTESIAN_POINT('Ctrl Pts',(-1.34560813242504,46.0833507061678,48.0631169416231)) ;
#7928=CARTESIAN_POINT('Ctrl Pts',(-1.46302722997465,46.3336877227691,47.1527476308917)) ;
#7929=CARTESIAN_POINT('Ctrl Pts',(-1.34627520533182,46.9107591797132,45.2786955776573)) ;
#7930=CARTESIAN_POINT('Ctrl Pts',(-1.08232247700463,47.2383195349501,44.3334069001318)) ;
#7931=CARTESIAN_POINT('Ctrl Pts',(-0.215987177965692,47.9083523080807,42.6567201668803)) ;
#7932=CARTESIAN_POINT('Ctrl Pts',(0.364376757671241,48.2450338483641,41.9307797259103)) ;
#7933=CARTESIAN_POINT('Ctrl Pts',(1.06650400490289,48.5844537758935,41.3386313446643)) ;
#7934=CARTESIAN_POINT('',(1.10488630355745,48.6029307720944,41.3065881552646)) ;
#7935=CARTESIAN_POINT('Origin',(-21.0084886185846,48.3727968889151,14.7032769090681)) ;
#7936=CARTESIAN_POINT('',(16.7460459354099,55.0677871747466,33.875818260496)) ;
#7937=CARTESIAN_POINT('Ctrl Pts',(1.10488630355745,48.6029307720944,41.3065881552646)) ;
#7938=CARTESIAN_POINT('Ctrl Pts',(1.48456672001327,48.785356686239,40.9910857258634)) ;
#7939=CARTESIAN_POINT('Ctrl Pts',(1.872950270617,48.9676174488035,40.6863609088291)) ;
#7940=CARTESIAN_POINT('Ctrl Pts',(3.14601974869293,49.5650439193917,39.6875136013786)) ;
#7941=CARTESIAN_POINT('Ctrl Pts',(4.50582053922401,50.16247038998,38.8103912326747)) ;
#7942=CARTESIAN_POINT('Ctrl Pts',(5.86562132975509,50.7598968605682,37.9332688639709)) ;
#7943=CARTESIAN_POINT('Ctrl Pts',(7.30055209184877,51.3573233311564,37.1853547327988)) ;
#7944=CARTESIAN_POINT('Ctrl Pts',(8.73548285394244,51.9547498017447,36.4374406016267)) ;
#7945=CARTESIAN_POINT('Ctrl Pts',(10.2333012642789,52.5521762723329,35.8251156476465)) ;
#7946=CARTESIAN_POINT('Ctrl Pts',(11.7311196746153,53.1496027429211,35.2127906936662)) ;
#7947=CARTESIAN_POINT('Ctrl Pts',(13.2790468746333,53.7470292135094,34.7412790574855)) ;
#7948=CARTESIAN_POINT('Ctrl Pts',(14.8269740746514,54.3444556840976,34.2697674213048)) ;
#7949=CARTESIAN_POINT('Ctrl Pts',(16.4118036952644,54.9418821546858,33.9430918739531)) ;
#7950=CARTESIAN_POINT('Ctrl Pts',(16.5787680203067,55.0048219850164,33.9086760846708)) ;
#7951=CARTESIAN_POINT('Ctrl Pts',(16.7460459354099,55.0677871747466,33.875818260496)) ;
#7952=CARTESIAN_POINT('',(16.7951325976017,55.0862551252693,33.8663068761758)) ;
#7953=CARTESIAN_POINT('Origin',(9.80672900050722,55.553531622349,-1.52672131664897)) ;
#7954=CARTESIAN_POINT('Ctrl Pts',(16.7951325976017,55.0862551252692,33.8663068761758)) ;
#7955=CARTESIAN_POINT('Ctrl Pts',(17.3269366349108,55.2861476150253,33.7660169109597)) ;
#7956=CARTESIAN_POINT('Ctrl Pts',(17.8689949355364,55.4856143511659,33.7276579994428)) ;
#7957=CARTESIAN_POINT('Ctrl Pts',(18.9906738261853,55.8948726679075,33.7786821697219)) ;
#7958=CARTESIAN_POINT('Ctrl Pts',(19.5668322091791,56.1030296514258,33.8772515792835)) ;
#7959=CARTESIAN_POINT('Ctrl Pts',(21.042556999384,56.639522788727,34.3251774027028)) ;
#7960=CARTESIAN_POINT('Ctrl Pts',(21.8999253408597,56.9553075668519,34.791153792355)) ;
#7961=CARTESIAN_POINT('Ctrl Pts',(23.3209771338725,57.5027527547765,36.0053548133869)) ;
#7962=CARTESIAN_POINT('Ctrl Pts',(23.8915820353075,57.7356391827932,36.71956623351)) ;
#7963=CARTESIAN_POINT('Ctrl Pts',(24.6195664683639,58.058368696673,38.1284250825275)) ;
#7964=CARTESIAN_POINT('Ctrl Pts',(24.8427619123796,58.167950706673,38.7711976908919)) ;
#7965=CARTESIAN_POINT('Ctrl Pts',(25.0783873637464,58.3023924852745,40.0133620327521)) ;
#7966=CARTESIAN_POINT('Ctrl Pts',(25.1153550438448,58.3364158759195,40.5995114251688)) ;
#7967=CARTESIAN_POINT('Ctrl Pts',(25.0785449650548,58.3353824278239,41.1845908766823)) ;
#7968=CARTESIAN_POINT('Ctrl Pts',(-4.89668542317829,45.3830585852922,47.7308516627133)) ;
#7969=CARTESIAN_POINT('Ctrl Pts',(-3.94930237640841,45.9804850758286,46.4190251645259)) ;
#7970=CARTESIAN_POINT('Ctrl Pts',(-2.88492061603778,46.5779115664506,45.2002081697134)) ;
#7971=CARTESIAN_POINT('Ctrl Pts',(-1.82053889135939,47.1753380370388,43.9813912157718)) ;
#7972=CARTESIAN_POINT('Ctrl Pts',(-0.64823939064702,47.772764507627,42.8659822756631)) ;
#7973=CARTESIAN_POINT('Ctrl Pts',(0.524060110065356,48.3701909782152,41.7505733355544)) ;
#7974=CARTESIAN_POINT('Ctrl Pts',(1.7942757408128,48.9676174488035,40.7480886850736)) ;
#7975=CARTESIAN_POINT('Ctrl Pts',(3.06449137156023,49.5650439193917,39.7456040345928)) ;
#7976=CARTESIAN_POINT('Ctrl Pts',(4.42178610044663,50.16247038998,38.8645965193115)) ;
#7977=CARTESIAN_POINT('Ctrl Pts',(5.77908082933302,50.7598968605682,37.9835890040303)) ;
#7978=CARTESIAN_POINT('Ctrl Pts',(7.21187469630014,51.3573233311564,37.2315750694345)) ;
#7979=CARTESIAN_POINT('Ctrl Pts',(8.64466856326726,51.9547498017447,36.4795611348387)) ;
#7980=CARTESIAN_POINT('Ctrl Pts',(10.140737476231,52.5521762723329,35.8629566986657)) ;
#7981=CARTESIAN_POINT('Ctrl Pts',(11.6368063891948,53.1496027429212,35.2463522624928)) ;
#7982=CARTESIAN_POINT('Ctrl Pts',(13.1833864156889,53.7470292135094,34.7704179763834)) ;
#7983=CARTESIAN_POINT('Ctrl Pts',(14.729966442183,54.3444556840976,34.2944836902741)) ;
#7984=CARTESIAN_POINT('Ctrl Pts',(16.31386270673,54.9418821546858,33.9632800577477)) ;
#7985=CARTESIAN_POINT('Ctrl Pts',(17.8977589712771,55.5393086252741,33.6320764252214)) ;
#7986=CARTESIAN_POINT('Ctrl Pts',(19.5054582294142,56.1367350958623,33.4484291588917)) ;
#7987=CARTESIAN_POINT('Ctrl Pts',(21.1131574875512,56.7341615664506,33.2647818925619)) ;
#7988=CARTESIAN_POINT('Ctrl Pts',(22.7309434160666,57.3315880370388,33.230257806153)) ;
#7989=CARTESIAN_POINT('Ctrl Pts',(24.1543552347212,57.8572347768351,33.199881727491)) ;
#7990=CARTESIAN_POINT('Ctrl Pts',(25.5755313903897,58.3831186720347,33.2852178054411)) ;
#7991=CARTESIAN_POINT('Ctrl Pts',(17.351282019329,45.3830585852922,63.8949460662004)) ;
#7992=CARTESIAN_POINT('Ctrl Pts',(17.5513538557446,45.9804850758286,63.6117052136026)) ;
#7993=CARTESIAN_POINT('Ctrl Pts',(17.7767063905955,46.5779115664506,63.3481329173662)) ;
#7994=CARTESIAN_POINT('Ctrl Pts',(18.0020589178895,47.1753380370388,63.0845606299682)) ;
#7995=CARTESIAN_POINT('Ctrl Pts',(18.2507695135888,47.772764507627,62.8429056034762)) ;
#7996=CARTESIAN_POINT('Ctrl Pts',(18.4994801092881,48.3701909782152,62.6012505769841)) ;
#7997=CARTESIAN_POINT('Ctrl Pts',(18.7694268622831,48.9676174488035,62.3835745268788)) ;
#7998=CARTESIAN_POINT('Ctrl Pts',(19.0393736152781,49.5650439193917,62.1658984767735)) ;
#7999=CARTESIAN_POINT('Ctrl Pts',(19.3282534350527,50.16247038998,61.974058538364)) ;
#8000=CARTESIAN_POINT('Ctrl Pts',(19.6171332548274,50.7598968605682,61.7822185999545)) ;
#8001=CARTESIAN_POINT('Ctrl Pts',(19.9224815206155,51.3573233311564,61.6178514839545)) ;
#8002=CARTESIAN_POINT('Ctrl Pts',(20.2278297864037,51.9547498017447,61.4534843679545)) ;
#8003=CARTESIAN_POINT('Ctrl Pts',(20.5470413744644,52.5521762723329,61.3179923966435)) ;
#8004=CARTESIAN_POINT('Ctrl Pts',(20.8662529625251,53.1496027429211,61.1825004253324)) ;
#8005=CARTESIAN_POINT('Ctrl Pts',(21.1966044721399,53.7470292135094,61.0770395684365)) ;
#8006=CARTESIAN_POINT('Ctrl Pts',(21.5269559817547,54.3444556840976,60.9715787115406)) ;
#8007=CARTESIAN_POINT('Ctrl Pts',(21.8656289703221,54.9418821546858,60.8970487239063)) ;
#8008=CARTESIAN_POINT('Ctrl Pts',(22.2043019588896,55.5393086252741,60.8225187362721)) ;
#8009=CARTESIAN_POINT('Ctrl Pts',(22.5484069878841,56.1367350958623,60.7795554814755)) ;
#8010=CARTESIAN_POINT('Ctrl Pts',(22.8925120168785,56.7341615664506,60.7365922266788)) ;
#8011=CARTESIAN_POINT('Ctrl Pts',(23.2391133035206,57.3315880370388,60.7255622520614)) ;
#8012=CARTESIAN_POINT('Ctrl Pts',(23.5440710603357,57.8572347768351,60.7158575093304)) ;
#8013=CARTESIAN_POINT('Ctrl Pts',(23.8488094920358,58.3831186720347,60.7309539896547)) ;
#8014=CARTESIAN_POINT('',(23.8673496931823,58.3830537363176,60.4362583055437)) ;
#8015=CARTESIAN_POINT('Ctrl Pts',(17.1123854551458,45.3830674541108,63.721395608331)) ;
#8016=CARTESIAN_POINT('Ctrl Pts',(17.1182555903267,45.3999249614348,63.7130941959663)) ;
#8017=CARTESIAN_POINT('Ctrl Pts',(17.1242245528045,45.4170195560983,63.7046879792065)) ;
#8018=CARTESIAN_POINT('Ctrl Pts',(17.136110401805,45.4509660823352,63.6880190307945)) ;
#8019=CARTESIAN_POINT('Ctrl Pts',(17.1420688908599,45.4679374856688,63.6796974657324)) ;
#8020=CARTESIAN_POINT('Ctrl Pts',(17.1599909175645,45.5188462146264,63.6547715850251)) ;
#8021=CARTESIAN_POINT('Ctrl Pts',(17.1720010144541,45.5527780591985,63.6382060836503)) ;
#8022=CARTESIAN_POINT('Ctrl Pts',(17.2082164796663,45.6545524513439,63.5886655433169)) ;
#8023=CARTESIAN_POINT('Ctrl Pts',(17.2326070347849,45.7223738576063,63.5558464774858)) ;
#8024=CARTESIAN_POINT('Ctrl Pts',(17.2882647437757,45.8755455989769,63.4821716097248)) ;
#8025=CARTESIAN_POINT('Ctrl Pts',(17.3196760141081,45.9608834226833,63.4414374945538)) ;
#8026=CARTESIAN_POINT('Ctrl Pts',(17.370165521914,46.0963466756243,63.3772837588605)) ;
#8027=CARTESIAN_POINT('Ctrl Pts',(17.3889996936742,46.1464973799216,63.3536369427366)) ;
#8028=CARTESIAN_POINT('Ctrl Pts',(17.4955782697342,46.4282028809689,63.2214096186718)) ;
#8029=CARTESIAN_POINT('Ctrl Pts',(17.5860373897972,46.6594344485538,63.1151569797222)) ;
#8030=CARTESIAN_POINT('Ctrl Pts',(17.6949271722414,46.9296827699032,62.9939899321235)) ;
#8031=CARTESIAN_POINT('Ctrl Pts',(17.7107643919321,46.9687950424163,62.976526950364)) ;
#8032=CARTESIAN_POINT('Ctrl Pts',(17.8251792031112,47.2499758749393,62.8515103176276)) ;
#8033=CARTESIAN_POINT('Ctrl Pts',(17.9265852618937,47.4918541916698,62.746770719906)) ;
#8034=CARTESIAN_POINT('Ctrl Pts',(18.1520599948226,48.0143150857794,62.526576356011)) ;
#8035=CARTESIAN_POINT('Ctrl Pts',(18.2770523113096,48.2952954282315,62.4122348405312)) ;
#8036=CARTESIAN_POINT('Ctrl Pts',(18.4133728607043,48.593120430708,62.2954439777444)) ;
#8037=CARTESIAN_POINT('Ctrl Pts',(18.4211678305597,48.6101204742723,62.2887923752948)) ;
#8038=CARTESIAN_POINT('Ctrl Pts',(18.5501994677138,48.8910362150329,62.1791264958796)) ;
#8039=CARTESIAN_POINT('Ctrl Pts',(18.6746809217014,49.154922679681,62.0797249566039)) ;
#8040=CARTESIAN_POINT('Ctrl Pts',(18.8049007382563,49.4249376060055,61.9821239583166)) ;
#8041=CARTESIAN_POINT('Ctrl Pts',(18.8077299832015,49.4308011237539,61.980006410541)) ;
#8042=CARTESIAN_POINT('Ctrl Pts',(18.9409149634897,49.7066812295575,61.8804651685687)) ;
#8043=CARTESIAN_POINT('Ctrl Pts',(19.0744281513532,49.9768666464288,61.7870358280021)) ;
#8044=CARTESIAN_POINT('Ctrl Pts',(19.2136570314282,50.2527043291671,61.6959902898179)) ;
#8045=CARTESIAN_POINT('Ctrl Pts',(19.2163616978931,50.2580605419638,61.6942240338067)) ;
#8046=CARTESIAN_POINT('Ctrl Pts',(19.3530104917543,50.5285623062289,61.6051079770347)) ;
#8047=CARTESIAN_POINT('Ctrl Pts',(19.4896723531249,50.7940892820341,61.5218500905069)) ;
#8048=CARTESIAN_POINT('Ctrl Pts',(19.6378635331462,51.0767673302897,61.4377267779672)) ;
#8049=CARTESIAN_POINT('Ctrl Pts',(19.6466506236689,51.0935097128495,61.4327611474076)) ;
#8050=CARTESIAN_POINT('Ctrl Pts',(19.7297354246784,51.2516332986689,61.3860219320458)) ;
#8051=CARTESIAN_POINT('Ctrl Pts',(19.8048581245304,51.3931664825954,61.3453693189635)) ;
#8052=CARTESIAN_POINT('Ctrl Pts',(19.9411643864943,51.6479675595812,61.2744794803297)) ;
#8053=CARTESIAN_POINT('Ctrl Pts',(20.0021436698153,51.7612319406867,61.2437773525758)) ;
#8054=CARTESIAN_POINT('Ctrl Pts',(20.0787570680475,51.9026374456283,61.2064554735793)) ;
#8055=CARTESIAN_POINT('Ctrl Pts',(20.0940444369611,51.9308091085123,61.1990699995767)) ;
#8056=CARTESIAN_POINT('Ctrl Pts',(20.2630277485757,52.2417252333154,61.1181119533642)) ;
#8057=CARTESIAN_POINT('Ctrl Pts',(20.4190788234136,52.524119549279,61.0495454272598)) ;
#8058=CARTESIAN_POINT('Ctrl Pts',(20.7067517642157,53.0381974993202,60.9342400965987)) ;
#8059=CARTESIAN_POINT('Ctrl Pts',(20.8376177185125,53.2697333986823,60.8858199040384)) ;
#8060=CARTESIAN_POINT('Ctrl Pts',(20.9988733465646,53.5522259966914,60.831031906915)) ;
#8061=CARTESIAN_POINT('Ctrl Pts',(21.0280209326871,53.6031771340238,60.8213204978166)) ;
#8062=CARTESIAN_POINT('Ctrl Pts',(21.183426574497,53.8742457620983,60.7705601480465)) ;
#8063=CARTESIAN_POINT('Ctrl Pts',(21.3107285320407,54.0945463050598,60.7325518486177)) ;
#8064=CARTESIAN_POINT('Ctrl Pts',(21.4752926476314,54.3774106831902,60.6879647640456)) ;
#8065=CARTESIAN_POINT('Ctrl Pts',(21.5117056194114,54.4398806254182,60.6783814028631)) ;
#8066=CARTESIAN_POINT('Ctrl Pts',(21.6702778897318,54.7114321393038,60.6378739818295)) ;
#8067=CARTESIAN_POINT('Ctrl Pts',(21.7932788702932,54.9205828276702,60.6096170503781)) ;
#8068=CARTESIAN_POINT('Ctrl Pts',(21.9603429329453,55.203368432955,60.5754722779609)) ;
#8069=CARTESIAN_POINT('Ctrl Pts',(22.0040512805472,55.2772338818095,60.5669287745172)) ;
#8070=CARTESIAN_POINT('Ctrl Pts',(22.1647806110715,55.5485088102251,60.5369417955332)) ;
#8071=CARTESIAN_POINT('Ctrl Pts',(22.2821573285742,55.7457837763586,60.5178093132553)) ;
#8072=CARTESIAN_POINT('Ctrl Pts',(22.450831654825,56.0282588904741,60.4942633908894)) ;
#8073=CARTESIAN_POINT('Ctrl Pts',(22.5018036784155,56.1134884206088,60.4876618904377)) ;
#8074=CARTESIAN_POINT('Ctrl Pts',(22.6640819348038,56.3844426291133,60.4682748073054)) ;
#8075=CARTESIAN_POINT('Ctrl Pts',(22.7754796800465,56.5701302611216,60.4573949544576)) ;
#8076=CARTESIAN_POINT('Ctrl Pts',(22.9452620536937,56.8526653483,60.4444955791702)) ;
#8077=CARTESIAN_POINT('Ctrl Pts',(23.0034860747583,56.9494716030797,60.4407289267428)) ;
#8078=CARTESIAN_POINT('Ctrl Pts',(23.1666024780397,57.2204413601139,60.4320127348201)) ;
#8079=CARTESIAN_POINT('Ctrl Pts',(23.2716417516358,57.3946576755336,60.4285278227131)) ;
#8080=CARTESIAN_POINT('Ctrl Pts',(23.4421351823808,57.6774250653637,60.426319247965)) ;
#8081=CARTESIAN_POINT('Ctrl Pts',(23.5075650498815,57.7859396412674,60.4262949212388)) ;
#8082=CARTESIAN_POINT('Ctrl Pts',(23.5893294576124,57.921622741885,60.4272945872543)) ;
#8083=CARTESIAN_POINT('Ctrl Pts',(23.6056644130462,57.9487278912592,60.4275457298318)) ;
#8084=CARTESIAN_POINT('Ctrl Pts',(23.662889166053,58.0436810159816,60.4286055603454)) ;
#8085=CARTESIAN_POINT('Ctrl Pts',(23.7037872596467,58.1115399743061,60.4296853156621)) ;
#8086=CARTESIAN_POINT('Ctrl Pts',(23.7651325370338,58.2133484522833,60.4317881034382)) ;
#8087=CARTESIAN_POINT('Ctrl Pts',(23.785578913315,58.2472850649071,60.4325694758602)) ;
#8088=CARTESIAN_POINT('Ctrl Pts',(23.8162473293565,58.2981973836593,60.4338623341475)) ;
#8089=CARTESIAN_POINT('Ctrl Pts',(23.8264699432712,58.3151693899118,60.4343134204592)) ;
#8090=CARTESIAN_POINT('Ctrl Pts',(23.8394771596519,58.3367668565656,60.4349130214635)) ;
#8091=CARTESIAN_POINT('Ctrl Pts',(23.8422673657082,58.3413999128699,60.4350431404392)) ;
#8092=CARTESIAN_POINT('Ctrl Pts',(23.8525116996386,58.3584108602029,60.4355263988823)) ;
#8093=CARTESIAN_POINT('Ctrl Pts',(23.8599705749502,58.3707975233386,60.4358890556515)) ;
#8094=CARTESIAN_POINT('Ctrl Pts',(23.8673485046708,58.3830508753326,60.436258249004)) ;
#8095=CARTESIAN_POINT('',(25.0785449650548,58.3831162793798,41.1845908766823)) ;
#8096=CARTESIAN_POINT('Ctrl Pts',(23.8673327885118,58.38309009802,60.4362572466387)) ;
#8097=CARTESIAN_POINT('Ctrl Pts',(24.0692014846605,58.3831052593851,57.2276461840538)) ;
#8098=CARTESIAN_POINT('Ctrl Pts',(24.2710701808123,58.3831073991803,54.0190351214176)) ;
#8099=CARTESIAN_POINT('Ctrl Pts',(24.6748075729936,58.3831134572106,47.6018129980939)) ;
#8100=CARTESIAN_POINT('Ctrl Pts',(24.8766762690243,58.383115023513,44.393201937388)) ;
#8101=CARTESIAN_POINT('Ctrl Pts',(25.0785449650548,58.3831162793798,41.1845908766823)) ;
#8102=CARTESIAN_POINT('',(16.7460321974209,55.1047242171091,33.8757481656485)) ;
#8103=CARTESIAN_POINT('Ctrl Pts',(25.0785449650548,58.3831162793797,41.1845908766823)) ;
#8104=CARTESIAN_POINT('Ctrl Pts',(25.1155757155261,58.3831165097557,40.5960039492146)) ;
#8105=CARTESIAN_POINT('Ctrl Pts',(25.0779368416003,58.3477204189414,40.0063991848858)) ;
#8106=CARTESIAN_POINT('Ctrl Pts',(24.838960064421,58.2097833704152,38.7566097094888)) ;
#8107=CARTESIAN_POINT('Ctrl Pts',(24.6125958308685,58.0979491851445,38.1099399214988)) ;
#8108=CARTESIAN_POINT('Ctrl Pts',(23.8774133952963,57.7707078254696,36.6991149643586)) ;
#8109=CARTESIAN_POINT('Ctrl Pts',(23.303921871022,57.5360202457533,35.9865255376264)) ;
#8110=CARTESIAN_POINT('Ctrl Pts',(21.8778342174311,56.9856758817169,34.7770271162412)) ;
#8111=CARTESIAN_POINT('Ctrl Pts',(21.0183674292568,56.6687344805944,34.3140462118494)) ;
#8112=CARTESIAN_POINT('Ctrl Pts',(19.5365000825384,56.1294192803768,33.8704549815538)) ;
#8113=CARTESIAN_POINT('Ctrl Pts',(18.9557023901162,55.9194276565173,33.77390896011)) ;
#8114=CARTESIAN_POINT('Ctrl Pts',(17.8260154983585,55.506862709361,33.7288845369499)) ;
#8115=CARTESIAN_POINT('Ctrl Pts',(17.2806296106359,55.3059551814418,33.77097165732)) ;
#8116=CARTESIAN_POINT('Ctrl Pts',(16.7460321974209,55.104724217109,33.8757481656485)) ;
#8117=CARTESIAN_POINT('',(1.10484064496481,48.6398835186857,41.3065332251917)) ;
#8118=CARTESIAN_POINT('Ctrl Pts',(1.10484064496481,48.6398835186857,41.3065332251917)) ;
#8119=CARTESIAN_POINT('Ctrl Pts',(1.44601886987501,48.8038201453524,41.0229414372091)) ;
#8120=CARTESIAN_POINT('Ctrl Pts',(1.79427577681365,48.9676174488035,40.7480887309581)) ;
#8121=CARTESIAN_POINT('Ctrl Pts',(3.06449140543972,49.5650439193917,39.7456040821417)) ;
#8122=CARTESIAN_POINT('Ctrl Pts',(4.42178613206022,50.16247038998,38.864596568322)) ;
#8123=CARTESIAN_POINT('Ctrl Pts',(5.77908085868072,50.7598968605682,37.9835890545023)) ;
#8124=CARTESIAN_POINT('Ctrl Pts',(7.21187472325676,51.3573233311564,37.2315751211528)) ;
#8125=CARTESIAN_POINT('Ctrl Pts',(8.6446685878328,51.9547498017447,36.4795611878033)) ;
#8126=CARTESIAN_POINT('Ctrl Pts',(10.1407374983007,52.5521762723329,35.8629567526507)) ;
#8127=CARTESIAN_POINT('Ctrl Pts',(11.6368064087686,53.1496027429211,35.2463523174981)) ;
#8128=CARTESIAN_POINT('Ctrl Pts',(13.1833864326833,53.7470292135094,34.7704180321744)) ;
#8129=CARTESIAN_POINT('Ctrl Pts',(14.729966456598,54.3444556840976,34.2944837468508)) ;
#8130=CARTESIAN_POINT('Ctrl Pts',(16.3138627185042,54.9418821546858,33.9632801148688)) ;
#8131=CARTESIAN_POINT('Ctrl Pts',(16.5296717625019,55.0232827101246,33.9181529554041)) ;
#8132=CARTESIAN_POINT('Ctrl Pts',(16.7460321974209,55.1047242171091,33.8757481656485)) ;
#8133=CARTESIAN_POINT('Ctrl Pts',(1.10484064496482,48.6398835186857,41.3065332251917)) ;
#8134=CARTESIAN_POINT('Ctrl Pts',(0.688510729437327,48.4398363968332,41.6525920780571)) ;
#8135=CARTESIAN_POINT('Ctrl Pts',(0.313395234053494,48.2402511072957,42.0460608191272)) ;
#8136=CARTESIAN_POINT('Ctrl Pts',(-0.361789782441167,47.8311034847342,42.9428152265227)) ;
#8137=CARTESIAN_POINT('Ctrl Pts',(-0.652682875411226,47.62311970224,43.4491246060191)) ;
#8138=CARTESIAN_POINT('Ctrl Pts',(-1.24789105437135,47.0862681322599,44.8711986217157)) ;
#8139=CARTESIAN_POINT('Ctrl Pts',(-1.43533510647897,46.770327077101,45.8290078005203)) ;
#8140=CARTESIAN_POINT('Ctrl Pts',(-1.4052997838034,46.2216257312613,47.6989976412504)) ;
#8141=CARTESIAN_POINT('Ctrl Pts',(-1.21835231594779,45.9879058539332,48.5942607190196)) ;
#8142=CARTESIAN_POINT('Ctrl Pts',(-0.596411936332433,45.6640068779433,50.0526247730249)) ;
#8143=CARTESIAN_POINT('Ctrl Pts',(-0.243839452258383,45.5539383973837,50.6333814528433)) ;
#8144=CARTESIAN_POINT('Ctrl Pts',(0.562423093908943,45.4179657782124,51.605995305929)) ;
#8145=CARTESIAN_POINT('Ctrl Pts',(0.990533295549593,45.3830586252741,52.0081662996818)) ;
#8146=CARTESIAN_POINT('Ctrl Pts',(1.46489508963947,45.3830586252741,52.352810316749)) ;
#8147=CARTESIAN_POINT('Origin',(5.57939185568678,45.3822493559848,46.6896913561244)) ;
#8148=CARTESIAN_POINT('',(1.10484064496481,45.3822493559848,41.3065332251917)) ;
#8149=CARTESIAN_POINT('Origin',(23.4776880157599,45.3822493559848,68.2224337400009)) ;
#8150=CARTESIAN_POINT('',(16.7460321974209,45.3822493559848,33.8757481656485)) ;
#8151=CARTESIAN_POINT('Origin',(18.0923578658931,45.3822493559848,40.74505724258)) ;
#8152=CARTESIAN_POINT('',(25.0785449650548,45.3822493559848,41.1845908766823)) ;
#8153=CARTESIAN_POINT('Origin',(23.8487920953129,45.3822493559848,60.7309531278765)) ;
#8154=CARTESIAN_POINT('Ctrl Pts',(23.8550298361323,57.8271591833517,60.6318070761082)) ;
#8155=CARTESIAN_POINT('Ctrl Pts',(23.8550352275545,57.8726762313018,60.6317213819064)) ;
#8156=CARTESIAN_POINT('Ctrl Pts',(23.855296076976,57.918955920172,60.627575298638)) ;
#8157=CARTESIAN_POINT('Ctrl Pts',(23.8563587264365,58.0070760893886,60.6106849690344)) ;
#8158=CARTESIAN_POINT('Ctrl Pts',(23.8571732808255,58.0511720064474,60.59773799811)) ;
#8159=CARTESIAN_POINT('Ctrl Pts',(23.8594428410483,58.1280396084341,60.5616643711575)) ;
#8160=CARTESIAN_POINT('Ctrl Pts',(23.8607537844068,58.1581206858333,60.5408275229561)) ;
#8161=CARTESIAN_POINT('Ctrl Pts',(23.8630017351916,58.1912258389784,60.5050973681879)) ;
#8162=CARTESIAN_POINT('Ctrl Pts',(23.8638861728135,58.2011509267549,60.4910396347398)) ;
#8163=CARTESIAN_POINT('Ctrl Pts',(23.8656938863924,58.2136664809647,60.4623068500248)) ;
#8164=CARTESIAN_POINT('Ctrl Pts',(23.8665670166679,58.2169696033441,60.4484288416232)) ;
#8165=CARTESIAN_POINT('Ctrl Pts',(23.8674708869362,58.2172758076353,60.4340622350259)) ;
#8166=CARTESIAN_POINT('Ctrl Pts',(23.8673327749686,58.3830247512608,60.4362574619018)) ;
#8167=CARTESIAN_POINT('Ctrl Pts',(23.8668913274621,58.3830247228383,60.4432740691308)) ;
#8168=CARTESIAN_POINT('Ctrl Pts',(23.8664534737013,58.3837424765051,60.4502335554086)) ;
#8169=CARTESIAN_POINT('Ctrl Pts',(23.8655593939275,58.3866521090668,60.4644445465522)) ;
#8170=CARTESIAN_POINT('Ctrl Pts',(23.8651108505696,58.3889169428591,60.4715739391106)) ;
#8171=CARTESIAN_POINT('Ctrl Pts',(23.8636819932964,58.3985444430715,60.4942849752503)) ;
#8172=CARTESIAN_POINT('Ctrl Pts',(23.8627851038498,58.408561172042,60.5085406252432)) ;
#8173=CARTESIAN_POINT('Ctrl Pts',(23.8605808340613,58.4411881110197,60.543576490452)) ;
#8174=CARTESIAN_POINT('Ctrl Pts',(23.859318365517,58.4701790972424,60.5636428530834)) ;
#8175=CARTESIAN_POINT('Ctrl Pts',(23.8571082748939,58.5450324120561,60.5987712378107)) ;
#8176=CARTESIAN_POINT('Ctrl Pts',(23.8563138253378,58.5884045335181,60.6113986531833)) ;
#8177=CARTESIAN_POINT('Ctrl Pts',(23.8552791568201,58.6752752681888,60.6278442384343)) ;
#8178=CARTESIAN_POINT('Ctrl Pts',(23.8550297927293,58.7210386855151,60.6318077659803)) ;
#8179=CARTESIAN_POINT('Ctrl Pts',(23.8550298103818,58.7660385537572,60.6318074854008)) ;
#8180=CARTESIAN_POINT('Ctrl Pts',(23.9138964394444,58.2943663992286,60.4365240299658)) ;
#8181=CARTESIAN_POINT('Ctrl Pts',(23.9017702691677,58.2924602039142,60.6324139695376)) ;
#8182=CARTESIAN_POINT('Ctrl Pts',(24.0693253324374,58.191081348463,60.6454973349943)) ;
#8183=CARTESIAN_POINT('Ctrl Pts',(23.5875061423568,57.7522999682109,60.4182390850653)) ;
#8184=CARTESIAN_POINT('Ctrl Pts',(23.5835904522462,57.7503889244903,60.6146349637289)) ;
#8185=CARTESIAN_POINT('Ctrl Pts',(23.7516792744512,57.6489874076351,60.6206942679821)) ;
#8186=CARTESIAN_POINT('Ctrl Pts',(23.2604720834133,57.2111033102479,60.4205244415559)) ;
#8187=CARTESIAN_POINT('Ctrl Pts',(23.2647892639797,57.2091968025947,60.6169122222677)) ;
#8188=CARTESIAN_POINT('Ctrl Pts',(23.4330242330242,57.1078632090985,60.6159239897169)) ;
#8189=CARTESIAN_POINT('Ctrl Pts',(22.7725719487901,56.3997926693515,60.4545477382972)) ;
#8190=CARTESIAN_POINT('Ctrl Pts',(22.7891733238429,56.3978864499763,60.650151731163)) ;
#8191=CARTESIAN_POINT('Ctrl Pts',(22.9568924415001,56.2965290899915,60.6386340110724)) ;
#8192=CARTESIAN_POINT('Ctrl Pts',(22.61021664358,56.1295297083805,60.4709967147976)) ;
#8193=CARTESIAN_POINT('Ctrl Pts',(22.6309062409902,56.1276240321524,60.6662120728825)) ;
#8194=CARTESIAN_POINT('Ctrl Pts',(22.7983168419127,56.0262125668428,60.6511907273074)) ;
#8195=CARTESIAN_POINT('Ctrl Pts',(22.2868305937246,55.5885108130465,60.5140535628389)) ;
#8196=CARTESIAN_POINT('Ctrl Pts',(22.3156666086983,55.5866055506163,60.708230771592)) ;
#8197=CARTESIAN_POINT('Ctrl Pts',(22.4823469794624,55.485272016298,60.6862170385931)) ;
#8198=CARTESIAN_POINT('Ctrl Pts',(22.1258777321222,55.317901160658,60.5406410241412)) ;
#8199=CARTESIAN_POINT('Ctrl Pts',(22.1587672526199,55.3159940909204,60.7341732409742)) ;
#8200=CARTESIAN_POINT('Ctrl Pts',(22.3249457959597,55.214651875968,60.7086777753867)) ;
#8201=CARTESIAN_POINT('Ctrl Pts',(21.8054571265389,54.7764805321528,60.6039693813565)) ;
#8202=CARTESIAN_POINT('Ctrl Pts',(21.846418716765,54.7745728258528,60.7959584644911)) ;
#8203=CARTESIAN_POINT('Ctrl Pts',(22.0113163449193,54.6731104541105,60.7635398914439)) ;
#8204=CARTESIAN_POINT('Ctrl Pts',(21.6460058840883,54.5052712784107,60.6407300937437)) ;
#8205=CARTESIAN_POINT('Ctrl Pts',(21.6909879829958,54.5033650627666,60.8318137773509)) ;
#8206=CARTESIAN_POINT('Ctrl Pts',(21.8552392919195,54.402027181747,60.7959300556672)) ;
#8207=CARTESIAN_POINT('Ctrl Pts',(21.3304302531076,53.9638812711429,60.723995284381)) ;
#8208=CARTESIAN_POINT('Ctrl Pts',(21.3833666353325,53.961974913084,60.9130306639828)) ;
#8209=CARTESIAN_POINT('Ctrl Pts',(21.5459580455397,53.8606102462171,60.8703104985783)) ;
#8210=CARTESIAN_POINT('Ctrl Pts',(21.1739449590052,53.6935003224017,60.7705861098554)) ;
#8211=CARTESIAN_POINT('Ctrl Pts',(21.2308267414169,53.6915946089307,60.9584728507535)) ;
#8212=CARTESIAN_POINT('Ctrl Pts',(21.3924690809887,53.5901950776532,60.9123643251348)) ;
#8213=CARTESIAN_POINT('Ctrl Pts',(20.8644295345407,53.1525885953574,60.8734112573306)) ;
#8214=CARTESIAN_POINT('Ctrl Pts',(20.9291169100103,53.1506832357842,61.0587537283216)) ;
#8215=CARTESIAN_POINT('Ctrl Pts',(21.0887268134599,53.0493503316648,61.0059167664191)) ;
#8216=CARTESIAN_POINT('Ctrl Pts',(20.7114237625881,52.882199970333,60.9296260238961)) ;
#8217=CARTESIAN_POINT('Ctrl Pts',(20.7799690600203,52.8802927777011,61.1135770768887)) ;
#8218=CARTESIAN_POINT('Ctrl Pts',(20.9384318123433,52.7789455602561,61.05741757716)) ;
#8219=CARTESIAN_POINT('Ctrl Pts',(20.4089174963609,52.3415574725868,61.0516641128343)) ;
#8220=CARTESIAN_POINT('Ctrl Pts',(20.4850932611546,52.3396495857293,61.2325923658241)) ;
#8221=CARTESIAN_POINT('Ctrl Pts',(20.6409989900421,52.2381712237815,61.1698828503062)) ;
#8222=CARTESIAN_POINT('Ctrl Pts',(20.2595076558012,52.0708923183184,61.1174628765065)) ;
#8223=CARTESIAN_POINT('Ctrl Pts',(20.3394548866061,52.0689860210861,61.2967525281003)) ;
#8224=CARTESIAN_POINT('Ctrl Pts',(20.4940904813883,51.9676510264126,61.2307636933388)) ;
#8225=CARTESIAN_POINT('Ctrl Pts',(19.9650527208262,51.5294526417529,61.2583331584609)) ;
#8226=CARTESIAN_POINT('Ctrl Pts',(20.0524312593111,51.5275461441627,61.434121987783)) ;
#8227=CARTESIAN_POINT('Ctrl Pts',(20.2041507845699,51.4261734610014,61.3617298195192)) ;
#8228=CARTESIAN_POINT('Ctrl Pts',(19.8196993362125,51.2584285629725,61.3335698183793)) ;
#8229=CARTESIAN_POINT('Ctrl Pts',(19.910747581436,51.2565228089847,61.5074867887763)) ;
#8230=CARTESIAN_POINT('Ctrl Pts',(20.0609066761106,51.155134072336,61.431931527665)) ;
#8231=CARTESIAN_POINT('Ctrl Pts',(19.5345636251539,50.716825622987,61.4927171177322)) ;
#8232=CARTESIAN_POINT('Ctrl Pts',(19.6328117475426,50.7149201642453,61.6626689874544)) ;
#8233=CARTESIAN_POINT('Ctrl Pts',(19.779704921468,50.6135869790364,61.5808800021285)) ;
#8234=CARTESIAN_POINT('Ctrl Pts',(19.3946960746612,50.4462620313475,61.5766493945011)) ;
#8235=CARTESIAN_POINT('Ctrl Pts',(19.4964757082143,50.4443547062501,61.7445107101472)) ;
#8236=CARTESIAN_POINT('Ctrl Pts',(19.6416157612327,50.3430015532564,61.6596722673663)) ;
#8237=CARTESIAN_POINT('Ctrl Pts',(19.120347271349,49.9056099883002,61.7532078208345)) ;
#8238=CARTESIAN_POINT('Ctrl Pts',(19.2290575176146,49.9037019096545,61.9166704920289)) ;
#8239=CARTESIAN_POINT('Ctrl Pts',(19.3704530768998,49.8022062837629,61.8258792263852)) ;
#8240=CARTESIAN_POINT('Ctrl Pts',(18.9859992421676,49.6350408217894,61.8457599517748)) ;
#8241=CARTESIAN_POINT('Ctrl Pts',(19.0981049563584,49.6331344367489,62.006907681661)) ;
#8242=CARTESIAN_POINT('Ctrl Pts',(19.2376494534462,49.5318014383597,61.91312930125)) ;
#8243=CARTESIAN_POINT('Ctrl Pts',(18.7234168960688,49.094225030673,62.0390565968025)) ;
#8244=CARTESIAN_POINT('Ctrl Pts',(18.8421597145869,49.0923183861909,62.1953797257233)) ;
#8245=CARTESIAN_POINT('Ctrl Pts',(18.9776400235437,48.9909365753488,62.0958671992294)) ;
#8246=CARTESIAN_POINT('Ctrl Pts',(18.5950057536361,48.8238179925609,62.1399409713884)) ;
#8247=CARTESIAN_POINT('Ctrl Pts',(18.7169956791222,48.8219121927132,62.2937435774521)) ;
#8248=CARTESIAN_POINT('Ctrl Pts',(18.8503646589018,48.7205331729861,62.191416023735)) ;
#8249=CARTESIAN_POINT('Ctrl Pts',(18.344791622651,48.2823982252904,62.3495579783263)) ;
#8250=CARTESIAN_POINT('Ctrl Pts',(18.4731096558997,48.2804926625104,62.4981204671872)) ;
#8251=CARTESIAN_POINT('Ctrl Pts',(18.6021004401867,48.1791582421601,62.3902864565594)) ;
#8252=CARTESIAN_POINT('Ctrl Pts',(18.2228959649897,48.0114576298592,62.4583587669778)) ;
#8253=CARTESIAN_POINT('Ctrl Pts',(18.3542987951968,48.0095520696155,62.6042054927202)) ;
#8254=CARTESIAN_POINT('Ctrl Pts',(18.4809339819869,47.9080609643498,62.4937510691697)) ;
#8255=CARTESIAN_POINT('Ctrl Pts',(17.9860167173073,47.4697670852059,62.6835784937478)) ;
#8256=CARTESIAN_POINT('Ctrl Pts',(18.1234139395054,47.4678622559185,62.8237875200317)) ;
#8257=CARTESIAN_POINT('Ctrl Pts',(18.2453689199781,47.3665093096488,62.7080713201897)) ;
#8258=CARTESIAN_POINT('Ctrl Pts',(17.8713622037688,47.1991192501592,62.7996706789161)) ;
#8259=CARTESIAN_POINT('Ctrl Pts',(18.0116612186128,47.1972127705363,62.9369749602238)) ;
#8260=CARTESIAN_POINT('Ctrl Pts',(18.1311767720907,47.0958808569954,62.8187239599312)) ;
#8261=CARTESIAN_POINT('Ctrl Pts',(17.6495728367388,46.6582159321309,63.0387734246909)) ;
#8262=CARTESIAN_POINT('Ctrl Pts',(17.7954894043096,46.6563091331966,63.1700945757485)) ;
#8263=CARTESIAN_POINT('Ctrl Pts',(17.909933212892,46.55491712217,63.0469754684038)) ;
#8264=CARTESIAN_POINT('Ctrl Pts',(17.5423655416169,46.387893043845,63.1618809435582)) ;
#8265=CARTESIAN_POINT('Ctrl Pts',(17.6909986176242,46.3859871917481,63.2901184799721)) ;
#8266=CARTESIAN_POINT('Ctrl Pts',(17.8028497172398,46.2846172014538,63.1646224320618)) ;
#8267=CARTESIAN_POINT('Ctrl Pts',(17.3360387404632,45.8470089936285,63.4143795876991)) ;
#8268=CARTESIAN_POINT('Ctrl Pts',(17.4899015253219,45.8451033188971,63.5362916945355)) ;
#8269=CARTESIAN_POINT('Ctrl Pts',(17.5964220062636,45.7437666877308,63.4062158185806)) ;
#8270=CARTESIAN_POINT('Ctrl Pts',(17.2368458636899,45.5765948766505,63.5438417903575)) ;
#8271=CARTESIAN_POINT('Ctrl Pts',(17.3932248689923,45.5746876691604,63.6625139851918)) ;
#8272=CARTESIAN_POINT('Ctrl Pts',(17.4969830128249,45.4732994150383,63.530260528991)) ;
#8273=CARTESIAN_POINT('Ctrl Pts',(17.1416766080821,45.3060601767044,63.6764864071842)) ;
#8274=CARTESIAN_POINT('Ctrl Pts',(17.3004704348883,45.3041537286489,63.791833369093)) ;
#8275=CARTESIAN_POINT('Ctrl Pts',(17.401402501053,45.2027271666488,63.6574852908108)) ;
#8276=CARTESIAN_POINT('Ctrl Pts',(17.0490336577126,45.1993067880441,63.8123519660661)) ;
#8277=CARTESIAN_POINT('Ctrl Pts',(17.2087077484269,45.2022941676425,63.9227233952561)) ;
#8278=CARTESIAN_POINT('Ctrl Pts',(17.1177210656172,45.3026134137914,64.06180633622)) ;
#8279=CARTESIAN_POINT('Ctrl Pts',(17.1455226949134,45.4820412744375,63.6716960182275)) ;
#8280=CARTESIAN_POINT('Ctrl Pts',(17.3027834310888,45.4850270679756,63.7855615284192)) ;
#8281=CARTESIAN_POINT('Ctrl Pts',(17.2087519082886,45.5853439255196,63.922655892153)) ;
#8282=CARTESIAN_POINT('Ctrl Pts',(17.2464212678063,45.7643410734657,63.5345175445691)) ;
#8283=CARTESIAN_POINT('Ctrl Pts',(17.401152681015,45.7673274764212,63.6517895025822)) ;
#8284=CARTESIAN_POINT('Ctrl Pts',(17.3041243260271,45.8675609242035,63.7868355301742)) ;
#8285=CARTESIAN_POINT('Ctrl Pts',(17.4565134656398,46.3280183067045,63.2675668339134)) ;
#8286=CARTESIAN_POINT('Ctrl Pts',(17.6059910908437,46.331004915594,63.3914666923995)) ;
#8287=CARTESIAN_POINT('Ctrl Pts',(17.5031785660295,46.4312549192417,63.5221510947456)) ;
#8288=CARTESIAN_POINT('Ctrl Pts',(17.5658513791384,46.6093355962106,63.1376190987605)) ;
#8289=CARTESIAN_POINT('Ctrl Pts',(17.7125968167087,46.6123217179431,63.2647451499116)) ;
#8290=CARTESIAN_POINT('Ctrl Pts',(17.6069791740221,46.712617478714,63.3931394651388)) ;
#8291=CARTESIAN_POINT('Ctrl Pts',(17.7924789756583,47.1717937445044,62.8854376933859)) ;
#8292=CARTESIAN_POINT('Ctrl Pts',(17.9335562333469,47.1747789756612,63.0188226312906)) ;
#8293=CARTESIAN_POINT('Ctrl Pts',(17.8224307838778,47.2750030883984,63.1425350068647)) ;
#8294=CARTESIAN_POINT('Ctrl Pts',(17.9097228296802,47.4527838882153,62.7632359923575)) ;
#8295=CARTESIAN_POINT('Ctrl Pts',(18.0478719290323,47.4557718391432,62.8996519815895)) ;
#8296=CARTESIAN_POINT('Ctrl Pts',(17.9340906077666,47.5560106522166,63.0209148247748)) ;
#8297=CARTESIAN_POINT('Ctrl Pts',(18.152046918103,48.0142871287591,62.5265870268212)) ;
#8298=CARTESIAN_POINT('Ctrl Pts',(18.2841480165347,48.0172768213242,62.6688740735516)) ;
#8299=CARTESIAN_POINT('Ctrl Pts',(18.165263429428,48.1176560532207,62.7850247741514)) ;
#8300=CARTESIAN_POINT('Ctrl Pts',(18.2770385109489,48.2952668191048,62.4122452341964)) ;
#8301=CARTESIAN_POINT('Ctrl Pts',(18.4060099207561,48.2982535238503,62.5573681352024)) ;
#8302=CARTESIAN_POINT('Ctrl Pts',(18.2845680798083,48.3984774868501,62.6709705308533)) ;
#8303=CARTESIAN_POINT('Ctrl Pts',(18.5341439279546,48.8569739450436,62.1919748252194)) ;
#8304=CARTESIAN_POINT('Ctrl Pts',(18.6566967270201,48.8599612929924,62.3425595457133)) ;
#8305=CARTESIAN_POINT('Ctrl Pts',(18.5304598910702,48.9602369846067,62.4507639370776)) ;
#8306=CARTESIAN_POINT('Ctrl Pts',(18.6664510738312,49.1378578224521,62.0858933183196)) ;
#8307=CARTESIAN_POINT('Ctrl Pts',(18.7856992455192,49.1408439740008,62.2391079338026)) ;
#8308=CARTESIAN_POINT('Ctrl Pts',(18.6571347380458,49.2411084827289,62.3445461273707)) ;
#8309=CARTESIAN_POINT('Ctrl Pts',(18.9376946500433,49.7002903800722,61.8825932573844)) ;
#8310=CARTESIAN_POINT('Ctrl Pts',(19.050169723931,49.7032760750642,62.0408453671987)) ;
#8311=CARTESIAN_POINT('Ctrl Pts',(18.9171280204917,49.803503874625,62.1406092424056)) ;
#8312=CARTESIAN_POINT('Ctrl Pts',(19.0766896002932,49.981574104154,61.7853116649667)) ;
#8313=CARTESIAN_POINT('Ctrl Pts',(19.1857006417587,49.9845603797215,61.9459752235339)) ;
#8314=CARTESIAN_POINT('Ctrl Pts',(19.0505798995618,50.0849206295543,62.0427767583232)) ;
#8315=CARTESIAN_POINT('Ctrl Pts',(19.3614455200386,50.5452598054505,61.599607012202)) ;
#8316=CARTESIAN_POINT('Ctrl Pts',(19.4633446760807,50.5482445256743,61.7648678207392)) ;
#8317=CARTESIAN_POINT('Ctrl Pts',(19.3240747731292,50.6484794513874,61.8557278637767)) ;
#8318=CARTESIAN_POINT('Ctrl Pts',(19.5068971693961,50.8275371605432,61.5113786134476)) ;
#8319=CARTESIAN_POINT('Ctrl Pts',(19.6051679348679,50.8305243023331,61.6788222555382)) ;
#8320=CARTESIAN_POINT('Ctrl Pts',(19.4639424629956,50.9307473366981,61.7666251609937)) ;
#8321=CARTESIAN_POINT('Ctrl Pts',(19.7297237719396,51.2516112326461,61.3860283416691)) ;
#8322=CARTESIAN_POINT('Ctrl Pts',(19.8224379405654,51.2545984104599,61.5565744041528)) ;
#8323=CARTESIAN_POINT('Ctrl Pts',(19.6784682413758,51.3548887142934,61.6396658154339)) ;
#8324=CARTESIAN_POINT('Ctrl Pts',(19.8048505346244,51.3931523912137,61.3453731396617)) ;
#8325=CARTESIAN_POINT('Ctrl Pts',(19.895690982332,51.3961391935501,61.5169252343388)) ;
#8326=CARTESIAN_POINT('Ctrl Pts',(19.7508279665644,51.4964465474925,61.5984296343693)) ;
#8327=CARTESIAN_POINT('Ctrl Pts',(19.9562473847284,51.6761627264631,61.2666350136366)) ;
#8328=CARTESIAN_POINT('Ctrl Pts',(20.0433090702939,51.6791488679163,61.4401333749345)) ;
#8329=CARTESIAN_POINT('Ctrl Pts',(19.896670741513,51.7794030062388,61.5184624170268)) ;
#8330=CARTESIAN_POINT('Ctrl Pts',(20.0325166502847,51.8176028378205,61.2285471996139)) ;
#8331=CARTESIAN_POINT('Ctrl Pts',(20.1176756133913,51.8205891355623,61.4029868205377)) ;
#8332=CARTESIAN_POINT('Ctrl Pts',(19.9701828553007,51.9208298261689,61.4797112591545)) ;
#8333=CARTESIAN_POINT('Ctrl Pts',(20.2630296190609,52.2417288193162,61.1181108441885)) ;
#8334=CARTESIAN_POINT('Ctrl Pts',(20.3424395047616,52.2447151365725,61.2952797212327)) ;
#8335=CARTESIAN_POINT('Ctrl Pts',(20.1924847498882,52.3449566194198,61.3671412503005)) ;
#8336=CARTESIAN_POINT('Ctrl Pts',(20.4190843256942,52.5241300049794,61.0495422547059)) ;
#8337=CARTESIAN_POINT('Ctrl Pts',(20.4946049613182,52.5271161388784,61.2284060668257)) ;
#8338=CARTESIAN_POINT('Ctrl Pts',(20.3431512476579,52.6274277787848,61.2969560666953)) ;
#8339=CARTESIAN_POINT('Ctrl Pts',(20.7352774289549,53.089174481225,60.9228046908309)) ;
#8340=CARTESIAN_POINT('Ctrl Pts',(20.8029106375314,53.0921595377318,61.1047944240417)) ;
#8341=CARTESIAN_POINT('Ctrl Pts',(20.6485625806559,53.1923844744817,61.1666835299605)) ;
#8342=CARTESIAN_POINT('Ctrl Pts',(20.8952932693716,53.3716654702891,60.8646724123074)) ;
#8343=CARTESIAN_POINT('Ctrl Pts',(20.958939113703,53.3746531996274,61.0480949606972)) ;
#8344=CARTESIAN_POINT('Ctrl Pts',(20.8032801065143,53.4748857690477,61.1065967793017)) ;
#8345=CARTESIAN_POINT('Ctrl Pts',(21.2191660762763,53.9365848433116,60.7588866402754)) ;
#8346=CARTESIAN_POINT('Ctrl Pts',(21.2747437665872,53.9395741566696,60.9449172512699)) ;
#8347=CARTESIAN_POINT('Ctrl Pts',(21.1167457369649,54.0399343658719,60.9965396864954)) ;
#8348=CARTESIAN_POINT('Ctrl Pts',(21.3829591038786,54.2194050937958,60.7112697291679)) ;
#8349=CARTESIAN_POINT('Ctrl Pts',(21.4344485275877,54.2223916876299,60.8984685858512)) ;
#8350=CARTESIAN_POINT('Ctrl Pts',(21.2752873587406,54.322617764982,60.9466468381776)) ;
#8351=CARTESIAN_POINT('Ctrl Pts',(21.7134230274786,54.7853172886335,60.6268523737491)) ;
#8352=CARTESIAN_POINT('Ctrl Pts',(21.7566785748286,54.7883043794258,60.8161247816509)) ;
#8353=CARTESIAN_POINT('Ctrl Pts',(21.5955845359118,54.8885704142163,60.8572908231305)) ;
#8354=CARTESIAN_POINT('Ctrl Pts',(21.8802808706122,55.0683374452623,60.5900200604226)) ;
#8355=CARTESIAN_POINT('Ctrl Pts',(21.9193783050032,55.0713235719889,60.7801950956779)) ;
#8356=CARTESIAN_POINT('Ctrl Pts',(21.7574250730561,55.1715968138679,60.8178208957825)) ;
#8357=CARTESIAN_POINT('Ctrl Pts',(22.2153336537663,55.6338317486076,60.5275072380942)) ;
#8358=CARTESIAN_POINT('Ctrl Pts',(22.2460816167474,55.6368172834239,60.7192077956619)) ;
#8359=CARTESIAN_POINT('Ctrl Pts',(22.0826126303576,55.7370429277275,60.7497260223226)) ;
#8360=CARTESIAN_POINT('Ctrl Pts',(22.3836539671604,55.9162154787364,60.5017754298194)) ;
#8361=CARTESIAN_POINT('Ctrl Pts',(22.4102134039785,55.9192018042841,60.6941060183188)) ;
#8362=CARTESIAN_POINT('Ctrl Pts',(22.2461996794021,56.0195762764982,60.7210326751055)) ;
#8363=CARTESIAN_POINT('Ctrl Pts',(22.7220464748074,56.4812254904543,60.461349008304)) ;
#8364=CARTESIAN_POINT('Ctrl Pts',(22.740172194055,56.4842101348188,60.6546523260149)) ;
#8365=CARTESIAN_POINT('Ctrl Pts',(22.5750628838645,56.5844490941092,60.6743976159306)) ;
#8366=CARTESIAN_POINT('Ctrl Pts',(22.8916830507608,56.7637439358806,60.4467024834945)) ;
#8367=CARTESIAN_POINT('Ctrl Pts',(22.9055849340659,56.7667309512735,60.6403547970455)) ;
#8368=CARTESIAN_POINT('Ctrl Pts',(22.7400743833527,56.8669533046418,60.6564901223893)) ;
#8369=CARTESIAN_POINT('Ctrl Pts',(23.2318362481627,57.3288079962322,60.428527054267)) ;
#8370=CARTESIAN_POINT('Ctrl Pts',(23.2372699125271,57.3317959922072,60.6226042851211)) ;
#8371=CARTESIAN_POINT('Ctrl Pts',(23.0712569554089,57.4320972449965,60.6314923959532)) ;
#8372=CARTESIAN_POINT('Ctrl Pts',(23.4024476603049,57.611503670388,60.4250093486565)) ;
#8373=CARTESIAN_POINT('Ctrl Pts',(23.4036306456897,57.6144899220688,60.6191573059636)) ;
#8374=CARTESIAN_POINT('Ctrl Pts',(23.2374315995444,57.7147356136583,60.624412729286)) ;
#8375=CARTESIAN_POINT('Ctrl Pts',(23.7435444880125,58.1775332619085,60.4291798819412)) ;
#8376=CARTESIAN_POINT('Ctrl Pts',(23.7362349072975,58.1805194049396,60.623193506534)) ;
#8377=CARTESIAN_POINT('Ctrl Pts',(23.5699601204502,58.2807563670397,60.6211751413546)) ;
#8378=CARTESIAN_POINT('Ctrl Pts',(23.9141929541263,58.4605262973812,60.4368761160161)) ;
#8379=CARTESIAN_POINT('Ctrl Pts',(23.9026365192723,58.4635110441036,60.6306861729615)) ;
#8380=CARTESIAN_POINT('Ctrl Pts',(23.7365085092164,58.5638587343536,60.6250289006596)) ;
#8381=CARTESIAN_POINT('Ctrl Pts',(24.0840192284084,58.7433256931628,60.4501282929911)) ;
#8382=CARTESIAN_POINT('Ctrl Pts',(24.0682327693193,58.7463119239391,60.6435880950894)) ;
#8383=CARTESIAN_POINT('Ctrl Pts',(23.9022262800894,58.846513767945,60.634300421317)) ;
#8384=CARTESIAN_POINT('Origin',(-4.80851752474837,45.3830586252741,88.8353684199565)) ;
#8385=CARTESIAN_POINT('',(17.1688786268051,45.3830610445957,72.8060570186675)) ;
#8386=CARTESIAN_POINT('',(0.569856645481987,45.3830586252741,84.8659474548835)) ;
#8387=CARTESIAN_POINT('',(17.1688762698447,45.3830586252741,72.8060537745881)) ;
#8388=CARTESIAN_POINT('Ctrl Pts',(17.1688794847748,45.3830586252741,72.8060581995622)) ;
#8389=CARTESIAN_POINT('Ctrl Pts',(17.1800655091625,45.3830586252741,72.7979310784706)) ;
#8390=CARTESIAN_POINT('Ctrl Pts',(17.1901949893514,45.3830586252741,72.7885022675957)) ;
#8391=CARTESIAN_POINT('Ctrl Pts',(17.2087915183656,45.3830586252741,72.7665630539906)) ;
#8392=CARTESIAN_POINT('Ctrl Pts',(17.2169373449558,45.3830586252741,72.7540141333136)) ;
#8393=CARTESIAN_POINT('Ctrl Pts',(17.2355140967823,45.3830586252741,72.7162404357135)) ;
#8394=CARTESIAN_POINT('Ctrl Pts',(17.2421115176057,45.3830586252741,72.6895919213799)) ;
#8395=CARTESIAN_POINT('Ctrl Pts',(17.2455991389693,45.3830586252741,72.6330329519167)) ;
#8396=CARTESIAN_POINT('Ctrl Pts',(17.2416418239109,45.3830586252736,72.6034108053733)) ;
#8397=CARTESIAN_POINT('Ctrl Pts',(17.2249824939971,45.3830586252736,72.5497711522179)) ;
#8398=CARTESIAN_POINT('Ctrl Pts',(17.2131755915674,45.3830586252741,72.5255254786368)) ;
#8399=CARTESIAN_POINT('Ctrl Pts',(17.1981507140927,45.3830586252741,72.5034867616281)) ;
#8400=CARTESIAN_POINT('',(17.2299597049927,45.3830674541111,72.8852989434337)) ;
#8401=CARTESIAN_POINT('Ctrl Pts',(17.5258214295105,45.3830586252741,72.9484557918475)) ;
#8402=CARTESIAN_POINT('Ctrl Pts',(17.5095041570387,45.3830586252741,72.9279068266439)) ;
#8403=CARTESIAN_POINT('Ctrl Pts',(17.4902242692681,45.3830586252745,72.9096981137126)) ;
#8404=CARTESIAN_POINT('Ctrl Pts',(17.4444073336212,45.3830586252745,72.8778489307896)) ;
#8405=CARTESIAN_POINT('Ctrl Pts',(17.4172953260424,45.3830586252741,72.8651171123935)) ;
#8406=CARTESIAN_POINT('Ctrl Pts',(17.3621978432612,45.3830586252741,72.8513607012809)) ;
#8407=CARTESIAN_POINT('Ctrl Pts',(17.3347399628247,45.3830586252741,72.849611691816)) ;
#8408=CARTESIAN_POINT('Ctrl Pts',(17.2932911066477,45.3830586252741,72.8559099542529)) ;
#8409=CARTESIAN_POINT('Ctrl Pts',(17.2790818332707,45.3830586252741,72.8598039396343)) ;
#8410=CARTESIAN_POINT('Ctrl Pts',(17.2529022556706,45.3830586252741,72.8706466438317)) ;
#8411=CARTESIAN_POINT('Ctrl Pts',(17.2409892021835,45.3830586252741,72.8772920314038)) ;
#8412=CARTESIAN_POINT('Ctrl Pts',(17.2299628898897,45.3830586252741,72.8853032108675)) ;
#8413=CARTESIAN_POINT('',(1.58245214009829,45.3830586252741,84.2538605621281)) ;
#8414=CARTESIAN_POINT('',(1.58245214009829,45.3830586252741,84.2538605621281)) ;
#8415=CARTESIAN_POINT('Origin',(-2.53204462594907,45.3830586252741,78.5907416015035)) ;
#8416=CARTESIAN_POINT('Ctrl Pts',(17.4100634185147,45.3830502402116,72.6308270694242)) ;
#8417=CARTESIAN_POINT('Ctrl Pts',(17.2062496612647,45.9804808943695,72.3503018815983)) ;
#8418=CARTESIAN_POINT('Ctrl Pts',(17.0291891298972,46.5779115664506,72.0521676888577)) ;
#8419=CARTESIAN_POINT('Ctrl Pts',(16.8521298437262,47.1753380370388,71.7540355927766)) ;
#8420=CARTESIAN_POINT('Ctrl Pts',(16.703334020664,47.772764507627,71.4408383057955)) ;
#8421=CARTESIAN_POINT('Ctrl Pts',(16.5545381976019,48.3701909782152,71.1276410188143)) ;
#8422=CARTESIAN_POINT('Ctrl Pts',(16.435275311147,48.9676174488035,70.8020506297554)) ;
#8423=CARTESIAN_POINT('Ctrl Pts',(16.3160124246922,49.5650439193917,70.4764602406964)) ;
#8424=CARTESIAN_POINT('Ctrl Pts',(16.2272999837411,50.16247038998,70.1412545719592)) ;
#8425=CARTESIAN_POINT('Ctrl Pts',(16.1385875427899,50.7598968605682,69.8060489032219)) ;
#8426=CARTESIAN_POINT('Ctrl Pts',(16.0811824106094,51.3573233311564,69.4640878113819)) ;
#8427=CARTESIAN_POINT('Ctrl Pts',(16.023777278429,51.9547498017447,69.1221267195418)) ;
#8428=CARTESIAN_POINT('Ctrl Pts',(15.9981692153665,52.5521762723329,68.7763276960625)) ;
#8429=CARTESIAN_POINT('Ctrl Pts',(15.9725611523041,53.1496027429211,68.4305286725831)) ;
#8430=CARTESIAN_POINT('Ctrl Pts',(15.9789686373246,53.7470292135094,68.0838419528074)) ;
#8431=CARTESIAN_POINT('Ctrl Pts',(15.985376122345,54.3444556840976,67.7371552330318)) ;
#8432=CARTESIAN_POINT('Ctrl Pts',(16.0237444890454,54.9418821546858,67.3925386258147)) ;
#8433=CARTESIAN_POINT('Ctrl Pts',(16.0621128557458,55.5393086252741,67.0479220185975)) ;
#8434=CARTESIAN_POINT('Ctrl Pts',(16.1321147587497,56.1367350958623,66.7083156713233)) ;
#8435=CARTESIAN_POINT('Ctrl Pts',(16.2021166617536,56.7341615664506,66.3687093240491)) ;
#8436=CARTESIAN_POINT('Ctrl Pts',(16.3031548695066,57.3315880370388,66.037010638331)) ;
#8437=CARTESIAN_POINT('Ctrl Pts',(16.3920498868663,57.8572133193466,65.7451768748386)) ;
#8438=CARTESIAN_POINT('Ctrl Pts',(16.5043534680133,58.3830758086166,65.4615271343363)) ;
#8439=CARTESIAN_POINT('Ctrl Pts',(-4.83789343805113,45.3830502402116,88.7949359439767)) ;
#8440=CARTESIAN_POINT('Ctrl Pts',(-5.78902430521799,45.9804808943695,87.4858184007887)) ;
#8441=CARTESIAN_POINT('Ctrl Pts',(-6.6153067849329,46.5779115664506,86.0945255013329)) ;
#8442=CARTESIAN_POINT('Ctrl Pts',(-7.44158345373106,47.1753380370388,84.7032423862879)) ;
#8443=CARTESIAN_POINT('Ctrl Pts',(-8.13596396135441,47.772764507627,83.2416550470425)) ;
#8444=CARTESIAN_POINT('Ctrl Pts',(-8.83034446897775,48.3701909782152,81.7800677077971)) ;
#8445=CARTESIAN_POINT('Ctrl Pts',(-9.38690460576691,48.9676174488035,80.2606458921887)) ;
#8446=CARTESIAN_POINT('Ctrl Pts',(-9.94346474255606,49.5650439193917,78.7412240765802)) ;
#8447=CARTESIAN_POINT('Ctrl Pts',(-10.3574561336615,50.16247038998,77.1769309558065)) ;
#8448=CARTESIAN_POINT('Ctrl Pts',(-10.771447524767,50.7598968605682,75.6126378350327)) ;
#8449=CARTESIAN_POINT('Ctrl Pts',(-11.0393381416091,51.3573233311564,74.0168194064458)) ;
#8450=CARTESIAN_POINT('Ctrl Pts',(-11.3072287584512,51.9547498017447,72.4210009778589)) ;
#8451=CARTESIAN_POINT('Ctrl Pts',(-11.4267330527426,52.5521762723329,70.8072722016218)) ;
#8452=CARTESIAN_POINT('Ctrl Pts',(-11.546237347034,53.1496027429211,69.1935434253848)) ;
#8453=CARTESIAN_POINT('Ctrl Pts',(-11.5163357502719,53.7470292135094,67.5756720664317)) ;
#8454=CARTESIAN_POINT('Ctrl Pts',(-11.4864341535098,54.3444556840976,65.9578007074786)) ;
#8455=CARTESIAN_POINT('Ctrl Pts',(-11.3073817755747,54.9418821546858,64.3495898737987)) ;
#8456=CARTESIAN_POINT('Ctrl Pts',(-11.1283293976396,55.5393086252741,62.7413790401188)) ;
#8457=CARTESIAN_POINT('Ctrl Pts',(-10.8016538502879,56.1367350958623,61.1565494195059)) ;
#8458=CARTESIAN_POINT('Ctrl Pts',(-10.4749783029363,56.7341615664506,59.5717197988929)) ;
#8459=CARTESIAN_POINT('Ctrl Pts',(-10.0034666667556,57.3315880370388,58.0237925988748)) ;
#8460=CARTESIAN_POINT('Ctrl Pts',(-9.5886232524106,57.8572133193466,56.6619017025771)) ;
#8461=CARTESIAN_POINT('Ctrl Pts',(-9.06453987372463,58.3830758086166,55.3382029135661)) ;
#8462=CARTESIAN_POINT('',(-1.74213662306825,58.3353824278239,58.3447753707129)) ;
#8463=CARTESIAN_POINT('',(16.1909549772416,58.2172712656977,65.4449915594351)) ;
#8464=CARTESIAN_POINT('Ctrl Pts',(-1.74213662306824,58.3353824278239,58.3447753707129)) ;
#8465=CARTESIAN_POINT('Ctrl Pts',(0.655926738612619,58.3308357090662,59.2942358214405)) ;
#8466=CARTESIAN_POINT('Ctrl Pts',(3.34356255401777,58.3244410141138,60.3583461170491)) ;
#8467=CARTESIAN_POINT('Ctrl Pts',(7.96103805230599,58.3066351840461,62.1865339947686)) ;
#8468=CARTESIAN_POINT('Ctrl Pts',(13.032674621552,58.2895264446023,64.1945369607899)) ;
#8469=CARTESIAN_POINT('Ctrl Pts',(16.1909559533793,58.2172696107886,65.4449889983622)) ;
#8470=CARTESIAN_POINT('Ctrl Pts',(16.1909549772416,58.2172712656977,65.4449915594351)) ;
#8471=CARTESIAN_POINT('Ctrl Pts',(16.1334478652878,57.9495340002375,65.5958675064122)) ;
#8472=CARTESIAN_POINT('Ctrl Pts',(16.080655138304,57.6819084045915,65.7484708734625)) ;
#8473=CARTESIAN_POINT('Ctrl Pts',(16.0326859680853,57.4145313636589,65.9024028922281)) ;
#8474=CARTESIAN_POINT('Ctrl Pts',(15.9881564338053,57.1663266301679,66.0452971944471)) ;
#8475=CARTESIAN_POINT('Ctrl Pts',(15.947768065655,56.9182638872712,66.189377214873)) ;
#8476=CARTESIAN_POINT('Ctrl Pts',(15.9115671974444,56.6702295478714,66.3344521043164)) ;
#8477=CARTESIAN_POINT('Ctrl Pts',(15.9087709003504,56.6510704023379,66.3456582579757)) ;
#8478=CARTESIAN_POINT('Ctrl Pts',(15.9059993799389,56.6319118940954,66.3568711437602)) ;
#8479=CARTESIAN_POINT('Ctrl Pts',(15.9032526664099,56.6127538456679,66.3680906454984)) ;
#8480=CARTESIAN_POINT('Ctrl Pts',(15.8672287819349,56.3614909032359,66.5152374193485)) ;
#8481=CARTESIAN_POINT('Ctrl Pts',(15.8354773115596,56.1103350670462,66.6635060977565)) ;
#8482=CARTESIAN_POINT('Ctrl Pts',(15.8080789997499,55.8590202585561,66.8125541649163)) ;
#8483=CARTESIAN_POINT('Ctrl Pts',(15.8063435636936,55.8431017310511,66.8219950162967)) ;
#8484=CARTESIAN_POINT('Ctrl Pts',(15.8046256056966,55.8271830724927,66.8314387157162)) ;
#8485=CARTESIAN_POINT('Ctrl Pts',(15.8029251298318,55.8112643008986,66.8408852528386)) ;
#8486=CARTESIAN_POINT('Ctrl Pts',(15.7757327417881,55.5567064895585,66.9919452639956)) ;
#8487=CARTESIAN_POINT('Ctrl Pts',(15.7529984536135,55.3019957844106,67.1438046094493)) ;
#8488=CARTESIAN_POINT('Ctrl Pts',(15.7347441072865,55.0471908391173,67.296431137788)) ;
#8489=CARTESIAN_POINT('Ctrl Pts',(15.7338348512874,55.034498906963,67.3040335237636)) ;
#8490=CARTESIAN_POINT('Ctrl Pts',(15.7329367612736,55.0218058655745,67.3116377919328)) ;
#8491=CARTESIAN_POINT('Ctrl Pts',(15.7320498443767,55.0091118266697,67.3192438421358)) ;
#8492=CARTESIAN_POINT('Ctrl Pts',(15.7140153711204,54.7509925981973,67.4739044529036)) ;
#8493=CARTESIAN_POINT('Ctrl Pts',(15.7006099199141,54.4926055130988,67.6292151883789)) ;
#8494=CARTESIAN_POINT('Ctrl Pts',(15.6918744372802,54.2345762733044,67.7845220130878)) ;
#8495=CARTESIAN_POINT('Ctrl Pts',(15.6915555684979,54.2251575070004,67.7901911329461)) ;
#8496=CARTESIAN_POINT('Ctrl Pts',(15.6912428906292,54.2157389752755,67.7958606956662)) ;
#8497=CARTESIAN_POINT('Ctrl Pts',(15.6909364038727,54.2063206495465,67.8015306898383)) ;
#8498=CARTESIAN_POINT('Ctrl Pts',(15.6824344247839,53.9450551732693,67.9588170027652)) ;
#8499=CARTESIAN_POINT('Ctrl Pts',(15.6787014922471,53.6840579939704,68.1163692599084)) ;
#8500=CARTESIAN_POINT('Ctrl Pts',(15.6797376472066,53.4230444575824,68.2737467183678)) ;
#8501=CARTESIAN_POINT('Ctrl Pts',(15.6797621169394,53.4168803877747,68.2774633288299)) ;
#8502=CARTESIAN_POINT('Ctrl Pts',(15.6797892402505,53.4107163826999,68.2811798266539)) ;
#8503=CARTESIAN_POINT('Ctrl Pts',(15.6798190170839,53.4045524432163,68.2848962113249)) ;
#8504=CARTESIAN_POINT('Ctrl Pts',(15.6810956661459,53.1402803009609,68.4442321264586)) ;
#8505=CARTESIAN_POINT('Ctrl Pts',(15.6872500775662,52.8760533725399,68.6034054826552)) ;
#8506=CARTESIAN_POINT('Ctrl Pts',(15.6982860026285,52.6118787196959,68.7624120508549)) ;
#8507=CARTESIAN_POINT('Ctrl Pts',(15.7095641185038,52.3419065760594,68.9249081253533)) ;
#8508=CARTESIAN_POINT('Ctrl Pts',(15.7259450053447,52.0715787920596,69.0871364559427)) ;
#8509=CARTESIAN_POINT('Ctrl Pts',(15.7473979457536,51.8011908422987,69.248727102498)) ;
#8510=CARTESIAN_POINT('Ctrl Pts',(15.7474248784871,51.8008513882914,69.2489299687594)) ;
#8511=CARTESIAN_POINT('Ctrl Pts',(15.7474518192137,51.8005119341974,69.249132834011)) ;
#8512=CARTESIAN_POINT('Ctrl Pts',(15.7474787679334,51.8001724800174,69.2493356982519)) ;
#8513=CARTESIAN_POINT('Ctrl Pts',(15.768687011999,51.5330270582814,69.4089868570238)) ;
#8514=CARTESIAN_POINT('Ctrl Pts',(15.7949064956035,51.265585354454,69.5683471237062)) ;
#8515=CARTESIAN_POINT('Ctrl Pts',(15.825976232437,50.9984015502859,69.7264176065219)) ;
#8516=CARTESIAN_POINT('Ctrl Pts',(15.8263938754657,50.9948100344075,69.7285424084002)) ;
#8517=CARTESIAN_POINT('Ctrl Pts',(15.8268123967231,50.9912185474961,69.7306669877117)) ;
#8518=CARTESIAN_POINT('Ctrl Pts',(15.8272317958496,50.9876270907846,69.7327913420942)) ;
#8519=CARTESIAN_POINT('Ctrl Pts',(15.8580524204697,50.7236996475837,69.8889049933665)) ;
#8520=CARTESIAN_POINT('Ctrl Pts',(15.8936084612277,50.4599498020535,70.0438872783466)) ;
#8521=CARTESIAN_POINT('Ctrl Pts',(15.9338929720513,50.1963788513667,70.1977390376298)) ;
#8522=CARTESIAN_POINT('Ctrl Pts',(15.9349345190615,50.1895642834339,70.2017168404282)) ;
#8523=CARTESIAN_POINT('Ctrl Pts',(15.9359792010563,50.1827500045963,70.205693788537)) ;
#8524=CARTESIAN_POINT('Ctrl Pts',(15.9370270183765,50.175936008737,70.2096698856566)) ;
#8525=CARTESIAN_POINT('Ctrl Pts',(15.9770577136676,49.915614875762,70.3615722537204)) ;
#8526=CARTESIAN_POINT('Ctrl Pts',(16.021633457865,49.6552611188172,70.51209499173)) ;
#8527=CARTESIAN_POINT('Ctrl Pts',(16.0707233750742,49.3948957256021,70.6611910631829)) ;
#8528=CARTESIAN_POINT('Ctrl Pts',(16.0726253546305,49.3848079176934,70.6669677622679)) ;
#8529=CARTESIAN_POINT('Ctrl Pts',(16.0745340756922,49.3747203101762,70.6727421930359)) ;
#8530=CARTESIAN_POINT('Ctrl Pts',(16.0764495328902,49.3646329259558,70.6785143401714)) ;
#8531=CARTESIAN_POINT('Ctrl Pts',(16.1252659004566,49.1075509841677,70.8256203452038)) ;
#8532=CARTESIAN_POINT('Ctrl Pts',(16.1785286510604,48.8504690628025,70.9714340403597)) ;
#8533=CARTESIAN_POINT('Ctrl Pts',(16.2360875883058,48.5931578990175,71.1155086094327)) ;
#8534=CARTESIAN_POINT('Ctrl Pts',(16.2390736559674,48.5798089981879,71.1229829727923)) ;
#8535=CARTESIAN_POINT('Ctrl Pts',(16.2420713782267,48.5664590689811,71.1304528859902)) ;
#8536=CARTESIAN_POINT('Ctrl Pts',(16.2450807296188,48.553108105864,71.1379182711826)) ;
#8537=CARTESIAN_POINT('Ctrl Pts',(16.302355237528,48.2990102146508,71.2800008024469)) ;
#8538=CARTESIAN_POINT('Ctrl Pts',(16.3638763057718,48.0446012919296,71.4205384228564)) ;
#8539=CARTESIAN_POINT('Ctrl Pts',(16.4295089824108,47.7903648312085,71.5591745911328)) ;
#8540=CARTESIAN_POINT('Ctrl Pts',(16.4337903177685,47.7737805380753,71.5682180731221)) ;
#8541=CARTESIAN_POINT('Ctrl Pts',(16.4380893087519,47.7571963611372,71.5772538003855)) ;
#8542=CARTESIAN_POINT('Ctrl Pts',(16.4424059394334,47.7406123516807,71.5862817190454)) ;
#8543=CARTESIAN_POINT('Ctrl Pts',(16.5077400019093,47.4896062337423,71.7229231519758)) ;
#8544=CARTESIAN_POINT('Ctrl Pts',(16.5769345851249,47.2387261489801,71.8574206887935)) ;
#8545=CARTESIAN_POINT('Ctrl Pts',(16.649994480359,46.9878897404754,71.9898280933001)) ;
#8546=CARTESIAN_POINT('Ctrl Pts',(16.6557445125371,46.968148165214,72.000248951886)) ;
#8547=CARTESIAN_POINT('Ctrl Pts',(16.6615183268011,46.9484074501544,72.0106565466277)) ;
#8548=CARTESIAN_POINT('Ctrl Pts',(16.6673159147512,46.9286675886394,72.0210508865765)) ;
#8549=CARTESIAN_POINT('Ctrl Pts',(16.7400494655528,46.6810214584449,72.1514529191488)) ;
#8550=CARTESIAN_POINT('Ctrl Pts',(16.816583194872,46.4334531760668,72.2798518018417)) ;
#8551=CARTESIAN_POINT('Ctrl Pts',(16.8967060985225,46.1857600468479,72.4058931251787)) ;
#8552=CARTESIAN_POINT('Ctrl Pts',(16.9040710432613,46.1629919477681,72.4174789182401)) ;
#8553=CARTESIAN_POINT('Ctrl Pts',(16.9114664718038,46.1402223084085,72.4290450372909)) ;
#8554=CARTESIAN_POINT('Ctrl Pts',(16.918892209119,46.1174510138863,72.4405911830445)) ;
#8555=CARTESIAN_POINT('Ctrl Pts',(16.9986900450414,45.8727480373458,72.5646674067618)) ;
#8556=CARTESIAN_POINT('Ctrl Pts',(17.0820250603088,45.6279743432131,72.6865119727705)) ;
#8557=CARTESIAN_POINT('Ctrl Pts',(17.1688786268051,45.3830610445957,72.8060570186675)) ;
#8558=CARTESIAN_POINT('',(-9.01576415853505,48.5844537758935,81.2291845178394)) ;
#8559=CARTESIAN_POINT('Ctrl Pts',(0.569856645481997,45.3830586252741,84.8659474548835)) ;
#8560=CARTESIAN_POINT('Ctrl Pts',(0.101768125792855,45.4231929016305,85.0973286092697)) ;
#8561=CARTESIAN_POINT('Ctrl Pts',(-0.388741206423391,45.4870033446879,85.2745890054788)) ;
#8562=CARTESIAN_POINT('Ctrl Pts',(-1.40461265481983,45.6539797372436,85.5194765725832)) ;
#8563=CARTESIAN_POINT('Ctrl Pts',(-1.92697987875259,45.7573388893142,85.5840021976)) ;
#8564=CARTESIAN_POINT('Ctrl Pts',(-3.36578195558735,46.0833507061679,85.6012198119695)) ;
#8565=CARTESIAN_POINT('Ctrl Pts',(-4.26787911740062,46.3336877227692,85.4315724216581)) ;
#8566=CARTESIAN_POINT('Ctrl Pts',(-6.01413017476312,46.9107591797134,84.7414207150381)) ;
#8567=CARTESIAN_POINT('Ctrl Pts',(-6.83158725253899,47.2383195349503,84.1982764868229)) ;
#8568=CARTESIAN_POINT('Ctrl Pts',(-8.15849876575339,47.9083523080808,82.8562179605577)) ;
#8569=CARTESIAN_POINT('Ctrl Pts',(-8.66956683354584,48.2450338483642,82.0799311245838)) ;
#8570=CARTESIAN_POINT('Ctrl Pts',(-9.01576415853505,48.5844537758935,81.2291845178394)) ;
#8571=CARTESIAN_POINT('',(-9.03437826004907,48.6029307720944,81.1827788925151)) ;
#8572=CARTESIAN_POINT('Origin',(-42.1505219076146,48.3660423604261,94.3834385474725)) ;
#8573=CARTESIAN_POINT('',(-11.2680762515848,55.0677871747466,64.0109179234559)) ;
#8574=CARTESIAN_POINT('Ctrl Pts',(-9.03437826004907,48.6029307720944,81.1827788925151)) ;
#8575=CARTESIAN_POINT('Ctrl Pts',(-9.21711120032186,48.785356686239,80.7241857458836)) ;
#8576=CARTESIAN_POINT('Ctrl Pts',(-9.38690460576691,48.9676174488035,80.2606458921887)) ;
#8577=CARTESIAN_POINT('Ctrl Pts',(-9.94346474255606,49.5650439193917,78.7412240765802)) ;
#8578=CARTESIAN_POINT('Ctrl Pts',(-10.3574561336615,50.16247038998,77.1769309558065)) ;
#8579=CARTESIAN_POINT('Ctrl Pts',(-10.771447524767,50.7598968605682,75.6126378350327)) ;
#8580=CARTESIAN_POINT('Ctrl Pts',(-11.0393381416091,51.3573233311564,74.0168194064458)) ;
#8581=CARTESIAN_POINT('Ctrl Pts',(-11.3072287584512,51.9547498017447,72.4210009778589)) ;
#8582=CARTESIAN_POINT('Ctrl Pts',(-11.4267330527426,52.5521762723329,70.8072722016218)) ;
#8583=CARTESIAN_POINT('Ctrl Pts',(-11.546237347034,53.1496027429211,69.1935434253848)) ;
#8584=CARTESIAN_POINT('Ctrl Pts',(-11.5163357502719,53.7470292135094,67.5756720664317)) ;
#8585=CARTESIAN_POINT('Ctrl Pts',(-11.4864341535098,54.3444556840976,65.9578007074786)) ;
#8586=CARTESIAN_POINT('Ctrl Pts',(-11.3073817755747,54.9418821546858,64.3495898737987)) ;
#8587=CARTESIAN_POINT('Ctrl Pts',(-11.2885183223426,55.0048219850164,64.1801623007153)) ;
#8588=CARTESIAN_POINT('Ctrl Pts',(-11.2680762515848,55.0677871747466,64.0109179234559)) ;
#8589=CARTESIAN_POINT('',(-11.2619535028072,55.0862551252693,63.9612945541202)) ;
#8590=CARTESIAN_POINT('Origin',(-46.060912756941,55.539936013522,59.793693489166)) ;
#8591=CARTESIAN_POINT('Ctrl Pts',(-11.2619535028072,55.0862551252693,63.9612945541202)) ;
#8592=CARTESIAN_POINT('Ctrl Pts',(-11.1929984329768,55.2861476427457,63.4245274809913)) ;
#8593=CARTESIAN_POINT('Ctrl Pts',(-11.0619746721449,55.4856144064207,62.8971457747828)) ;
#8594=CARTESIAN_POINT('Ctrl Pts',(-10.6668298706646,55.8948727823204,61.8461329491164)) ;
#8595=CARTESIAN_POINT('Ctrl Pts',(-10.3950419897871,56.1030297966037,61.3286333190244)) ;
#8596=CARTESIAN_POINT('Ctrl Pts',(-9.51301503825525,56.6395229540353,60.0635523254179)) ;
#8597=CARTESIAN_POINT('Ctrl Pts',(-8.80490372629695,56.9553077214544,59.3921412545655)) ;
#8598=CARTESIAN_POINT('Ctrl Pts',(-7.21100071989772,57.5027528833965,58.415849551118)) ;
#8599=CARTESIAN_POINT('Ctrl Pts',(-6.35541866395493,57.7356392971192,58.0938755668734)) ;
#8600=CARTESIAN_POINT('Ctrl Pts',(-4.79055478616098,58.0583687617078,57.8368826753342)) ;
#8601=CARTESIAN_POINT('Ctrl Pts',(-4.11027061379133,58.1679507457142,57.8232388884774)) ;
#8602=CARTESIAN_POINT('Ctrl Pts',(-2.8560896867665,58.3023925284601,57.9829957173458)) ;
#8603=CARTESIAN_POINT('Ctrl Pts',(-2.28720555794782,58.3364158763933,58.1289673129034)) ;
#8604=CARTESIAN_POINT('Ctrl Pts',(-1.74213662306824,58.3353824278239,58.3447753707129)) ;
#8605=CARTESIAN_POINT('Ctrl Pts',(-4.7791282454143,45.3830585852922,88.8758193913844)) ;
#8606=CARTESIAN_POINT('Ctrl Pts',(-5.73399192312948,45.9804850758286,87.569427889715)) ;
#8607=CARTESIAN_POINT('Ctrl Pts',(-6.56424371575999,46.5779115664506,86.1805055162587)) ;
#8608=CARTESIAN_POINT('Ctrl Pts',(-7.39449548054943,47.1753380370388,84.7915831893776)) ;
#8609=CARTESIAN_POINT('Ctrl Pts',(-8.09305195315626,47.772764507627,83.3319797920042)) ;
#8610=CARTESIAN_POINT('Ctrl Pts',(-8.79160842576309,48.3701909782153,81.8723763946309)) ;
#8611=CARTESIAN_POINT('Ctrl Pts',(-9.35250976866712,48.9676174488035,80.35454474831)) ;
#8612=CARTESIAN_POINT('Ctrl Pts',(-9.91341111157114,49.5650439193917,78.836713101989)) ;
#8613=CARTESIAN_POINT('Ctrl Pts',(-10.331871912283,50.16247038998,77.2736028111546)) ;
#8614=CARTESIAN_POINT('Ctrl Pts',(-10.7503327129948,50.7598968605682,75.7104925203202)) ;
#8615=CARTESIAN_POINT('Ctrl Pts',(-11.0227828115078,51.3573233311564,74.1154394908365)) ;
#8616=CARTESIAN_POINT('Ctrl Pts',(-11.2952329100208,51.9547498017447,72.5203864613528)) ;
#8617=CARTESIAN_POINT('Ctrl Pts',(-11.4193478581578,52.5521762723329,70.9069991232676)) ;
#8618=CARTESIAN_POINT('Ctrl Pts',(-11.5434628062947,53.1496027429211,69.2936117851824)) ;
#8619=CARTESIAN_POINT('Ctrl Pts',(-11.5181836990798,53.7470292135094,67.6756549903998)) ;
#8620=CARTESIAN_POINT('Ctrl Pts',(-11.4929045918648,54.3444556840976,66.0576981956171)) ;
#8621=CARTESIAN_POINT('Ctrl Pts',(-11.3184471017276,54.9418821546858,64.4489757810347)) ;
#8622=CARTESIAN_POINT('Ctrl Pts',(-11.1439896115904,55.5393086252741,62.8402533664523)) ;
#8623=CARTESIAN_POINT('Ctrl Pts',(-10.8218421483247,56.1367350958623,61.2544903844918)) ;
#8624=CARTESIAN_POINT('Ctrl Pts',(-10.499694685059,56.7341615664506,59.6687274025313)) ;
#8625=CARTESIAN_POINT('Ctrl Pts',(-10.0326056972355,57.3315880370388,58.1194530238305)) ;
#8626=CARTESIAN_POINT('Ctrl Pts',(-9.62163662282806,57.8572347768351,56.7563212137985)) ;
#8627=CARTESIAN_POINT('Ctrl Pts',(-9.10130960571656,58.3831186720347,55.4310726684666)) ;
#8628=CARTESIAN_POINT('Ctrl Pts',(17.4688390970673,45.3830585852922,72.7117248502237)) ;
#8629=CARTESIAN_POINT('Ctrl Pts',(17.2612866360714,45.9804850758286,72.4339189895196)) ;
#8630=CARTESIAN_POINT('Ctrl Pts',(17.0802522492153,46.5779115664506,72.1381476740026)) ;
#8631=CARTESIAN_POINT('Ctrl Pts',(16.8992178684299,47.1753380370388,71.8423763684038)) ;
#8632=CARTESIAN_POINT('Ctrl Pts',(16.7462460815413,47.772764507627,71.5311630257302)) ;
#8633=CARTESIAN_POINT('Ctrl Pts',(16.5932742946527,48.3701909782152,71.2199496830565)) ;
#8634=CARTESIAN_POINT('Ctrl Pts',(16.4696702030105,48.9676174488035,70.8959494658169)) ;
#8635=CARTESIAN_POINT('Ctrl Pts',(16.3460661113682,49.5650439193917,70.5719492485774)) ;
#8636=CARTESIAN_POINT('Ctrl Pts',(16.2528842615005,50.16247038998,70.2379264123862)) ;
#8637=CARTESIAN_POINT('Ctrl Pts',(16.1597024116328,50.7598968605682,69.9039035761949)) ;
#8638=CARTESIAN_POINT('Ctrl Pts',(16.0977377982279,51.3573233311564,69.5627078861173)) ;
#8639=CARTESIAN_POINT('Ctrl Pts',(16.0357731848229,51.9547498017447,69.2215121960397)) ;
#8640=CARTESIAN_POINT('Ctrl Pts',(16.005554468114,52.5521762723329,68.8760546134011)) ;
#8641=CARTESIAN_POINT('Ctrl Pts',(15.9753357514052,53.1496027429211,68.5305970307626)) ;
#8642=CARTESIAN_POINT('Ctrl Pts',(15.9771207468286,53.7470292135094,68.1838248778533)) ;
#8643=CARTESIAN_POINT('Ctrl Pts',(15.9789057422521,54.3444556840976,67.837052724944)) ;
#8644=CARTESIAN_POINT('Ctrl Pts',(16.0126792208562,54.9418821546858,67.4919245395043)) ;
#8645=CARTESIAN_POINT('Ctrl Pts',(16.0464526994604,55.5393086252741,67.1467963540644)) ;
#8646=CARTESIAN_POINT('Ctrl Pts',(16.111926517834,56.1367350958623,66.8062566480835)) ;
#8647=CARTESIAN_POINT('Ctrl Pts',(16.1774003362076,56.7341615664506,66.4657169421026)) ;
#8648=CARTESIAN_POINT('Ctrl Pts',(16.2740158948177,57.3315880370388,66.1326710802811)) ;
#8649=CARTESIAN_POINT('Ctrl Pts',(16.3590232654268,57.8572347768351,65.8396400880374)) ;
#8650=CARTESIAN_POINT('Ctrl Pts',(16.4675502256468,58.3831186720347,65.5544816857789)) ;
#8651=CARTESIAN_POINT('',(16.1930072121277,58.3830537363184,65.4457829320825)) ;
#8652=CARTESIAN_POINT('Ctrl Pts',(17.2299597049927,45.3830674541111,72.8852989434337)) ;
#8653=CARTESIAN_POINT('Ctrl Pts',(17.2238785641997,45.3999249614351,72.8771508356198)) ;
#8654=CARTESIAN_POINT('Ctrl Pts',(17.217728287818,45.4170195560986,72.8688763511221)) ;
#8655=CARTESIAN_POINT('Ctrl Pts',(17.2055481051456,45.4509660823354,72.8524212486401)) ;
#8656=CARTESIAN_POINT('Ctrl Pts',(17.1994751008465,45.467937485669,72.844182883773)) ;
#8657=CARTESIAN_POINT('Ctrl Pts',(17.1813073904012,45.5188462146265,72.8194355027519)) ;
#8658=CARTESIAN_POINT('Ctrl Pts',(17.1692639864156,45.5527780591987,72.802894200399)) ;
#8659=CARTESIAN_POINT('Ctrl Pts',(17.1333393268993,45.6545524513436,72.7531423773599)) ;
#8660=CARTESIAN_POINT('Ctrl Pts',(17.1096636365158,45.7223738576061,72.719803931897)) ;
#8661=CARTESIAN_POINT('Ctrl Pts',(17.0567938513938,45.8755455989764,72.644103518881)) ;
#8662=CARTESIAN_POINT('Ctrl Pts',(17.0277600220691,45.960883422686,72.601642091708)) ;
#8663=CARTESIAN_POINT('Ctrl Pts',(16.982348309643,46.0963466756233,72.5337991217255)) ;
#8664=CARTESIAN_POINT('Ctrl Pts',(16.9656789302262,46.1464973799211,72.5085794918992)) ;
#8665=CARTESIAN_POINT('Ctrl Pts',(16.8728578632745,46.4282028809683,72.3663567523871)) ;
#8666=CARTESIAN_POINT('Ctrl Pts',(16.7997590040171,46.6594344485583,72.2474911456601)) ;
#8667=CARTESIAN_POINT('Ctrl Pts',(16.7181710871407,46.9296827699028,72.106488131638)) ;
#8668=CARTESIAN_POINT('Ctrl Pts',(16.7064567745732,46.9687950424159,72.0860296825146)) ;
#8669=CARTESIAN_POINT('Ctrl Pts',(16.6229150124267,47.2499758749389,71.9385824666865)) ;
#8670=CARTESIAN_POINT('Ctrl Pts',(16.5546379309754,47.4918541916704,71.8097732580192)) ;
#8671=CARTESIAN_POINT('Ctrl Pts',(16.4148961706487,48.0143150857792,71.527290243484)) ;
#8672=CARTESIAN_POINT('Ctrl Pts',(16.3447756772163,48.2952954282258,71.3730820149661)) ;
#8673=CARTESIAN_POINT('Ctrl Pts',(16.2758263325691,48.5931204307081,71.2073431067649)) ;
#8674=CARTESIAN_POINT('Ctrl Pts',(16.2719090608717,48.6101204742725,71.1978741916928)) ;
#8675=CARTESIAN_POINT('Ctrl Pts',(16.2074835803316,48.8910362150329,71.0412691919266)) ;
#8676=CARTESIAN_POINT('Ctrl Pts',(16.1514139834133,49.1549226796743,70.8921635290642)) ;
#8677=CARTESIAN_POINT('Ctrl Pts',(16.0988300543287,49.4249376060053,70.7381567568313)) ;
#8678=CARTESIAN_POINT('Ctrl Pts',(16.0976904314877,49.4308011237537,70.7348116267408)) ;
#8679=CARTESIAN_POINT('Ctrl Pts',(16.0441775069865,49.7066812295575,70.5773852479501)) ;
#8680=CARTESIAN_POINT('Ctrl Pts',(15.9965787678505,49.9768666464287,70.4215354066132)) ;
#8681=CARTESIAN_POINT('Ctrl Pts',(15.9530134055317,50.2527043291671,70.2609862544005)) ;
#8682=CARTESIAN_POINT('Ctrl Pts',(15.9521693841446,50.2580605419637,70.2578681606108)) ;
#8683=CARTESIAN_POINT('Ctrl Pts',(15.9096417772101,50.5285623062336,70.1003690587478)) ;
#8684=CARTESIAN_POINT('Ctrl Pts',(15.8726896593404,50.794089282034,69.9446678031123)) ;
#8685=CARTESIAN_POINT('Ctrl Pts',(15.8384772278282,51.0767673302898,69.7777340824964)) ;
#8686=CARTESIAN_POINT('Ctrl Pts',(15.8364699928302,51.0935097128496,69.7678425985647)) ;
#8687=CARTESIAN_POINT('Ctrl Pts',(15.817692972988,51.2516332986708,69.6743810453064)) ;
#8688=CARTESIAN_POINT('Ctrl Pts',(15.8022442313088,51.3931664825854,69.5903727637932)) ;
#8689=CARTESIAN_POINT('Ctrl Pts',(15.7769449397264,51.6479675595878,69.4388316402636)) ;
#8690=CARTESIAN_POINT('Ctrl Pts',(15.7665891159126,51.7612319406874,69.3713494162665)) ;
#8691=CARTESIAN_POINT('Ctrl Pts',(15.754768741742,51.9026374456281,69.286952649771)) ;
#8692=CARTESIAN_POINT('Ctrl Pts',(15.7524687953592,51.930809108512,69.2701312609705)) ;
#8693=CARTESIAN_POINT('Ctrl Pts',(15.7276918330122,52.2417252333189,69.0844011692014)) ;
#8694=CARTESIAN_POINT('Ctrl Pts',(15.7107036256911,52.5241195492542,68.9147995558063)) ;
#8695=CARTESIAN_POINT('Ctrl Pts',(15.6899375671172,53.0381974993431,68.6055750241504)) ;
#8696=CARTESIAN_POINT('Ctrl Pts',(15.6843270313333,53.2697333986809,68.4661514431976)) ;
#8697=CARTESIAN_POINT('Ctrl Pts',(15.6820512791615,53.5522259966907,68.2958578051499)) ;
#8698=CARTESIAN_POINT('Ctrl Pts',(15.6818222797127,53.6031771340228,68.2651358129833)) ;
#8699=CARTESIAN_POINT('Ctrl Pts',(15.6815693026304,53.8742457621066,68.1016504539459)) ;
#8700=CARTESIAN_POINT('Ctrl Pts',(15.6847597300816,54.094546305059,67.9688338872412)) ;
#8701=CARTESIAN_POINT('Ctrl Pts',(15.6932080011421,54.3774106831915,67.7985459458968)) ;
#8702=CARTESIAN_POINT('Ctrl Pts',(15.6953459101383,54.4398806254195,67.7609537303392)) ;
#8703=CARTESIAN_POINT('Ctrl Pts',(15.7058225897779,54.7114321392936,67.597625057857)) ;
#8704=CARTESIAN_POINT('Ctrl Pts',(15.7169580443123,54.9205828276717,67.4719123017497)) ;
#8705=CARTESIAN_POINT('Ctrl Pts',(15.7361100705114,55.203368432956,67.3024736213794)) ;
#8706=CARTESIAN_POINT('Ctrl Pts',(15.7414913380932,55.2772338818112,67.25826442482)) ;
#8707=CARTESIAN_POINT('Ctrl Pts',(15.7626401209462,55.5485088102171,67.096135261554)) ;
#8708=CARTESIAN_POINT('Ctrl Pts',(15.7807154494597,55.7457837763595,66.9785911073384)) ;
#8709=CARTESIAN_POINT('Ctrl Pts',(15.8104451798875,56.028258890474,66.8108962000672)) ;
#8710=CARTESIAN_POINT('Ctrl Pts',(15.8199180013933,56.1134884206094,66.7603789490545)) ;
#8711=CARTESIAN_POINT('Ctrl Pts',(15.8516265286932,56.3844426291125,66.6000522177058)) ;
#8712=CARTESIAN_POINT('Ctrl Pts',(15.8757029701572,56.5701302611215,66.4907446067644)) ;
#8713=CARTESIAN_POINT('Ctrl Pts',(15.9159005740361,56.8526653482992,66.3252858477751)) ;
#8714=CARTESIAN_POINT('Ctrl Pts',(15.9303104866897,56.9494716030786,66.2687475535247)) ;
#8715=CARTESIAN_POINT('Ctrl Pts',(15.97242663624,57.2204413601181,66.1109211838358)) ;
#8716=CARTESIAN_POINT('Ctrl Pts',(16.0015712084872,57.3946576755328,66.0099460011525)) ;
#8717=CARTESIAN_POINT('Ctrl Pts',(16.052156096611,57.6774250653639,65.847114625726)) ;
#8718=CARTESIAN_POINT('Ctrl Pts',(16.0723519015129,57.7859396412651,65.7848796065074)) ;
#8719=CARTESIAN_POINT('Ctrl Pts',(16.0985692319185,57.9216227418852,65.7074259475211)) ;
#8720=CARTESIAN_POINT('Ctrl Pts',(16.1038558615345,57.9487278912594,65.6919680890366)) ;
#8721=CARTESIAN_POINT('Ctrl Pts',(16.1225472414256,58.0436810159813,65.6378716204347)) ;
#8722=CARTESIAN_POINT('Ctrl Pts',(16.1362123557029,58.1115399743054,65.5993088847567)) ;
#8723=CARTESIAN_POINT('Ctrl Pts',(16.1571689589409,58.213348452282,65.5416158561056)) ;
#8724=CARTESIAN_POINT('Ctrl Pts',(16.1642303660134,58.2472850649057,65.5224116540639)) ;
#8725=CARTESIAN_POINT('Ctrl Pts',(16.1749370090524,58.2981973836577,65.4936437723222)) ;
#8726=CARTESIAN_POINT('Ctrl Pts',(16.1785249790529,58.3151693899102,65.4840608820805)) ;
#8727=CARTESIAN_POINT('Ctrl Pts',(16.1831146844042,58.3367668565652,65.4718755710812)) ;
#8728=CARTESIAN_POINT('Ctrl Pts',(16.1841006559929,58.3413999128708,65.4692621364033)) ;
#8729=CARTESIAN_POINT('Ctrl Pts',(16.1877259353632,58.3584108602044,65.4596685309343)) ;
#8730=CARTESIAN_POINT('Ctrl Pts',(16.1903757616756,58.3707975233394,65.4526867860696)) ;
#8731=CARTESIAN_POINT('Ctrl Pts',(16.193006791085,58.3830508753327,65.4457840449521)) ;
#8732=CARTESIAN_POINT('',(-1.74213662306821,58.3831162793798,58.3447753707129)) ;
#8733=CARTESIAN_POINT('Ctrl Pts',(16.193000981218,58.3830900980199,65.4457986821614)) ;
#8734=CARTESIAN_POINT('Ctrl Pts',(13.2038113796415,58.383105259385,64.2622947965787)) ;
#8735=CARTESIAN_POINT('Ctrl Pts',(10.214621778017,58.3831073991803,63.078790910977)) ;
#8736=CARTESIAN_POINT('Ctrl Pts',(4.2362422666582,58.3831134572109,60.7117830177842)) ;
#8737=CARTESIAN_POINT('Ctrl Pts',(1.24705235690671,58.3831150235133,59.5282790101862)) ;
#8738=CARTESIAN_POINT('Ctrl Pts',(-1.7421375528447,58.3831162793802,58.3447750025884)) ;
#8739=CARTESIAN_POINT('',(-11.2681471610183,55.1047242171091,64.0109093285607)) ;
#8740=CARTESIAN_POINT('Ctrl Pts',(-1.74213662306821,58.3831162793798,58.3447753707129)) ;
#8741=CARTESIAN_POINT('Ctrl Pts',(-2.29047317474531,58.3831165097558,58.1276735718927)) ;
#8742=CARTESIAN_POINT('Ctrl Pts',(-2.86285096802688,58.3477204630489,57.9812725503403)) ;
#8743=CARTESIAN_POINT('Ctrl Pts',(-4.12531944509307,58.2097834099593,57.8223467259657)) ;
#8744=CARTESIAN_POINT('Ctrl Pts',(-4.8102892656691,58.0979492508202,57.8377999156764)) ;
#8745=CARTESIAN_POINT('Ctrl Pts',(-6.37924732927157,57.7707079403455,58.1010309533822)) ;
#8746=CARTESIAN_POINT('Ctrl Pts',(-7.23417879357875,57.5360203747158,58.426251502882)) ;
#8747=CARTESIAN_POINT('Ctrl Pts',(-8.82516552869592,56.9856760363639,59.4087857781323)) ;
#8748=CARTESIAN_POINT('Ctrl Pts',(-9.53107642063704,56.668734645817,60.0831182465607)) ;
#8749=CARTESIAN_POINT('Ctrl Pts',(-10.4108790833113,56.1294194252976,61.3553806219125)) ;
#8750=CARTESIAN_POINT('Ctrl Pts',(-10.6821762328728,55.9194277706208,61.8779177589046)) ;
#8751=CARTESIAN_POINT('Ctrl Pts',(-11.0740895432526,55.5068627643851,62.9384006699818)) ;
#8752=CARTESIAN_POINT('Ctrl Pts',(-11.2025958471988,55.3059552090325,63.4700991792931)) ;
#8753=CARTESIAN_POINT('Ctrl Pts',(-11.2681471610183,55.104724217109,64.0109093285607)) ;
#8754=CARTESIAN_POINT('',(-9.03444461093391,48.6398835186857,81.1828053420911)) ;
#8755=CARTESIAN_POINT('Ctrl Pts',(-9.03444461093391,48.6398835186857,81.1828053420911)) ;
#8756=CARTESIAN_POINT('Ctrl Pts',(-9.19872655925457,48.8038201453524,80.7706908861205)) ;
#8757=CARTESIAN_POINT('Ctrl Pts',(-9.35250971390351,48.9676174488035,80.3545447282502)) ;
#8758=CARTESIAN_POINT('Ctrl Pts',(-9.91341105588012,49.5650439193917,78.8367130844612)) ;
#8759=CARTESIAN_POINT('Ctrl Pts',(-10.3318718559021,50.16247038998,77.2736027962334)) ;
#8760=CARTESIAN_POINT('Ctrl Pts',(-10.750332655924,50.7598968605682,75.7104925080056)) ;
#8761=CARTESIAN_POINT('Ctrl Pts',(-11.0227827539907,51.3573233311564,74.1154394811811)) ;
#8762=CARTESIAN_POINT('Ctrl Pts',(-11.2952328520573,51.9547498017447,72.5203864543566)) ;
#8763=CARTESIAN_POINT('Ctrl Pts',(-11.4193477999951,52.5521762723329,70.9069991189604)) ;
#8764=CARTESIAN_POINT('Ctrl Pts',(-11.5434627479329,53.1496027429211,69.2936117835642)) ;
#8765=CARTESIAN_POINT('Ctrl Pts',(-11.5181836407678,53.7470292135094,67.6756549914775)) ;
#8766=CARTESIAN_POINT('Ctrl Pts',(-11.4929045336027,54.3444556840976,66.0576981993908)) ;
#8767=CARTESIAN_POINT('Ctrl Pts',(-11.3184470437638,54.9418821546858,64.4489757874882)) ;
#8768=CARTESIAN_POINT('Ctrl Pts',(-11.2946768606995,55.0232827101246,64.2297841307363)) ;
#8769=CARTESIAN_POINT('Ctrl Pts',(-11.2681471610183,55.1047242171091,64.0109093285607)) ;
#8770=CARTESIAN_POINT('Ctrl Pts',(-9.03444461093392,48.6398835186858,81.1828053420911)) ;
#8771=CARTESIAN_POINT('Ctrl Pts',(-8.83397598669229,48.4398362807108,81.6856969796876)) ;
#8772=CARTESIAN_POINT('Ctrl Pts',(-8.57568233556347,48.2402512214434,82.1640409953046)) ;
#8773=CARTESIAN_POINT('Ctrl Pts',(-7.93146167760747,47.8311034847343,83.0832927130734)) ;
#8774=CARTESIAN_POINT('Ctrl Pts',(-7.53982375225014,47.6231197022401,83.5164066873636)) ;
#8775=CARTESIAN_POINT('Ctrl Pts',(-6.37128043545755,47.08626813226,84.5219283426251)) ;
#8776=CARTESIAN_POINT('Ctrl Pts',(-5.51827317218396,46.770327077101,84.9961775434417)) ;
#8777=CARTESIAN_POINT('Ctrl Pts',(-3.73052572361336,46.2216257312613,85.5454708941863)) ;
#8778=CARTESIAN_POINT('Ctrl Pts',(-2.82130999507985,45.9879058539332,85.6443247921444)) ;
#8779=CARTESIAN_POINT('Ctrl Pts',(-1.24213321159846,45.6640068779433,85.5034836180374)) ;
#8780=CARTESIAN_POINT('Ctrl Pts',(-0.580849897547363,45.5539383973837,85.347630943253)) ;
#8781=CARTESIAN_POINT('Ctrl Pts',(0.593309673962527,45.4179657782124,84.8813839044439)) ;
#8782=CARTESIAN_POINT('Ctrl Pts',(1.10809034600835,45.3830586252741,84.5985045791954)) ;
#8783=CARTESIAN_POINT('Ctrl Pts',(1.58245214009828,45.3830586252741,84.2538605621281)) ;
#8784=CARTESIAN_POINT('Origin',(-2.53204462594907,45.3822493559848,78.5907416015035)) ;
#8785=CARTESIAN_POINT('',(-9.03444461093391,45.3822493559848,81.1828053420911)) ;
#8786=CARTESIAN_POINT('Origin',(23.4776880157599,45.3822493559848,68.2224337400009)) ;
#8787=CARTESIAN_POINT('',(-11.2681471610183,45.3822493559848,64.0109093285607)) ;
#8788=CARTESIAN_POINT('Origin',(-4.31900848943611,45.3822493559848,64.8532107728907)) ;
#8789=CARTESIAN_POINT('',(-1.74213662306825,45.3822493559848,58.3447753707129)) ;
#8790=CARTESIAN_POINT('Origin',(16.4675440301639,45.3822493559848,65.5544979647415)) ;
#8791=CARTESIAN_POINT('Ctrl Pts',(16.3751780994845,57.8271591849708,65.5179277057667)) ;
#8792=CARTESIAN_POINT('Ctrl Pts',(16.375098264844,57.8726765548514,65.5178960969965)) ;
#8793=CARTESIAN_POINT('Ctrl Pts',(16.3712357710984,57.9189555946976,65.5163668275686)) ;
#8794=CARTESIAN_POINT('Ctrl Pts',(16.3555004313488,58.0070760904206,65.5101367658406)) ;
#8795=CARTESIAN_POINT('Ctrl Pts',(16.343438841416,58.0511720072647,65.5053612445326)) ;
#8796=CARTESIAN_POINT('Ctrl Pts',(16.3098321161203,58.1280396089059,65.4920554007185)) ;
#8797=CARTESIAN_POINT('Ctrl Pts',(16.2904201996508,58.1581206861651,65.4843696792975)) ;
#8798=CARTESIAN_POINT('Ctrl Pts',(16.257133458184,58.1912258391351,65.4711905260435)) ;
#8799=CARTESIAN_POINT('Ctrl Pts',(16.2440370654752,58.2011509268498,65.4660052973562)) ;
#8800=CARTESIAN_POINT('Ctrl Pts',(16.2172691776374,58.2136664809846,65.4554071408364)) ;
#8801=CARTESIAN_POINT('Ctrl Pts',(16.2043402194456,58.2169696033444,65.4502882041693)) ;
#8802=CARTESIAN_POINT('Ctrl Pts',(16.1909560759401,58.2172758076352,65.4449890468874)) ;
#8803=CARTESIAN_POINT('Ctrl Pts',(16.1930011817604,58.3830247512578,65.4457987615618)) ;
#8804=CARTESIAN_POINT('Ctrl Pts',(16.1995379570469,58.3830247228401,65.4483868539821)) ;
#8805=CARTESIAN_POINT('Ctrl Pts',(16.2060215176076,58.3837424765203,65.450953877202)) ;
#8806=CARTESIAN_POINT('Ctrl Pts',(16.219260687547,58.3866521091205,65.4561956353886)) ;
#8807=CARTESIAN_POINT('Ctrl Pts',(16.2259025352896,58.3889169429325,65.4588253289371)) ;
#8808=CARTESIAN_POINT('Ctrl Pts',(16.2470604727698,58.3985444430827,65.4672023489848)) ;
#8809=CARTESIAN_POINT('Ctrl Pts',(16.2603412472946,58.408561171848,65.4724605795664)) ;
#8810=CARTESIAN_POINT('Ctrl Pts',(16.2929811784212,58.4411881106263,65.4853836424906)) ;
#8811=CARTESIAN_POINT('Ctrl Pts',(16.3116752992976,58.4701790970316,65.492785168563)) ;
#8812=CARTESIAN_POINT('Ctrl Pts',(16.344401615182,58.5450328515258,65.5057424336322)) ;
#8813=CARTESIAN_POINT('Ctrl Pts',(16.3561655785037,58.5884055134699,65.5104001161195)) ;
#8814=CARTESIAN_POINT('Ctrl Pts',(16.3714864465992,58.6752768777081,65.516466076911)) ;
#8815=CARTESIAN_POINT('Ctrl Pts',(16.3751788432793,58.7210404158283,65.5179280002559)) ;
#8816=CARTESIAN_POINT('Ctrl Pts',(16.3751784807748,58.7660404020406,65.5179278567302)) ;
#8817=CARTESIAN_POINT('Ctrl Pts',(16.2076436667534,58.2943663992286,65.4015964591232)) ;
#8818=CARTESIAN_POINT('Ctrl Pts',(16.3901988775676,58.2924602039142,65.4736624527373)) ;
#8819=CARTESIAN_POINT('Ctrl Pts',(16.4544192595841,58.191081348463,65.3183511002461)) ;
#8820=CARTESIAN_POINT('Ctrl Pts',(16.0893935021919,57.752299968197,65.7063617193311)) ;
#8821=CARTESIAN_POINT('Ctrl Pts',(16.2749670678282,57.7503889244133,65.7707754261454)) ;
#8822=CARTESIAN_POINT('Ctrl Pts',(16.3326721110413,57.6489874075171,65.6127858841635)) ;
#8823=CARTESIAN_POINT('Ctrl Pts',(15.9905079233388,57.2111033102693,66.0180958060857)) ;
#8824=CARTESIAN_POINT('Ctrl Pts',(16.1786178839759,57.2091968025795,66.0746770851081)) ;
#8825=CARTESIAN_POINT('Ctrl Pts',(16.2296654835751,57.1078632091335,65.9143707409572)) ;
#8826=CARTESIAN_POINT('Ctrl Pts',(15.8720965683249,56.3997926693407,66.4926301853558)) ;
#8827=CARTESIAN_POINT('Ctrl Pts',(16.0632571274154,56.3978864499462,66.5372862974148)) ;
#8828=CARTESIAN_POINT('Ctrl Pts',(16.1041311822517,56.296529089974,66.3742167663536)) ;
#8829=CARTESIAN_POINT('Ctrl Pts',(15.8375699261364,56.1295297083804,66.6521222695944)) ;
#8830=CARTESIAN_POINT('Ctrl Pts',(16.029624201713,56.1276240321266,66.6927701563547)) ;
#8831=CARTESIAN_POINT('Ctrl Pts',(16.0670707738748,56.0262125668428,66.528911362414)) ;
#8832=CARTESIAN_POINT('Ctrl Pts',(15.7785876369184,55.5885108130466,66.9729859773628)) ;
#8833=CARTESIAN_POINT('Ctrl Pts',(15.9721719553117,55.5866055506255,67.0055653548671)) ;
#8834=CARTESIAN_POINT('Ctrl Pts',(16.0027427182606,55.485272016298,66.8402402844729)) ;
#8835=CARTESIAN_POINT('Ctrl Pts',(15.754136645686,55.317901160646,67.1342772225888)) ;
#8836=CARTESIAN_POINT('Ctrl Pts',(15.9483601423746,55.3159940909051,67.162802173736)) ;
#8837=CARTESIAN_POINT('Ctrl Pts',(15.9754645077105,55.2146518759505,66.9968784550975)) ;
#8838=CARTESIAN_POINT('Ctrl Pts',(15.7153500800329,54.7764805321647,67.4585848660779)) ;
#8839=CARTESIAN_POINT('Ctrl Pts',(15.9106003761165,54.7745728258726,67.4789559682221)) ;
#8840=CARTESIAN_POINT('Ctrl Pts',(15.9307246503761,54.6731104541281,67.3121111144227)) ;
#8841=CARTESIAN_POINT('Ctrl Pts',(15.7010384513997,54.5052712784467,67.6215916940795)) ;
#8842=CARTESIAN_POINT('Ctrl Pts',(15.896670066885,54.5033650628029,67.6378592813634)) ;
#8843=CARTESIAN_POINT('Ctrl Pts',(15.9132990653192,54.4020271817646,67.4705583238743)) ;
#8844=CARTESIAN_POINT('Ctrl Pts',(15.6827101205307,53.9638812711069,67.9474523132968)) ;
#8845=CARTESIAN_POINT('Ctrl Pts',(15.8788516918128,53.9619749130852,67.9555219668616)) ;
#8846=CARTESIAN_POINT('Ctrl Pts',(15.8884659090552,53.8606102461995,67.7876870896055)) ;
#8847=CARTESIAN_POINT('Ctrl Pts',(15.6786640134442,53.69350032242,68.1106760287787)) ;
#8848=CARTESIAN_POINT('Ctrl Pts',(15.8749323601421,53.691594608915,68.1146384349466)) ;
#8849=CARTESIAN_POINT('Ctrl Pts',(15.8810307763445,53.5901950776882,67.9466591165899)) ;
#8850=CARTESIAN_POINT('Ctrl Pts',(15.6808110138424,53.1525885953391,68.4368174081503)) ;
#8851=CARTESIAN_POINT('Ctrl Pts',(15.8770716769607,53.1506832357684,68.4325700314882)) ;
#8852=CARTESIAN_POINT('Ctrl Pts',(15.8761429126677,53.0493503316298,68.2644444735657)) ;
#8853=CARTESIAN_POINT('Ctrl Pts',(15.6869930500739,52.8821999703205,68.5997058627992)) ;
#8854=CARTESIAN_POINT('Ctrl Pts',(15.8831225594926,52.8802927777111,68.5913594125356)) ;
#8855=CARTESIAN_POINT('Ctrl Pts',(15.8786793848031,52.7789455602561,68.4232981395322)) ;
#8856=CARTESIAN_POINT('Ctrl Pts',(15.7095785926957,52.3415574725993,68.9251182619377)) ;
#8857=CARTESIAN_POINT('Ctrl Pts',(15.9051911925639,52.3396495857393,68.9085807093587)) ;
#8858=CARTESIAN_POINT('Ctrl Pts',(15.8937284189081,52.2381712237815,68.7409272439851)) ;
#8859=CARTESIAN_POINT('Ctrl Pts',(15.7259867557631,52.070892318345,69.087548400577)) ;
#8860=CARTESIAN_POINT('Ctrl Pts',(15.9212064002032,52.0689860211472,69.0669176150257)) ;
#8861=CARTESIAN_POINT('Ctrl Pts',(15.9062323156006,51.9676510264301,68.899458753588)) ;
#8862=CARTESIAN_POINT('Ctrl Pts',(15.7689707763681,51.5294526417263,69.4111229964008)) ;
#8863=CARTESIAN_POINT('Ctrl Pts',(15.9631573413053,51.5275461441184,69.382342803655)) ;
#8864=CARTESIAN_POINT('Ctrl Pts',(15.9411922096572,51.4261734609838,69.2156785502537)) ;
#8865=CARTESIAN_POINT('Ctrl Pts',(15.7956084260211,51.2584285629724,69.5726116865006)) ;
#8866=CARTESIAN_POINT('Ctrl Pts',(15.9891487491342,51.2565228090376,69.5397629590593)) ;
#8867=CARTESIAN_POINT('Ctrl Pts',(15.9636931377913,51.1551340723535,69.3736053139055)) ;
#8868=CARTESIAN_POINT('Ctrl Pts',(15.8588547216987,50.7168256229871,69.8929710826407)) ;
#8869=CARTESIAN_POINT('Ctrl Pts',(16.0508488942934,50.714920164228,69.8520495815658)) ;
#8870=CARTESIAN_POINT('Ctrl Pts',(16.0184554339797,50.6135869790189,69.6870716848916)) ;
#8871=CARTESIAN_POINT('Ctrl Pts',(15.8954576104322,50.4462620313559,70.0519295278353)) ;
#8872=CARTESIAN_POINT('Ctrl Pts',(16.086554844969,50.4443547062442,70.0070033433742)) ;
#8873=CARTESIAN_POINT('Ctrl Pts',(16.0507194340179,50.3430015532915,69.8427504295619)) ;
#8874=CARTESIAN_POINT('Ctrl Pts',(15.9785962095983,49.9056099882918,70.3674102992357)) ;
#8875=CARTESIAN_POINT('Ctrl Pts',(16.1676517617608,49.9037019096486,70.3145334544655)) ;
#8876=CARTESIAN_POINT('Ctrl Pts',(16.1249977677534,49.8022062837278,70.1520022424188)) ;
#8877=CARTESIAN_POINT('Ctrl Pts',(16.0251026927125,49.6350408217638,70.5237830491593)) ;
#8878=CARTESIAN_POINT('Ctrl Pts',(16.2130058621674,49.6331344367341,70.4669615662931)) ;
#8879=CARTESIAN_POINT('Ctrl Pts',(16.166938943436,49.5318014383334,70.3052677497731)) ;
#8880=CARTESIAN_POINT('Ctrl Pts',(16.1277963191435,49.0942250306986,70.8332456487283)) ;
#8881=CARTESIAN_POINT('Ctrl Pts',(16.3131619984201,49.0923183862286,70.7686210208621)) ;
#8882=CARTESIAN_POINT('Ctrl Pts',(16.2603856795457,48.9909365753751,70.6090205283714)) ;
#8883=CARTESIAN_POINT('Ctrl Pts',(16.1840618356866,48.8238179925398,70.9865468887572)) ;
#8884=CARTESIAN_POINT('Ctrl Pts',(16.3680337664969,48.8219121926559,70.9180551942438)) ;
#8885=CARTESIAN_POINT('Ctrl Pts',(16.3119277610878,48.7205331729598,70.7595928038727)) ;
#8886=CARTESIAN_POINT('Ctrl Pts',(16.3060990374279,48.2823982253115,71.2892898858962)) ;
#8887=CARTESIAN_POINT('Ctrl Pts',(16.4870428135359,48.2804926625057,71.2131605180457)) ;
#8888=CARTESIAN_POINT('Ctrl Pts',(16.4243469194233,48.1791582421864,71.0571604502067)) ;
#8889=CARTESIAN_POINT('Ctrl Pts',(16.37190690666,48.0114576298554,71.4388408381481)) ;
#8890=CARTESIAN_POINT('Ctrl Pts',(16.5512210931819,48.0095520695984,71.3589384370468)) ;
#8891=CARTESIAN_POINT('Ctrl Pts',(16.4853051187392,47.908060964341,71.204368923494)) ;
#8892=CARTESIAN_POINT('Ctrl Pts',(16.5129038822507,47.4697670852096,71.7337231132686)) ;
#8893=CARTESIAN_POINT('Ctrl Pts',(16.6887086670034,47.4678622559189,71.6463775616732)) ;
#8894=CARTESIAN_POINT('Ctrl Pts',(16.6163421825885,47.3665093096576,71.4946332104983)) ;
#8895=CARTESIAN_POINT('Ctrl Pts',(16.5878839183077,47.1991192501698,71.8786404936035)) ;
#8896=CARTESIAN_POINT('Ctrl Pts',(16.7618228296394,47.1972127705445,71.7876375575991)) ;
#8897=CARTESIAN_POINT('Ctrl Pts',(16.6862917823392,47.0958808569866,71.6374299430126)) ;
#8898=CARTESIAN_POINT('Ctrl Pts',(16.7467474591064,46.6582159321204,72.1634615282512)) ;
#8899=CARTESIAN_POINT('Ctrl Pts',(16.9167319946848,46.6563091332048,72.0652670932486)) ;
#8900=CARTESIAN_POINT('Ctrl Pts',(16.8350038471522,46.5549171221787,71.9183786668138)) ;
#8901=CARTESIAN_POINT('Ctrl Pts',(16.8307007910212,46.3878930438422,72.3034640403305)) ;
#8902=CARTESIAN_POINT('Ctrl Pts',(16.9985920820615,46.3859871917183,72.2017331629075)) ;
#8903=CARTESIAN_POINT('Ctrl Pts',(16.9138021385845,46.2846172014626,72.056576034241)) ;
#8904=CARTESIAN_POINT('Ctrl Pts',(17.0070827839767,45.8470089936314,72.5777188611197)) ;
#8905=CARTESIAN_POINT('Ctrl Pts',(17.1705743029419,45.8451033189024,72.4690595698271)) ;
#8906=CARTESIAN_POINT('Ctrl Pts',(17.0797814323178,45.7437666877221,72.3275569160594)) ;
#8907=CARTESIAN_POINT('Ctrl Pts',(17.0995563707454,45.5765948766489,72.7120629137262)) ;
#8908=CARTESIAN_POINT('Ctrl Pts',(17.2607441051786,45.5746876691147,72.6000093665917)) ;
#8909=CARTESIAN_POINT('Ctrl Pts',(17.1670266235441,45.4732994149914,72.4604609422583)) ;
#8910=CARTESIAN_POINT('Ctrl Pts',(17.1962999806241,45.3060601767044,72.8435636952195)) ;
#8911=CARTESIAN_POINT('Ctrl Pts',(17.3550714514673,45.3041537286489,72.7281859629674)) ;
#8912=CARTESIAN_POINT('Ctrl Pts',(17.2584885598876,45.2027271666488,72.5906780243875)) ;
#8913=CARTESIAN_POINT('Ctrl Pts',(17.2968875596656,45.1993067880442,72.973657143502)) ;
#8914=CARTESIAN_POINT('Ctrl Pts',(17.451249335316,45.2022951414426,72.855866322441)) ;
#8915=CARTESIAN_POINT('Ctrl Pts',(17.5553932904832,45.3026470834629,72.9854606506312)) ;
#8916=CARTESIAN_POINT('Ctrl Pts',(17.1929325562347,45.4820412744203,72.8384255376541)) ;
#8917=CARTESIAN_POINT('Ctrl Pts',(17.3498724730783,45.4850280413069,72.7240107837351)) ;
#8918=CARTESIAN_POINT('Ctrl Pts',(17.4511824806264,45.5853775943584,72.8558860880284)) ;
#8919=CARTESIAN_POINT('Ctrl Pts',(17.0936474486457,45.7643410734892,72.7000748128061)) ;
#8920=CARTESIAN_POINT('Ctrl Pts',(17.2530462868952,45.7673284499132,72.5891193657422)) ;
#8921=CARTESIAN_POINT('Ctrl Pts',(17.3514803736145,45.8675945653398,72.7232114728561)) ;
#8922=CARTESIAN_POINT('Ctrl Pts',(16.9046842952674,46.328018306681,72.4177729528116)) ;
#8923=CARTESIAN_POINT('Ctrl Pts',(17.0687646573102,46.331005889118,72.3138645852439)) ;
#8924=CARTESIAN_POINT('Ctrl Pts',(17.1612596670856,46.4312885658147,72.4521090456578)) ;
#8925=CARTESIAN_POINT('Ctrl Pts',(16.8148839283541,46.6093355962119,72.2736303591509)) ;
#8926=CARTESIAN_POINT('Ctrl Pts',(16.9811890146995,46.6123226913613,72.1733185766999)) ;
#8927=CARTESIAN_POINT('Ctrl Pts',(17.070637445787,46.7126511405725,72.3135226725028)) ;
#8928=CARTESIAN_POINT('Ctrl Pts',(16.6450769382365,47.1717937445032,71.9801663667652)) ;
#8929=CARTESIAN_POINT('Ctrl Pts',(16.8155843847405,47.1747799487467,71.8871818339373)) ;
#8930=CARTESIAN_POINT('Ctrl Pts',(16.898874585859,47.2750367263762,72.0311762509218)) ;
#8931=CARTESIAN_POINT('Ctrl Pts',(16.5650865575195,47.4527838882157,71.8308984330576)) ;
#8932=CARTESIAN_POINT('Ctrl Pts',(16.7375724992622,47.4557728130825,71.7416366037205)) ;
#8933=CARTESIAN_POINT('Ctrl Pts',(16.8177106448256,47.5560442950795,71.8873993380807)) ;
#8934=CARTESIAN_POINT('Ctrl Pts',(16.4149022782682,48.0142871287587,71.5273059776434)) ;
#8935=CARTESIAN_POINT('Ctrl Pts',(16.5911042040292,48.0172777959156,71.4456128616253)) ;
#8936=CARTESIAN_POINT('Ctrl Pts',(16.6648000440323,48.1176897428506,71.5946479830374)) ;
#8937=CARTESIAN_POINT('Ctrl Pts',(16.3447812976334,48.2952668190988,71.3730983517084)) ;
#8938=CARTESIAN_POINT('Ctrl Pts',(16.5227137172553,48.2982544973843,71.2952593298538)) ;
#8939=CARTESIAN_POINT('Ctrl Pts',(16.5931940987698,48.3985111247922,71.4459383708063)) ;
#8940=CARTESIAN_POINT('Ctrl Pts',(16.214741633037,48.8569739450496,71.0605092697478)) ;
#8941=CARTESIAN_POINT('Ctrl Pts',(16.3958861388272,48.8599622667949,70.9904650444409)) ;
#8942=CARTESIAN_POINT('Ctrl Pts',(16.4597477106443,48.9602706397639,71.1440347517157)) ;
#8943=CARTESIAN_POINT('Ctrl Pts',(16.1547372811686,49.1378578224163,70.9018967081238)) ;
#8944=CARTESIAN_POINT('Ctrl Pts',(16.3373622620764,49.1408449473386,70.8358093418605)) ;
#8945=CARTESIAN_POINT('Ctrl Pts',(16.3978721266104,49.2411421341037,70.9907371606981)) ;
#8946=CARTESIAN_POINT('Ctrl Pts',(16.045206308162,49.7002903801079,70.5811055636178)) ;
#8947=CARTESIAN_POINT('Ctrl Pts',(16.2305301078175,49.7032770483596,70.523019074802)) ;
#8948=CARTESIAN_POINT('Ctrl Pts',(16.284256690246,49.8035375139106,70.6804497323144)) ;
#8949=CARTESIAN_POINT('Ctrl Pts',(15.9956378175181,49.9815741041282,70.4188518451987)) ;
#8950=CARTESIAN_POINT('Ctrl Pts',(16.1821849956454,49.9845613531715,70.3648063422433)) ;
#8951=CARTESIAN_POINT('Ctrl Pts',(16.2324502058595,50.0849543128215,70.5232979085427)) ;
#8952=CARTESIAN_POINT('Ctrl Pts',(15.9070166158438,50.5452598054762,70.090646978502)) ;
#8953=CARTESIAN_POINT('Ctrl Pts',(16.0957390532765,50.5482454986069,70.044788576911)) ;
#8954=CARTESIAN_POINT('Ctrl Pts',(16.1390683728253,50.6485130930204,70.2053882479554)) ;
#8955=CARTESIAN_POINT('Ctrl Pts',(15.8680534537747,50.8275371605423,69.9250501649938)) ;
#8956=CARTESIAN_POINT('Ctrl Pts',(16.0577309660869,50.8305252760806,69.8833184453582)) ;
#8957=CARTESIAN_POINT('Ctrl Pts',(16.0975469811511,50.9307809743298,70.0448322276628)) ;
#8958=CARTESIAN_POINT('Ctrl Pts',(15.817695468004,51.2516112326466,69.6743941084036)) ;
#8959=CARTESIAN_POINT('Ctrl Pts',(16.0086068770328,51.2545993841867,69.6389077620491)) ;
#8960=CARTESIAN_POINT('Ctrl Pts',(16.0430917908323,51.3549223743145,69.8015738795152)) ;
#8961=CARTESIAN_POINT('Ctrl Pts',(15.8022455195989,51.3931523912035,69.5903811628836)) ;
#8962=CARTESIAN_POINT('Ctrl Pts',(15.9935348337152,51.3961401671646,69.5569883942883)) ;
#8963=CARTESIAN_POINT('Ctrl Pts',(16.0262336376549,51.4964802131712,69.7200131309892)) ;
#8964=CARTESIAN_POINT('Ctrl Pts',(15.7741453113461,51.6761627264733,69.422062782985)) ;
#8965=CARTESIAN_POINT('Ctrl Pts',(15.9661181557686,51.6791498413111,69.3928666277847)) ;
#8966=CARTESIAN_POINT('Ctrl Pts',(15.9952469927814,51.7794366542442,69.556597417726)) ;
#8967=CARTESIAN_POINT('Ctrl Pts',(15.761490146833,51.8176028378204,69.3377566191795)) ;
#8968=CARTESIAN_POINT('Ctrl Pts',(15.9537703088477,51.8205901090039,69.3106616104865)) ;
#8969=CARTESIAN_POINT('Ctrl Pts',(15.9811083432102,51.9208634696797,69.4747085828085)) ;
#8970=CARTESIAN_POINT('Ctrl Pts',(15.727691356137,52.2417288193164,69.0843990475119)) ;
#8971=CARTESIAN_POINT('Ctrl Pts',(15.9207908993607,52.244716110021,69.0636171801009)) ;
#8972=CARTESIAN_POINT('Ctrl Pts',(15.9427411584188,52.3449902631942,69.2285011527611)) ;
#8973=CARTESIAN_POINT('Ctrl Pts',(15.7107023087123,52.5241300049526,68.9147933424545)) ;
#8974=CARTESIAN_POINT('Ctrl Pts',(15.9042121206607,52.5271171122649,68.8982355118463)) ;
#8975=CARTESIAN_POINT('Ctrl Pts',(15.9225483779282,52.6274614458918,69.0635205182557)) ;
#8976=CARTESIAN_POINT('Ctrl Pts',(15.6878767651245,53.0891744812518,68.5749117700964)) ;
#8977=CARTESIAN_POINT('Ctrl Pts',(15.881922329841,53.0921605107966,68.5668240512164)) ;
#8978=CARTESIAN_POINT('Ctrl Pts',(15.8930266987946,53.1924181127708,68.7328008850591)) ;
#8979=CARTESIAN_POINT('Ctrl Pts',(15.6820372968995,53.3716654702733,68.4047638003974)) ;
#8980=CARTESIAN_POINT('Ctrl Pts',(15.8762134290656,53.3746541735213,68.4009124350081)) ;
#8981=CARTESIAN_POINT('Ctrl Pts',(15.8836899306515,53.4749194098514,68.5670880136959)) ;
#8982=CARTESIAN_POINT('Ctrl Pts',(15.6815112504157,53.9365848433274,68.0640528555997)) ;
#8983=CARTESIAN_POINT('Ctrl Pts',(15.8756745974021,53.939575131127,68.0686834602829)) ;
#8984=CARTESIAN_POINT('Ctrl Pts',(15.8758831838286,54.0399680491534,68.2349550032619)) ;
#8985=CARTESIAN_POINT('Ctrl Pts',(15.6868397059094,54.2194050938135,67.8935619946214)) ;
#8986=CARTESIAN_POINT('Ctrl Pts',(15.88085072629,54.2223926611942,67.9024431647425)) ;
#8987=CARTESIAN_POINT('Ctrl Pts',(15.8774231007484,54.3226514036281,68.0687552371563)) ;
#8988=CARTESIAN_POINT('Ctrl Pts',(15.7086729983829,54.7853172886158,67.553185729259)) ;
#8989=CARTESIAN_POINT('Ctrl Pts',(15.9021114891387,54.7883053531188,67.5705413052623)) ;
#8990=CARTESIAN_POINT('Ctrl Pts',(15.8914153126205,54.8886040661601,67.736521881602)) ;
#8991=CARTESIAN_POINT('Ctrl Pts',(15.7252052959611,55.0683374452749,67.3831126794745)) ;
#8992=CARTESIAN_POINT('Ctrl Pts',(15.9182171697501,55.0713245454019,67.404703163084)) ;
#8993=CARTESIAN_POINT('Ctrl Pts',(15.9038874382428,55.1716304682316,67.5704054125967)) ;
#8994=CARTESIAN_POINT('Ctrl Pts',(15.769289072919,55.6338317485951,67.0451410222993)) ;
#8995=CARTESIAN_POINT('Ctrl Pts',(15.9611713077456,55.6368182566034,67.0751464795178)) ;
#8996=CARTESIAN_POINT('Ctrl Pts',(15.9396114207564,55.7370765662141,67.240090940531)) ;
#8997=CARTESIAN_POINT('Ctrl Pts',(15.7968305063234,55.9162154787387,66.8771073253589)) ;
#8998=CARTESIAN_POINT('Ctrl Pts',(15.9880173845642,55.9192027777541,66.9112923600459)) ;
#8999=CARTESIAN_POINT('Ctrl Pts',(15.9628724013359,56.0196099645353,67.0756434800854)) ;
#9000=CARTESIAN_POINT('Ctrl Pts',(15.8629517303589,56.481225490452,66.542784474632)) ;
#9001=CARTESIAN_POINT('Ctrl Pts',(16.0524570183557,56.4842111077296,66.585293753671)) ;
#9002=CARTESIAN_POINT('Ctrl Pts',(16.0201417374786,56.5844827370484,66.7484645657872)) ;
#9003=CARTESIAN_POINT('Ctrl Pts',(15.9014426423274,56.7637439358746,66.3769244785956)) ;
#9004=CARTESIAN_POINT('Ctrl Pts',(16.0899742906582,56.7667319249263,66.4235600545759)) ;
#9005=CARTESIAN_POINT('Ctrl Pts',(16.0541008627812,56.8669869420473,66.5859953376069)) ;
#9006=CARTESIAN_POINT('Ctrl Pts',(15.9892699006111,57.3288079962382,66.0478030471487)) ;
#9007=CARTESIAN_POINT('Ctrl Pts',(16.1755881248362,57.3317969661861,66.1026263528049)) ;
#9008=CARTESIAN_POINT('Ctrl Pts',(16.1326652899509,57.4321309086594,66.2632966799852)) ;
#9009=CARTESIAN_POINT('Ctrl Pts',(16.0386461895469,57.6115036703746,65.8844549210715)) ;
#9010=CARTESIAN_POINT('Ctrl Pts',(16.2237177401031,57.6144908954445,65.9433440431311)) ;
#9011=CARTESIAN_POINT('Ctrl Pts',(16.1772817370448,57.7147692588153,66.1030671471929)) ;
#9012=CARTESIAN_POINT('Ctrl Pts',(16.1480173189084,58.1775332619219,65.5613413260415)) ;
#9013=CARTESIAN_POINT('Ctrl Pts',(16.3303358670001,58.1805203783525,65.6282684666599)) ;
#9014=CARTESIAN_POINT('Ctrl Pts',(16.2769572424907,58.2807900093283,65.7858125302268)) ;
#9015=CARTESIAN_POINT('Ctrl Pts',(16.2080701484261,58.4605262973704,65.4014232574249)) ;
#9016=CARTESIAN_POINT('Ctrl Pts',(16.3888822517855,58.4635120170919,65.4723277868928)) ;
#9017=CARTESIAN_POINT('Ctrl Pts',(16.3320875218486,58.5638924134504,65.6286060519377)) ;
#9018=CARTESIAN_POINT('Ctrl Pts',(16.2731529226733,58.7433256931628,65.2440040205795)) ;
#9019=CARTESIAN_POINT('Ctrl Pts',(16.4523242289707,58.7463128973535,65.3188245830744)) ;
#9020=CARTESIAN_POINT('Ctrl Pts',(16.3921137230323,58.846547398596,65.4738637287654)) ;
#9021=CARTESIAN_POINT('Origin',(34.3408356446983,45.3830586252741,101.493960960612)) ;
#9022=CARTESIAN_POINT('',(25.8874434877188,45.3830610445957,75.638885508351)) ;
#9023=CARTESIAN_POINT('',(32.2277009906555,45.3830586252741,95.1522046229055)) ;
#9024=CARTESIAN_POINT('',(25.8874396740751,45.3830586252741,75.6388867474779)) ;
#9025=CARTESIAN_POINT('Ctrl Pts',(25.8874448759437,45.3830586252741,75.6388850572898)) ;
#9026=CARTESIAN_POINT('Ctrl Pts',(25.8831721961058,45.3830586252741,75.6257350973774)) ;
#9027=CARTESIAN_POINT('Ctrl Pts',(25.877335045612,45.3830586252741,75.6131877264577)) ;
#9028=CARTESIAN_POINT('Ctrl Pts',(25.8622162570581,45.3830586252741,75.5887217865201)) ;
#9029=CARTESIAN_POINT('Ctrl Pts',(25.8527987231294,45.3830586252741,75.5770968153146)) ;
#9030=CARTESIAN_POINT('Ctrl Pts',(25.8226143339006,45.3830586252741,75.5477565599384)) ;
#9031=CARTESIAN_POINT('Ctrl Pts',(25.799308805845,45.3830586252741,75.5332471960665)) ;
#9032=CARTESIAN_POINT('Ctrl Pts',(25.7465957636447,45.3830586252741,75.5124525882851)) ;
#9033=CARTESIAN_POINT('Ctrl Pts',(25.7172005505345,45.3830586252736,75.5070624718622)) ;
#9034=CARTESIAN_POINT('Ctrl Pts',(25.6610381928182,45.3830586252736,75.5063308717296)) ;
#9035=CARTESIAN_POINT('Ctrl Pts',(25.634330653479,45.3830586252741,75.5100675780367)) ;
#9036=CARTESIAN_POINT('Ctrl Pts',(25.6087276455907,45.3830586252741,75.5175467475628)) ;
#9037=CARTESIAN_POINT('',(25.9816821278123,45.3830674541116,75.6052810522977)) ;
#9038=CARTESIAN_POINT('Ctrl Pts',(26.1331741609198,45.3830586252741,75.3434163707841)) ;
#9039=CARTESIAN_POINT('Ctrl Pts',(26.108588619251,45.3830586252741,75.3525850395932)) ;
#9040=CARTESIAN_POINT('Ctrl Pts',(26.0853132912683,45.3830586252745,75.3652945006832)) ;
#9041=CARTESIAN_POINT('Ctrl Pts',(26.040864706517,45.3830586252745,75.3990270570443)) ;
#9042=CARTESIAN_POINT('Ctrl Pts',(26.0203779564856,45.3830586252741,75.4208777603213)) ;
#9043=CARTESIAN_POINT('Ctrl Pts',(25.9902687734762,45.3830586252741,75.4690276156026)) ;
#9044=CARTESIAN_POINT('Ctrl Pts',(25.980120414945,45.3830586252741,75.4946011380552)) ;
#9045=CARTESIAN_POINT('Ctrl Pts',(25.9733020175168,45.3830586252741,75.5359676129567)) ;
#9046=CARTESIAN_POINT('Ctrl Pts',(25.972614510739,45.3830586252741,75.5506847426767)) ;
#9047=CARTESIAN_POINT('Ctrl Pts',(25.97483660085,45.3830586252741,75.5789335804189)) ;
#9048=CARTESIAN_POINT('Ctrl Pts',(25.9774754040238,45.3830586252741,75.5923171052466)) ;
#9049=CARTESIAN_POINT('Ctrl Pts',(25.9816871705707,45.3830586252741,75.6052793419901)) ;
#9050=CARTESIAN_POINT('',(31.9584809790255,45.3830586252741,94.000023827484)) ;
#9051=CARTESIAN_POINT('',(31.9584809790255,45.3830586252741,94.000023827484)) ;
#9052=CARTESIAN_POINT('Origin',(25.3010853649595,45.3830586252741,96.1631427881087)) ;
#9053=CARTESIAN_POINT('Ctrl Pts',(25.7953201020593,45.38305024022,75.3553561083262)) ;
#9054=CARTESIAN_POINT('Ctrl Pts',(25.465542879517,45.9804808943737,75.46250745988)) ;
#9055=CARTESIAN_POINT('Ctrl Pts',(25.1272856995576,46.5779115664506,75.5387734998541)) ;
#9056=CARTESIAN_POINT('Ctrl Pts',(24.7890308984242,47.1753380370388,75.61503900348)) ;
#9057=CARTESIAN_POINT('Ctrl Pts',(24.4451821397366,47.772764507627,75.6597689563314)) ;
#9058=CARTESIAN_POINT('Ctrl Pts',(24.101333381049,48.3701909782152,75.7044989091829)) ;
#9059=CARTESIAN_POINT('Ctrl Pts',(23.7548242611786,48.9676174488035,75.7173116910735)) ;
#9060=CARTESIAN_POINT('Ctrl Pts',(23.4083151413083,49.5650439193917,75.7301244729642)) ;
#9061=CARTESIAN_POINT('Ctrl Pts',(23.0621019538903,50.16247038998,75.7109107697566)) ;
#9062=CARTESIAN_POINT('Ctrl Pts',(22.7158887664722,50.7598968605682,75.6916970665491)) ;
#9063=CARTESIAN_POINT('Ctrl Pts',(22.3729252803503,51.3573233311564,75.6406208027845)) ;
#9064=CARTESIAN_POINT('Ctrl Pts',(22.0299617942283,51.9547498017447,75.5895445390199)) ;
#9065=CARTESIAN_POINT('Ctrl Pts',(21.6931740529404,52.5521762723329,75.5070414793717)) ;
#9066=CARTESIAN_POINT('Ctrl Pts',(21.3563863116525,53.1496027429211,75.4245384197236)) ;
#9067=CARTESIAN_POINT('Ctrl Pts',(21.0286476694594,53.7470292135094,75.311312451207)) ;
#9068=CARTESIAN_POINT('Ctrl Pts',(20.7009090272663,54.3444556840976,75.1980864826905)) ;
#9069=CARTESIAN_POINT('Ctrl Pts',(20.3850156347058,54.9418821546858,75.0551036093466)) ;
#9070=CARTESIAN_POINT('Ctrl Pts',(20.0691222421452,55.5393086252741,74.9121207360026)) ;
#9071=CARTESIAN_POINT('Ctrl Pts',(19.7677691902617,56.1367350958623,74.7406008372924)) ;
#9072=CARTESIAN_POINT('Ctrl Pts',(19.4664161383782,56.7341615664506,74.5690809385821)) ;
#9073=CARTESIAN_POINT('Ctrl Pts',(19.1821744651562,57.3315880370388,74.3704873618051)) ;
#9074=CARTESIAN_POINT('Ctrl Pts',(18.9320941337912,57.8572133193466,74.1957615838275)) ;
#9075=CARTESIAN_POINT('Ctrl Pts',(18.6970309148446,58.3830758086166,74.0013019409091)) ;
#9076=CARTESIAN_POINT('Ctrl Pts',(34.2933044184902,45.38305024022,101.509404792186)) ;
#9077=CARTESIAN_POINT('Ctrl Pts',(32.7543440466264,45.9804808943737,102.00944443277)) ;
#9078=CARTESIAN_POINT('Ctrl Pts',(31.1758105401488,46.5779115664505,102.365352619316)) ;
#9079=CARTESIAN_POINT('Ctrl Pts',(29.5972881348596,47.1753380370388,102.721258302903)) ;
#9080=CARTESIAN_POINT('Ctrl Pts',(27.9926605943175,47.772764507627,102.929998082877)) ;
#9081=CARTESIAN_POINT('Ctrl Pts',(26.3880330537754,48.3701909782152,103.13873786285)) ;
#9082=CARTESIAN_POINT('Ctrl Pts',(24.7709904943805,48.9676174488035,103.198530845007)) ;
#9083=CARTESIAN_POINT('Ctrl Pts',(23.1539479349856,49.5650439193917,103.258323827163)) ;
#9084=CARTESIAN_POINT('Ctrl Pts',(21.5382863937015,50.16247038998,103.168659878861)) ;
#9085=CARTESIAN_POINT('Ctrl Pts',(19.9226248524173,50.7598968605682,103.078995930559)) ;
#9086=CARTESIAN_POINT('Ctrl Pts',(18.3221285838481,51.3573233311564,102.840640032991)) ;
#9087=CARTESIAN_POINT('Ctrl Pts',(16.7216323152788,51.9547498017447,102.602284135423)) ;
#9088=CARTESIAN_POINT('Ctrl Pts',(15.1499561892687,52.5521762723329,102.217269857065)) ;
#9089=CARTESIAN_POINT('Ctrl Pts',(13.5782800632586,53.1496027429211,101.832255578707)) ;
#9090=CARTESIAN_POINT('Ctrl Pts',(12.0488330663575,53.7470292135094,101.30386772563)) ;
#9091=CARTESIAN_POINT('Ctrl Pts',(10.5193860694563,54.3444556840976,100.775479872552)) ;
#9092=CARTESIAN_POINT('Ctrl Pts',(9.04521690417374,54.9418821546858,100.108226463614)) ;
#9093=CARTESIAN_POINT('Ctrl Pts',(7.57104773889119,55.5393086252741,99.4409730546758)) ;
#9094=CARTESIAN_POINT('Ctrl Pts',(6.16473349676808,56.1367350958623,98.6405468606946)) ;
#9095=CARTESIAN_POINT('Ctrl Pts',(4.75841925464496,56.7341615664505,97.8401206667133)) ;
#9096=CARTESIAN_POINT('Ctrl Pts',(3.43195811294263,57.3315880370388,96.9133506417539)) ;
#9097=CARTESIAN_POINT('Ctrl Pts',(2.26491656657273,57.8572133193466,96.0979636778584)) ;
#9098=CARTESIAN_POINT('Ctrl Pts',(1.16795487815523,58.3830758086166,95.1904853442392)) ;
#9099=CARTESIAN_POINT('',(6.29012224935737,58.3353824278239,89.1555480018396)) ;
#9100=CARTESIAN_POINT('',(18.5844591889196,58.2172712656977,74.2942518441039)) ;
#9101=CARTESIAN_POINT('Ctrl Pts',(6.2901222493574,58.3353824278239,89.1555480018396)) ;
#9102=CARTESIAN_POINT('Ctrl Pts',(7.9341551303245,58.3308357090662,87.1682536299972)) ;
#9103=CARTESIAN_POINT('Ctrl Pts',(9.7767093026726,58.3244410141138,84.9409882395581)) ;
#9104=CARTESIAN_POINT('Ctrl Pts',(12.9422976968674,58.3066351840462,81.1144492012072)) ;
#9105=CARTESIAN_POINT('Ctrl Pts',(16.4192438916362,58.2895264446024,76.9115432349964)) ;
#9106=CARTESIAN_POINT('Ctrl Pts',(18.5844570548379,58.2172696107887,74.2942501243266)) ;
#9107=CARTESIAN_POINT('Ctrl Pts',(18.5844591889196,58.2172712656977,74.2942518441039)) ;
#9108=CARTESIAN_POINT('Ctrl Pts',(18.7101800665396,57.9495340002374,74.3955675893354)) ;
#9109=CARTESIAN_POINT('Ctrl Pts',(18.839000643377,57.6819084045899,74.4929334901453)) ;
#9110=CARTESIAN_POINT('Ctrl Pts',(18.9705754040965,57.4145313636573,74.5861224918267)) ;
#9111=CARTESIAN_POINT('Ctrl Pts',(19.0927155785282,57.1663266301663,74.6726293633439)) ;
#9112=CARTESIAN_POINT('Ctrl Pts',(19.2172631286827,56.9182638872732,74.7555641589253)) ;
#9113=CARTESIAN_POINT('Ctrl Pts',(19.3440508641358,56.6702295478716,74.8348238368534)) ;
#9114=CARTESIAN_POINT('Ctrl Pts',(19.3538444462716,56.651070402338,74.8409461653505)) ;
#9115=CARTESIAN_POINT('Ctrl Pts',(19.3636520874551,56.6319118940955,74.8470470101628)) ;
#9116=CARTESIAN_POINT('Ctrl Pts',(19.3734736865329,56.6127538456681,74.8531263066697)) ;
#9117=CARTESIAN_POINT('Ctrl Pts',(19.5022865921394,56.361490903236,74.9328579105444)) ;
#9118=CARTESIAN_POINT('Ctrl Pts',(19.6334867409694,56.1103350670491,75.0088728946902)) ;
#9119=CARTESIAN_POINT('Ctrl Pts',(19.7667733325224,55.8590202585562,75.0809886233964)) ;
#9120=CARTESIAN_POINT('Ctrl Pts',(19.7752158365134,55.8431017310511,75.0855565046838)) ;
#9121=CARTESIAN_POINT('Ctrl Pts',(19.7836664501678,55.8271830724926,75.0901086434416)) ;
#9122=CARTESIAN_POINT('Ctrl Pts',(19.7921251649139,55.8112643008986,75.0946450326021)) ;
#9123=CARTESIAN_POINT('Ctrl Pts',(19.927388862856,55.5567064895584,75.1671866410578)) ;
#9124=CARTESIAN_POINT('Ctrl Pts',(20.0647904015071,55.3019957844152,75.2357353524665)) ;
#9125=CARTESIAN_POINT('Ctrl Pts',(20.2043059526064,55.0471908391173,75.3002604585485)) ;
#9126=CARTESIAN_POINT('Ctrl Pts',(20.2112552757719,55.034498906963,75.303474478856)) ;
#9127=CARTESIAN_POINT('Ctrl Pts',(20.2182098394889,55.0218058655745,75.3066784613102)) ;
#9128=CARTESIAN_POINT('Ctrl Pts',(20.2251695507038,55.0091118266698,75.3098723681775)) ;
#9129=CARTESIAN_POINT('Ctrl Pts',(20.3666875736652,54.7509925981976,75.3748169285795)) ;
#9130=CARTESIAN_POINT('Ctrl Pts',(20.510254348456,54.4926055130936,75.4355599269685)) ;
#9131=CARTESIAN_POINT('Ctrl Pts',(20.6552605035336,54.2345762733044,75.4918603128164)) ;
#9132=CARTESIAN_POINT('Ctrl Pts',(20.6605536210439,54.2251575070005,75.4939154294286)) ;
#9133=CARTESIAN_POINT('Ctrl Pts',(20.6658490728384,54.2157389752755,75.4959647949841)) ;
#9134=CARTESIAN_POINT('Ctrl Pts',(20.6711468481269,54.2063206495464,75.498008405768)) ;
#9135=CARTESIAN_POINT('Ctrl Pts',(20.8181077649379,53.9450551732693,75.5546984120534)) ;
#9136=CARTESIAN_POINT('Ctrl Pts',(20.9667953261445,53.6840579939653,75.6069349668757)) ;
#9137=CARTESIAN_POINT('Ctrl Pts',(21.1167903730235,53.4230444575826,75.6545818341298)) ;
#9138=CARTESIAN_POINT('Ctrl Pts',(21.1203326411854,53.416880387775,75.6557070578249)) ;
#9139=CARTESIAN_POINT('Ctrl Pts',(21.1238756222229,53.4107163827002,75.65682972301)) ;
#9140=CARTESIAN_POINT('Ctrl Pts',(21.127419315629,53.4045524432165,75.6579498295793)) ;
#9141=CARTESIAN_POINT('Ctrl Pts',(21.2793512822543,53.1402803009654,75.705973169749)) ;
#9142=CARTESIAN_POINT('Ctrl Pts',(21.4326359576011,52.876053372543,75.7493072487968)) ;
#9143=CARTESIAN_POINT('Ctrl Pts',(21.5872704788157,52.6118787196962,75.7879471921473)) ;
#9144=CARTESIAN_POINT('Ctrl Pts',(21.7452985588166,52.341906576048,75.8274351150965)) ;
#9145=CARTESIAN_POINT('Ctrl Pts',(21.9046488421704,52.0715787920638,75.8619872769898)) ;
#9146=CARTESIAN_POINT('Ctrl Pts',(22.0649600027153,51.8011908422986,75.8915185741482)) ;
#9147=CARTESIAN_POINT('Ctrl Pts',(22.0651612626675,51.8008513882913,75.8915556487189)) ;
#9148=CARTESIAN_POINT('Ctrl Pts',(22.0653625241294,51.8005119341973,75.8915927153756)) ;
#9149=CARTESIAN_POINT('Ctrl Pts',(22.0655637871,51.8001724800173,75.8916297741181)) ;
#9150=CARTESIAN_POINT('Ctrl Pts',(22.2239547698191,51.5330270582815,75.9207944566424)) ;
#9151=CARTESIAN_POINT('Ctrl Pts',(22.3836176559041,51.2655853544539,75.9451032765368)) ;
#9152=CARTESIAN_POINT('Ctrl Pts',(22.5435526953119,50.998401550286,75.9644006663621)) ;
#9153=CARTESIAN_POINT('Ctrl Pts',(22.5457025607775,50.9948100344075,75.9646600641283)) ;
#9154=CARTESIAN_POINT('Ctrl Pts',(22.5478524859572,50.9912185474961,75.9649185578724)) ;
#9155=CARTESIAN_POINT('Ctrl Pts',(22.5500024684931,50.9876270907846,75.9651761472065)) ;
#9156=CARTESIAN_POINT('Ctrl Pts',(22.7079994706035,50.7236996475827,75.9841057626246)) ;
#9157=CARTESIAN_POINT('Ctrl Pts',(22.8663838034903,50.4599498020535,75.9981821182529)) ;
#9158=CARTESIAN_POINT('Ctrl Pts',(23.0251541201544,50.1963788513668,76.0074120799679)) ;
#9159=CARTESIAN_POINT('Ctrl Pts',(23.0292590911529,50.189564283434,76.007650718562)) ;
#9160=CARTESIAN_POINT('Ctrl Pts',(23.0333642180568,50.1827500045964,76.007886111495)) ;
#9161=CARTESIAN_POINT('Ctrl Pts',(23.0374695044909,50.175936008737,76.0081182595862)) ;
#9162=CARTESIAN_POINT('Ctrl Pts',(23.1943074066204,49.9156148757611,76.0169872192053)) ;
#9163=CARTESIAN_POINT('Ctrl Pts',(23.3512376999488,49.6552611188171,76.0211072512855)) ;
#9164=CARTESIAN_POINT('Ctrl Pts',(23.5082061089285,49.3948957256022,76.0204931855221)) ;
#9165=CARTESIAN_POINT('Ctrl Pts',(23.5142878202418,49.3848079176936,76.0204693936602)) ;
#9166=CARTESIAN_POINT('Ctrl Pts',(23.5203694574972,49.3747203101764,76.0204384892973)) ;
#9167=CARTESIAN_POINT('Ctrl Pts',(23.5264510044697,49.364632925956,76.0204004728069)) ;
#9168=CARTESIAN_POINT('Ctrl Pts',(23.681442216326,49.1075509841643,76.0194316038757)) ;
#9169=CARTESIAN_POINT('Ctrl Pts',(23.8365783763701,48.8504690628024,76.0138346276243)) ;
#9170=CARTESIAN_POINT('Ctrl Pts',(23.9913881239066,48.5931578990174,76.0036143155886)) ;
#9171=CARTESIAN_POINT('Ctrl Pts',(23.9994194115387,48.5798089981878,76.0030841017813)) ;
#9172=CARTESIAN_POINT('Ctrl Pts',(24.0074500682842,48.566459068981,76.0025414286173)) ;
#9173=CARTESIAN_POINT('Ctrl Pts',(24.0154800122403,48.5531081058639,76.0019862962604)) ;
#9174=CARTESIAN_POINT('Ctrl Pts',(24.1683073257374,48.2990102146546,75.9914209190658)) ;
#9175=CARTESIAN_POINT('Ctrl Pts',(24.320977601014,48.0446012919295,75.9763394192743)) ;
#9176=CARTESIAN_POINT('Ctrl Pts',(24.4731100447151,47.7903648312084,75.9567599665068)) ;
#9177=CARTESIAN_POINT('Ctrl Pts',(24.4830339125752,47.7737805380753,75.9554827642394)) ;
#9178=CARTESIAN_POINT('Ctrl Pts',(24.492955861141,47.7571963611373,75.9541863741319)) ;
#9179=CARTESIAN_POINT('Ctrl Pts',(24.50287583425,47.7406123516807,75.9528707946832)) ;
#9180=CARTESIAN_POINT('Ctrl Pts',(24.6530188950513,47.4896062337405,75.9329589337344)) ;
#9181=CARTESIAN_POINT('Ctrl Pts',(24.8023159560001,47.2387261489803,75.9087129990594)) ;
#9182=CARTESIAN_POINT('Ctrl Pts',(24.9508196300929,46.9878897404751,75.8801450477756)) ;
#9183=CARTESIAN_POINT('Ctrl Pts',(24.9625073132173,46.9681481652139,75.8778966646015)) ;
#9184=CARTESIAN_POINT('Ctrl Pts',(24.9741897307449,46.9484074501543,75.8756215645657)) ;
#9185=CARTESIAN_POINT('Ctrl Pts',(24.9858668886883,46.9286675886392,75.8733197584537)) ;
#9186=CARTESIAN_POINT('Ctrl Pts',(25.1323624947587,46.6810214584402,75.8444424851415)) ;
#9187=CARTESIAN_POINT('Ctrl Pts',(25.2781273118314,46.4334531760666,75.8113320199874)) ;
#9188=CARTESIAN_POINT('Ctrl Pts',(25.4227590725841,46.1857600468476,75.7740795212884)) ;
#9189=CARTESIAN_POINT('Ctrl Pts',(25.4360537096591,46.1629919477676,75.7706552495533)) ;
#9190=CARTESIAN_POINT('Ctrl Pts',(25.4493390556513,46.140222308408,75.7671959063944)) ;
#9191=CARTESIAN_POINT('Ctrl Pts',(25.4626147718347,46.1174510138861,75.7637015657915)) ;
#9192=CARTESIAN_POINT('Ctrl Pts',(25.6052771603323,45.8727480373531,75.7261509756951)) ;
#9193=CARTESIAN_POINT('Ctrl Pts',(25.7469101647593,45.6279743432129,75.6845467079578)) ;
#9194=CARTESIAN_POINT('Ctrl Pts',(25.8874434877188,45.3830610445957,75.638885508351)) ;
#9195=CARTESIAN_POINT('',(25.8068141710837,48.5844537758935,103.144850199241)) ;
#9196=CARTESIAN_POINT('Ctrl Pts',(32.2277008466604,45.3830585486371,95.1522036362991)) ;
#9197=CARTESIAN_POINT('Ctrl Pts',(32.3031100938315,45.4231928249935,95.6688829820357)) ;
#9198=CARTESIAN_POINT('Ctrl Pts',(32.320119173168,45.4870033446877,96.190162540208)) ;
#9199=CARTESIAN_POINT('Ctrl Pts',(32.2390995479676,45.6539797372435,97.2319881208699)) ;
#9200=CARTESIAN_POINT('Ctrl Pts',(32.1390467146082,45.7573388893141,97.7487283877929)) ;
#9201=CARTESIAN_POINT('Ctrl Pts',(31.7108073456657,46.0833507061677,99.1224310140683)) ;
#9202=CARTESIAN_POINT('Ctrl Pts',(31.2706997360599,46.3336877227689,99.9279524714847)) ;
#9203=CARTESIAN_POINT('Ctrl Pts',(30.0747052050763,46.9107591797133,101.375467312635)) ;
#9204=CARTESIAN_POINT('Ctrl Pts',(29.3055362183394,47.2383195349502,101.98507439633)) ;
#9205=CARTESIAN_POINT('Ctrl Pts',(27.6191245040703,47.9083523080808,102.832323345458)) ;
#9206=CARTESIAN_POINT('Ctrl Pts',(26.722903131973,48.2450338483641,103.078492136777)) ;
#9207=CARTESIAN_POINT('Ctrl Pts',(25.8068141710837,48.5844537758935,103.144850199241)) ;
#9208=CARTESIAN_POINT('',(25.7569277250234,48.6029307720944,103.148213134921)) ;
#9209=CARTESIAN_POINT('Origin',(28.1803190987662,48.3559725194583,140.311274111017)) ;
#9210=CARTESIAN_POINT('',(8.73526681379954,55.0677871747466,99.9661893007231)) ;
#9211=CARTESIAN_POINT('Ctrl Pts',(25.7569277250234,48.6029307720944,103.148213134921)) ;
#9212=CARTESIAN_POINT('Ctrl Pts',(25.2643121406148,48.785356686239,103.180289412696)) ;
#9213=CARTESIAN_POINT('Ctrl Pts',(24.7709904943805,48.9676174488035,103.198530845007)) ;
#9214=CARTESIAN_POINT('Ctrl Pts',(23.1539479349856,49.5650439193917,103.258323827163)) ;
#9215=CARTESIAN_POINT('Ctrl Pts',(21.5382863937015,50.16247038998,103.168659878861)) ;
#9216=CARTESIAN_POINT('Ctrl Pts',(19.9226248524173,50.7598968605682,103.078995930559)) ;
#9217=CARTESIAN_POINT('Ctrl Pts',(18.3221285838481,51.3573233311564,102.840640032991)) ;
#9218=CARTESIAN_POINT('Ctrl Pts',(16.7216323152788,51.9547498017447,102.602284135423)) ;
#9219=CARTESIAN_POINT('Ctrl Pts',(15.1499561892687,52.5521762723329,102.217269857065)) ;
#9220=CARTESIAN_POINT('Ctrl Pts',(13.5782800632586,53.1496027429211,101.832255578707)) ;
#9221=CARTESIAN_POINT('Ctrl Pts',(12.0488330663575,53.7470292135094,101.30386772563)) ;
#9222=CARTESIAN_POINT('Ctrl Pts',(10.5193860694563,54.3444556840976,100.775479872552)) ;
#9223=CARTESIAN_POINT('Ctrl Pts',(9.04521690417374,54.9418821546858,100.108226463614)) ;
#9224=CARTESIAN_POINT('Ctrl Pts',(8.88991083437399,55.0048219850164,100.0379302541)) ;
#9225=CARTESIAN_POINT('Ctrl Pts',(8.73526681379953,55.0677871747466,99.9661893007231)) ;
#9226=CARTESIAN_POINT('',(8.68996421845689,55.0862551252693,99.9450317561577)) ;
#9227=CARTESIAN_POINT('Origin',(-6.32810000537899,55.5493242894856,132.402663943764)) ;
#9228=CARTESIAN_POINT('Ctrl Pts',(8.68996421845687,55.0862551252692,99.9450317561577)) ;
#9229=CARTESIAN_POINT('Ctrl Pts',(8.20077668425168,55.2861476427454,99.7135814400466)) ;
#9230=CARTESIAN_POINT('Ctrl Pts',(7.73969544475074,55.4856144064204,99.4260005287769)) ;
#9231=CARTESIAN_POINT('Ctrl Pts',(6.86222930708719,55.8948727823203,98.7254146660119)) ;
#9232=CARTESIAN_POINT('Ctrl Pts',(6.45404498576417,56.1030297966035,98.3070128505722)) ;
#9233=CARTESIAN_POINT('Ctrl Pts',(5.52344278067351,56.6395229540351,97.0772238444848)) ;
#9234=CARTESIAN_POINT('Ctrl Pts',(5.1037113359308,56.9553077214542,96.1962925358796)) ;
#9235=CARTESIAN_POINT('Ctrl Pts',(4.66774586592465,57.5027528833965,94.3787099674685)) ;
#9236=CARTESIAN_POINT('Ctrl Pts',(4.62591980549989,57.7356392971192,93.4655076450606)) ;
#9237=CARTESIAN_POINT('Ctrl Pts',(4.86507457348184,58.0583687617078,91.8978184860504)) ;
#9238=CARTESIAN_POINT('Ctrl Pts',(5.06231793135134,58.1679507457142,91.2466136289794)) ;
#9239=CARTESIAN_POINT('Ctrl Pts',(5.60181878346812,58.3023924932056,90.1031845606475)) ;
#9240=CARTESIAN_POINT('Ctrl Pts',(5.91644124082818,58.3364158757984,89.6072507467857)) ;
#9241=CARTESIAN_POINT('Ctrl Pts',(6.29012224935736,58.3353824278239,89.1555480018396)) ;
#9242=CARTESIAN_POINT('Ctrl Pts',(34.3883885914319,45.3830585852922,101.478510132603)) ;
#9243=CARTESIAN_POINT('Ctrl Pts',(32.8508673372113,45.9804850758286,101.982942280144)) ;
#9244=CARTESIAN_POINT('Ctrl Pts',(31.2733617497745,46.5779115664505,102.343358040426)) ;
#9245=CARTESIAN_POINT('Ctrl Pts',(29.6958562152367,47.1753380370388,102.703773788621)) ;
#9246=CARTESIAN_POINT('Ctrl Pts',(28.0918250713921,47.772764507627,102.917098219058)) ;
#9247=CARTESIAN_POINT('Ctrl Pts',(26.4877939275474,48.3701909782152,103.130422649496)) ;
#9248=CARTESIAN_POINT('Ctrl Pts',(24.8709222025499,48.9676174488035,103.19483575335)) ;
#9249=CARTESIAN_POINT('Ctrl Pts',(23.2540504775523,49.5650439193917,103.259248857204)) ;
#9250=CARTESIAN_POINT('Ctrl Pts',(21.6381327508665,50.16247038998,103.174201084585)) ;
#9251=CARTESIAN_POINT('Ctrl Pts',(20.0222150241807,50.7598968605682,103.089153311966)) ;
#9252=CARTESIAN_POINT('Ctrl Pts',(18.4210377360943,51.3573233311564,102.855370260482)) ;
#9253=CARTESIAN_POINT('Ctrl Pts',(16.8198604480078,51.9547498017447,102.621587208999)) ;
#9254=CARTESIAN_POINT('Ctrl Pts',(15.2470842785835,52.5521762723329,102.241063433216)) ;
#9255=CARTESIAN_POINT('Ctrl Pts',(13.6743081091592,53.1496027429211,101.860539657434)) ;
#9256=CARTESIAN_POINT('Ctrl Pts',(12.1433514301292,53.7470292135094,101.336521652039)) ;
#9257=CARTESIAN_POINT('Ctrl Pts',(10.6123947510992,54.3444556840976,100.812503646644)) ;
#9258=CARTESIAN_POINT('Ctrl Pts',(9.13631914504893,54.9418821546858,100.149462148494)) ;
#9259=CARTESIAN_POINT('Ctrl Pts',(7.66024353899866,55.5393086252741,99.4864206503448)) ;
#9260=CARTESIAN_POINT('Ctrl Pts',(6.25164236254934,56.1367350958623,98.6900124957215)) ;
#9261=CARTESIAN_POINT('Ctrl Pts',(4.84304118610003,56.7341615664505,97.8936043410982)) ;
#9262=CARTESIAN_POINT('Ctrl Pts',(3.51393212783033,57.3315880370388,96.9706242035708)) ;
#9263=CARTESIAN_POINT('Ctrl Pts',(2.34451316548462,57.857234776835,96.1585384924868)) ;
#9264=CARTESIAN_POINT('Ctrl Pts',(1.24491679165593,58.3831186720347,95.2541537699803)) ;
#9265=CARTESIAN_POINT('Ctrl Pts',(25.8904211471758,45.3830585852922,75.3244559053118)) ;
#9266=CARTESIAN_POINT('Ctrl Pts',(25.5620748354161,45.9804850758286,75.4360032937205)) ;
#9267=CARTESIAN_POINT('Ctrl Pts',(25.2248368963556,46.5779115664506,75.5167788640701)) ;
#9268=CARTESIAN_POINT('Ctrl Pts',(24.8875989686039,47.1753380370388,75.5975544317111)) ;
#9269=CARTESIAN_POINT('Ctrl Pts',(24.5443466092877,47.772764507627,75.6468690346784)) ;
#9270=CARTESIAN_POINT('Ctrl Pts',(24.2010942499714,48.3701909782152,75.6961836376457)) ;
#9271=CARTESIAN_POINT('Ctrl Pts',(23.854755967193,48.9676174488035,75.7136165411346)) ;
#9272=CARTESIAN_POINT('Ctrl Pts',(23.5084176844145,49.5650439193917,75.7310494446235)) ;
#9273=CARTESIAN_POINT('Ctrl Pts',(23.1619483142871,50.16247038998,75.7164519172482)) ;
#9274=CARTESIAN_POINT('Ctrl Pts',(22.8154789441596,50.7598968605682,75.7018543898729)) ;
#9275=CARTESIAN_POINT('Ctrl Pts',(22.4718344411874,51.3573233311564,75.6553509725899)) ;
#9276=CARTESIAN_POINT('Ctrl Pts',(22.1281899382152,51.9547498017447,75.608847555307)) ;
#9277=CARTESIAN_POINT('Ctrl Pts',(21.7903021561321,52.5521762723329,75.530834998876)) ;
#9278=CARTESIAN_POINT('Ctrl Pts',(21.4524143740489,53.1496027429211,75.452822442445)) ;
#9279=CARTESIAN_POINT('Ctrl Pts',(21.1231660522755,53.7470292135094,75.3439663224911)) ;
#9280=CARTESIAN_POINT('Ctrl Pts',(20.7939177305022,54.3444556840976,75.2351102025371)) ;
#9281=CARTESIAN_POINT('Ctrl Pts',(20.4761178996304,54.9418821546858,75.096339241094)) ;
#9282=CARTESIAN_POINT('Ctrl Pts',(20.1583180687586,55.5393086252741,74.9575682796509)) ;
#9283=CARTESIAN_POINT('Ctrl Pts',(19.8546780848923,56.1367350958623,74.7900664216324)) ;
#9284=CARTESIAN_POINT('Ctrl Pts',(19.551038101026,56.7341615664506,74.6225645636139)) ;
#9285=CARTESIAN_POINT('Ctrl Pts',(19.264148513447,57.3315880370388,74.4277608758131)) ;
#9286=CARTESIAN_POINT('Ctrl Pts',(19.0117282009625,57.8572347768351,74.2563625055804)) ;
#9287=CARTESIAN_POINT('Ctrl Pts',(18.7740631193741,58.3831186720347,74.0650284404828)) ;
#9288=CARTESIAN_POINT('',(18.5858460045131,58.3830537363182,74.292544600312)) ;
#9289=CARTESIAN_POINT('Ctrl Pts',(25.9816821278123,45.3830674541116,75.6052810522977)) ;
#9290=CARTESIAN_POINT('Ctrl Pts',(25.9720536409296,45.3999249614356,75.6085466570867)) ;
#9291=CARTESIAN_POINT('Ctrl Pts',(25.9622835986064,45.4170195560991,75.6118389611852)) ;
#9292=CARTESIAN_POINT('Ctrl Pts',(25.9428699827234,45.450966082336,75.6183380969714)) ;
#9293=CARTESIAN_POINT('Ctrl Pts',(25.9331581705972,45.4679374856696,75.6215680725326)) ;
#9294=CARTESIAN_POINT('Ctrl Pts',(25.9040078813387,45.5188462146271,75.6311992306336)) ;
#9295=CARTESIAN_POINT('Ctrl Pts',(25.8845545514463,45.5527780591992,75.6375416449359)) ;
#9296=CARTESIAN_POINT('Ctrl Pts',(25.8261364256564,45.6545524513434,75.6563338676956)) ;
#9297=CARTESIAN_POINT('Ctrl Pts',(25.7871134891735,45.7223738576059,75.6685486410987)) ;
#9298=CARTESIAN_POINT('Ctrl Pts',(25.6987804559921,45.8755455989773,75.6954380806355)) ;
#9299=CARTESIAN_POINT('Ctrl Pts',(25.6494252923191,45.9608834226817,75.709929590608)) ;
#9300=CARTESIAN_POINT('Ctrl Pts',(25.5708698027494,46.096346675625,75.7321540649685)) ;
#9301=CARTESIAN_POINT('Ctrl Pts',(25.5417333879409,46.1464973799218,75.7402142926808)) ;
#9302=CARTESIAN_POINT('Ctrl Pts',(25.3777882376432,46.4282028809694,75.7845431297761)) ;
#9303=CARTESIAN_POINT('Ctrl Pts',(25.2421515380204,46.6594344485447,75.8173327836383)) ;
#9304=CARTESIAN_POINT('Ctrl Pts',(25.082837649862,46.9296827699039,75.8513551760635)) ;
#9305=CARTESIAN_POINT('Ctrl Pts',(25.0597605868494,46.968795042417,75.8561741409081)) ;
#9306=CARTESIAN_POINT('Ctrl Pts',(24.8937141271844,47.2499758749388,75.8900633827158)) ;
#9307=CARTESIAN_POINT('Ctrl Pts',(24.7501105114405,47.4918541916406,75.9151945113985)) ;
#9308=CARTESIAN_POINT('Ctrl Pts',(24.4382706209287,48.0143150858147,75.9608047711095)) ;
#9309=CARTESIAN_POINT('Ctrl Pts',(24.2699414562195,48.2952954282308,75.9798403599875)) ;
#9310=CARTESIAN_POINT('Ctrl Pts',(24.0910078683281,48.5931204307079,75.9941989442598)) ;
#9311=CARTESIAN_POINT('Ctrl Pts',(24.0807918914205,48.6101204742723,75.9949984353586)) ;
#9312=CARTESIAN_POINT('Ctrl Pts',(23.9119431175511,48.8910362150329,76.0078771021127)) ;
#9313=CARTESIAN_POINT('Ctrl Pts',(23.7528087469497,49.1549226796789,76.0151262737856)) ;
#9314=CARTESIAN_POINT('Ctrl Pts',(23.5900902749489,49.4249376060057,76.0175458523535)) ;
#9315=CARTESIAN_POINT('Ctrl Pts',(23.5865567043535,49.430801123754,76.0175959960367)) ;
#9316=CARTESIAN_POINT('Ctrl Pts',(23.420298917879,49.7066812295575,76.0198423852037)) ;
#9317=CARTESIAN_POINT('Ctrl Pts',(23.2573680914076,49.9768666464288,76.0169512266826)) ;
#9318=CARTESIAN_POINT('Ctrl Pts',(23.0912143366874,50.2527043291671,76.0087719319334)) ;
#9319=CARTESIAN_POINT('Ctrl Pts',(23.0879880363181,50.2580605419638,76.0086111000024)) ;
#9320=CARTESIAN_POINT('Ctrl Pts',(22.9250557359098,50.5285623062303,76.0003873586263)) ;
#9321=CARTESIAN_POINT('Ctrl Pts',(22.7655562097403,50.794089282034,75.9874165770804)) ;
#9322=CARTESIAN_POINT('Ctrl Pts',(22.596220584203,51.0767673302901,75.9683691764023)) ;
#9323=CARTESIAN_POINT('Ctrl Pts',(22.5861929542279,51.09350971285,75.9672215336923)) ;
#9324=CARTESIAN_POINT('Ctrl Pts',(22.4915033167505,51.2516332986598,75.9561983324922)) ;
#9325=CARTESIAN_POINT('Ctrl Pts',(22.4068327694471,51.3931664826184,75.944930972281)) ;
#9326=CARTESIAN_POINT('Ctrl Pts',(22.2548906854115,51.6479675595709,75.922163245892)) ;
#9327=CARTESIAN_POINT('Ctrl Pts',(22.1875111509901,51.7612319406822,75.9111590655696)) ;
#9328=CARTESIAN_POINT('Ctrl Pts',(22.1035923597581,51.9026374456282,75.8963208743334)) ;
#9329=CARTESIAN_POINT('Ctrl Pts',(22.0868835458075,51.9308091085122,75.8933101583207)) ;
#9330=CARTESIAN_POINT('Ctrl Pts',(21.9025872293205,52.2417252333167,75.8594806951164)) ;
#9331=CARTESIAN_POINT('Ctrl Pts',(21.7360368649525,52.5241195492734,75.8232276595509)) ;
#9332=CARTESIAN_POINT('Ctrl Pts',(21.4355297941431,53.0381974993209,75.7474217195157)) ;
#9333=CARTESIAN_POINT('Ctrl Pts',(21.3011963380331,53.2697333986845,75.7096734001977)) ;
#9334=CARTESIAN_POINT('Ctrl Pts',(21.1385342177892,53.5522259966922,75.6592141409401)) ;
#9335=CARTESIAN_POINT('Ctrl Pts',(21.109245102224,53.6031771340245,75.6499383146778)) ;
#9336=CARTESIAN_POINT('Ctrl Pts',(20.9536831119847,53.8742457620906,75.599659155911)) ;
#9337=CARTESIAN_POINT('Ctrl Pts',(20.8283529470414,54.0945463050606,75.5555823028404)) ;
#9338=CARTESIAN_POINT('Ctrl Pts',(20.6690101501099,54.3774106831927,75.4949256517854)) ;
#9339=CARTESIAN_POINT('Ctrl Pts',(20.6339184787535,54.4398806254215,75.48127574604)) ;
#9340=CARTESIAN_POINT('Ctrl Pts',(20.481821152551,54.711432139282,75.4208404961403)) ;
#9341=CARTESIAN_POINT('Ctrl Pts',(20.3657022613531,54.9205828276725,75.3714026715031)) ;
#9342=CARTESIAN_POINT('Ctrl Pts',(20.2104748018518,55.203368432954,75.3008285804407)) ;
#9343=CARTESIAN_POINT('Ctrl Pts',(20.1700922605189,55.2772338818091,75.2820492977946)) ;
#9344=CARTESIAN_POINT('Ctrl Pts',(20.0224335966246,55.5485088102294,75.2118349432992)) ;
#9345=CARTESIAN_POINT('Ctrl Pts',(19.916228046497,55.7457837763575,75.1583211431054)) ;
#9346=CARTESIAN_POINT('Ctrl Pts',(19.7659277041273,56.0282588904728,75.0782259130373)) ;
#9347=CARTESIAN_POINT('Ctrl Pts',(19.720810206197,56.1134884206069,75.0536060353448)) ;
#9348=CARTESIAN_POINT('Ctrl Pts',(19.5781288974087,56.3844426291216,74.9739057491897)) ;
#9349=CARTESIAN_POINT('Ctrl Pts',(19.481611211323,56.5701302611202,74.9172297832555)) ;
#9350=CARTESIAN_POINT('Ctrl Pts',(19.3366723231393,56.8526653482991,74.8278700217508)) ;
#9351=CARTESIAN_POINT('Ctrl Pts',(19.2873541178717,56.9494716030763,74.7966940866653)) ;
#9352=CARTESIAN_POINT('Ctrl Pts',(19.1502669264902,57.2204413601227,74.7078682177841)) ;
#9353=CARTESIAN_POINT('Ctrl Pts',(19.0632399891367,57.394657675533,74.6489470349753)) ;
#9354=CARTESIAN_POINT('Ctrl Pts',(18.9240097385661,57.6774250653638,74.5505202852794)) ;
#9355=CARTESIAN_POINT('Ctrl Pts',(18.8710615649226,57.7859396412685,74.5120812548434)) ;
#9356=CARTESIAN_POINT('Ctrl Pts',(18.8055003584704,57.9216227418848,74.4632125950281)) ;
#9357=CARTESIAN_POINT('Ctrl Pts',(18.7924327198245,57.948727891259,74.4534079705152)) ;
#9358=CARTESIAN_POINT('Ctrl Pts',(18.7467598748858,58.0436810159814,74.4189146837387)) ;
#9359=CARTESIAN_POINT('Ctrl Pts',(18.7143072863786,58.1115399743058,74.394001847081)) ;
#9360=CARTESIAN_POINT('Ctrl Pts',(18.6659139020866,58.2133484522828,74.356242806694)) ;
#9361=CARTESIAN_POINT('Ctrl Pts',(18.6498317153866,58.2472850649065,74.3435925846863)) ;
#9362=CARTESIAN_POINT('Ctrl Pts',(18.6257803686513,58.2981973836588,74.3245201977021)) ;
#9363=CARTESIAN_POINT('Ctrl Pts',(18.6177752421485,58.3151693899113,74.3181465595116)) ;
#9364=CARTESIAN_POINT('Ctrl Pts',(18.607604619674,58.3367668565651,74.3100160221478)) ;
#9365=CARTESIAN_POINT('Ctrl Pts',(18.6054237775714,58.3413999128696,74.3082707117144)) ;
#9366=CARTESIAN_POINT('Ctrl Pts',(18.5974199895112,58.3584108602029,74.3018582790177)) ;
#9367=CARTESIAN_POINT('Ctrl Pts',(18.5915987969254,58.3707975233387,74.2971806666215)) ;
#9368=CARTESIAN_POINT('Ctrl Pts',(18.5858469328057,58.3830508753329,74.2925453446431)) ;
#9369=CARTESIAN_POINT('',(6.29012224935737,58.3831162793798,89.1555480018396)) ;
#9370=CARTESIAN_POINT('Ctrl Pts',(18.5858590582705,58.3830900980199,74.2925553933006)) ;
#9371=CARTESIAN_POINT('Ctrl Pts',(16.5365695895273,58.383105259385,76.7697208287716)) ;
#9372=CARTESIAN_POINT('Ctrl Pts',(14.4872801207512,58.3831073991803,79.2468862642824)) ;
#9373=CARTESIAN_POINT('Ctrl Pts',(10.3887011844437,58.3831134572106,84.2012171337991)) ;
#9374=CARTESIAN_POINT('Ctrl Pts',(8.33941171690048,58.3831150235129,86.6783825678194)) ;
#9375=CARTESIAN_POINT('Ctrl Pts',(6.2901222493574,58.3831162793798,89.1555480018396)) ;
#9376=CARTESIAN_POINT('',(8.73523672734845,55.104724217109,99.9662540836333)) ;
#9377=CARTESIAN_POINT('Ctrl Pts',(6.29012224935736,58.3831162793798,89.1555480018396)) ;
#9378=CARTESIAN_POINT('Ctrl Pts',(5.91420081213285,58.3831165097559,89.6099589598563)) ;
#9379=CARTESIAN_POINT('Ctrl Pts',(5.59809067175723,58.3477204548742,90.1090822491473)) ;
#9380=CARTESIAN_POINT('Ctrl Pts',(5.05681898264549,58.2097833704153,91.2606504993859)) ;
#9381=CARTESIAN_POINT('Ctrl Pts',(4.85984853002451,58.0979491851445,91.9168709057473)) ;
#9382=CARTESIAN_POINT('Ctrl Pts',(4.62536151099518,57.7707078254696,93.4903816655359)) ;
#9383=CARTESIAN_POINT('Ctrl Pts',(4.67047634429036,57.5360202457534,94.4039684820573)) ;
#9384=CARTESIAN_POINT('Ctrl Pts',(5.11328015675259,56.9856758817168,96.220706550885)) ;
#9385=CARTESIAN_POINT('Ctrl Pts',(5.53647004679195,56.6687344805943,97.1004478735331)) ;
#9386=CARTESIAN_POINT('Ctrl Pts',(6.47458953048251,56.1294192803767,98.3303404896527)) ;
#9387=CARTESIAN_POINT('Ctrl Pts',(6.88771640637359,55.9194276565173,98.7498321799113)) ;
#9388=CARTESIAN_POINT('Ctrl Pts',(7.77518736240662,55.5068628236254,99.4502708040986)) ;
#9389=CARTESIAN_POINT('Ctrl Pts',(8.24115253357343,55.3059550653477,99.7367917164622)) ;
#9390=CARTESIAN_POINT('Ctrl Pts',(8.73523672734845,55.104724217109,99.9662540836333)) ;
#9391=CARTESIAN_POINT('',(25.7569323765141,48.6398835186857,103.148284411731)) ;
#9392=CARTESIAN_POINT('Ctrl Pts',(25.7569323765141,48.6398835186857,103.148284411731)) ;
#9393=CARTESIAN_POINT('Ctrl Pts',(25.3142223238036,48.8038201453524,103.177175458668)) ;
#9394=CARTESIAN_POINT('Ctrl Pts',(24.8709222003948,48.9676174488035,103.194835695068)) ;
#9395=CARTESIAN_POINT('Ctrl Pts',(23.2540504780917,49.5650439193917,103.259248798822)) ;
#9396=CARTESIAN_POINT('Ctrl Pts',(21.6381327540982,50.16247038998,103.174201026353)) ;
#9397=CARTESIAN_POINT('Ctrl Pts',(20.0222150301047,50.7598968605682,103.089153253883)) ;
#9398=CARTESIAN_POINT('Ctrl Pts',(18.4210377446852,51.3573233311564,102.855370202796)) ;
#9399=CARTESIAN_POINT('Ctrl Pts',(16.8198604592657,51.9547498017447,102.62158715171)) ;
#9400=CARTESIAN_POINT('Ctrl Pts',(15.2470842924603,52.5521762723329,102.241063376569)) ;
#9401=CARTESIAN_POINT('Ctrl Pts',(13.6743081256549,53.1496027429211,101.860539601428)) ;
#9402=CARTESIAN_POINT('Ctrl Pts',(12.1433514491735,53.7470292135094,101.336521596914)) ;
#9403=CARTESIAN_POINT('Ctrl Pts',(10.6123947726921,54.3444556840976,100.812503592399)) ;
#9404=CARTESIAN_POINT('Ctrl Pts',(9.13631916909835,54.9418821546858,100.149462095362)) ;
#9405=CARTESIAN_POINT('Ctrl Pts',(8.93520090615318,55.0232827101246,100.059121360903)) ;
#9406=CARTESIAN_POINT('Ctrl Pts',(8.73523672734845,55.104724217109,99.9662540836333)) ;
#9407=CARTESIAN_POINT('Ctrl Pts',(25.7569323765141,48.6398835186857,103.148284411731)) ;
#9408=CARTESIAN_POINT('Ctrl Pts',(26.2971586435828,48.4398363968329,103.113029503144)) ;
#9409=CARTESIAN_POINT('Ctrl Pts',(26.8319085774414,48.2402511072952,103.015193960956)) ;
#9410=CARTESIAN_POINT('Ctrl Pts',(27.9052437457281,47.8311034847338,102.686568200856)) ;
#9411=CARTESIAN_POINT('Ctrl Pts',(28.4381823878521,47.6231197022397,102.447937978474)) ;
#9412=CARTESIAN_POINT('Ctrl Pts',(29.755590053916,47.0862681322598,101.647310522153)) ;
#9413=CARTESIAN_POINT('Ctrl Pts',(30.4702215873772,46.7703270771007,100.982603468591)) ;
#9414=CARTESIAN_POINT('Ctrl Pts',(31.545074951219,46.2216257312612,99.4520955884149)) ;
#9415=CARTESIAN_POINT('Ctrl Pts',(31.920053706703,45.9879058539332,98.6179275795044)) ;
#9416=CARTESIAN_POINT('Ctrl Pts',(32.2740982535239,45.6640068779433,97.0725188928857)) ;
#9417=CARTESIAN_POINT('Ctrl Pts',(32.3302213337266,45.5539383973837,96.3954399628129)) ;
#9418=CARTESIAN_POINT('Ctrl Pts',(32.2496293109684,45.4179657782124,95.134669592589)) ;
#9419=CARTESIAN_POINT('Ctrl Pts',(32.1396710614035,45.3830586252741,94.557669561118)) ;
#9420=CARTESIAN_POINT('Ctrl Pts',(31.9584809790255,45.3830586252741,94.000023827484)) ;
#9421=CARTESIAN_POINT('Origin',(25.3010853649595,45.3822493559848,96.1631427881087)) ;
#9422=CARTESIAN_POINT('',(25.7569323765141,45.3822493559848,103.148284411731)) ;
#9423=CARTESIAN_POINT('Origin',(23.47768801576,45.3822493559848,68.2224337400009)) ;
#9424=CARTESIAN_POINT('',(8.73523672734845,45.3822493559848,99.9662540836333)) ;
#9425=CARTESIAN_POINT('Origin',(11.6837149504503,45.3822493559848,93.6175159280709)) ;
#9426=CARTESIAN_POINT('',(6.29012224935737,45.3822493559848,89.1555480018396)) ;
#9427=CARTESIAN_POINT('Origin',(18.7740766870781,45.3822493559848,74.0650393632132)) ;
#9428=CARTESIAN_POINT('Ctrl Pts',(18.7107542394381,57.826549970365,74.1415830535878)) ;
#9429=CARTESIAN_POINT('Ctrl Pts',(18.7107226067175,57.8721147557093,74.1416212909784)) ;
#9430=CARTESIAN_POINT('Ctrl Pts',(18.708092508703,57.9184467892871,74.1448005333832)) ;
#9431=CARTESIAN_POINT('Ctrl Pts',(18.6973298341945,58.006695871061,74.1578103720089)) ;
#9432=CARTESIAN_POINT('Ctrl Pts',(18.6890653833466,58.0508719526447,74.1678003769401)) ;
#9433=CARTESIAN_POINT('Ctrl Pts',(18.66602343776,58.1278680024908,74.1956533045249)) ;
#9434=CARTESIAN_POINT('Ctrl Pts',(18.6527112796475,58.1579990081032,74.2117449394387)) ;
#9435=CARTESIAN_POINT('Ctrl Pts',(18.6298766097115,58.1911673829066,74.2393473138024)) ;
#9436=CARTESIAN_POINT('Ctrl Pts',(18.6208888935898,58.2011153712953,74.2502115962984)) ;
#9437=CARTESIAN_POINT('Ctrl Pts',(18.6025171726295,58.2136587167219,74.272419192076)) ;
#9438=CARTESIAN_POINT('Ctrl Pts',(18.593643669708,58.2169692427703,74.2831454145369)) ;
#9439=CARTESIAN_POINT('Ctrl Pts',(18.5844571388615,58.2172758076351,74.2942500227594)) ;
#9440=CARTESIAN_POINT('Ctrl Pts',(18.5858591957557,58.3830247512599,74.2925552271096)) ;
#9441=CARTESIAN_POINT('Ctrl Pts',(18.5903405925418,58.3830247228371,74.2871381489514)) ;
#9442=CARTESIAN_POINT('Ctrl Pts',(18.5947855070738,58.3837424765035,74.2817651702627)) ;
#9443=CARTESIAN_POINT('Ctrl Pts',(18.6038618438227,58.3866521090648,74.2707937638226)) ;
#9444=CARTESIAN_POINT('Ctrl Pts',(18.6084152748266,58.3889169428568,74.2652896112528)) ;
#9445=CARTESIAN_POINT('Ctrl Pts',(18.6229204567539,58.3985444430684,74.2477558582845)) ;
#9446=CARTESIAN_POINT('Ctrl Pts',(18.6320253163883,58.4085611720381,74.2367499735612)) ;
#9447=CARTESIAN_POINT('Ctrl Pts',(18.6544021729805,58.4411881110096,74.2097010004657)) ;
#9448=CARTESIAN_POINT('Ctrl Pts',(18.6672182435102,58.4701790972226,74.1942090324728)) ;
#9449=CARTESIAN_POINT('Ctrl Pts',(18.6896541908679,58.5450324120245,74.167088630912)) ;
#9450=CARTESIAN_POINT('Ctrl Pts',(18.6977191225924,58.5884045334883,74.1573398030111)) ;
#9451=CARTESIAN_POINT('Ctrl Pts',(18.7082226594837,58.6752752681701,74.144643207955)) ;
#9452=CARTESIAN_POINT('Ctrl Pts',(18.710754102308,58.721038685503,74.1415832193495)) ;
#9453=CARTESIAN_POINT('Ctrl Pts',(18.7107539231051,58.7660385537516,74.1415834359687)) ;
#9454=CARTESIAN_POINT('Ctrl Pts',(18.5483450846703,58.2943663992286,74.2649701337207)) ;
#9455=CARTESIAN_POINT('Ctrl Pts',(18.6732965800537,58.2924602039142,74.1136194276355)) ;
#9456=CARTESIAN_POINT('Ctrl Pts',(18.5454318956407,58.191081348463,74.0045483675006)) ;
#9457=CARTESIAN_POINT('Ctrl Pts',(18.8016527608616,57.752299968185,74.4716103680308)) ;
#9458=CARTESIAN_POINT('Ctrl Pts',(18.9202592219973,57.7503889244304,74.31502434924)) ;
#9459=CARTESIAN_POINT('Ctrl Pts',(18.7878340776408,57.6489874075623,74.2113221384691)) ;
#9460=CARTESIAN_POINT('Ctrl Pts',(19.0675721711253,57.2111033102809,74.6619872725778)) ;
#9461=CARTESIAN_POINT('Ctrl Pts',(19.1795133398185,57.2091968025493,74.5005686455089)) ;
#9462=CARTESIAN_POINT('Ctrl Pts',(19.0428275223573,57.1078632090634,74.4024821086413)) ;
#9463=CARTESIAN_POINT('Ctrl Pts',(19.4822900636562,56.3997926693349,74.9212423510824)) ;
#9464=CARTESIAN_POINT('Ctrl Pts',(19.5838324114684,56.3978864499649,74.7532373532317)) ;
#9465=CARTESIAN_POINT('Ctrl Pts',(19.4413748489443,56.2965290900091,74.6639725606601)) ;
#9466=CARTESIAN_POINT('Ctrl Pts',(19.6233067304825,56.1295297083821,75.0033649035992)) ;
#9467=CARTESIAN_POINT('Ctrl Pts',(19.7213132030636,56.1276240321501,74.8332713211198)) ;
#9468=CARTESIAN_POINT('Ctrl Pts',(19.5770458564908,56.0262125668604,74.7470223626232)) ;
#9469=CARTESIAN_POINT('Ctrl Pts',(19.9102397208812,55.5885108130449,75.1586127326548)) ;
#9470=CARTESIAN_POINT('Ctrl Pts',(20.0010453943668,55.586605550614,74.9845706865102)) ;
#9471=CARTESIAN_POINT('Ctrl Pts',(19.8532587941722,55.4852720162805,74.9044079068786)) ;
#9472=CARTESIAN_POINT('Ctrl Pts',(20.0560810388402,55.3179011606656,75.231708743013)) ;
#9473=CARTESIAN_POINT('Ctrl Pts',(20.1432282407444,55.3159940909541,75.055805915533)) ;
#9474=CARTESIAN_POINT('Ctrl Pts',(19.9938011163935,55.2146518759856,74.9787548834564)) ;
#9475=CARTESIAN_POINT('Ctrl Pts',(20.352530228535,54.7764805321452,75.3688135322997)) ;
#9476=CARTESIAN_POINT('Ctrl Pts',(20.4322399575503,54.7745728258514,75.1894144826555)) ;
#9477=CARTESIAN_POINT('Ctrl Pts',(20.2797798149369,54.673110454093,75.1187172652187)) ;
#9478=CARTESIAN_POINT('Ctrl Pts',(20.5031363980417,54.5052712784276,75.4327965800233)) ;
#9479=CARTESIAN_POINT('Ctrl Pts',(20.5790612867906,54.5033650628295,75.2517668182727)) ;
#9480=CARTESIAN_POINT('Ctrl Pts',(20.4250872640913,54.4020271817646,75.1842528618848)) ;
#9481=CARTESIAN_POINT('Ctrl Pts',(20.8073844976248,53.963881271126,75.5509243276279)) ;
#9482=CARTESIAN_POINT('Ctrl Pts',(20.8756702730153,53.9619749130767,75.3668762682082)) ;
#9483=CARTESIAN_POINT('Ctrl Pts',(20.7190207758772,53.8606102461995,75.305868774962)) ;
#9484=CARTESIAN_POINT('Ctrl Pts',(20.9613691600088,53.6935003223872,75.6052113061699)) ;
#9485=CARTESIAN_POINT('Ctrl Pts',(21.0257878867995,53.6915946089085,75.4197734669531)) ;
#9486=CARTESIAN_POINT('Ctrl Pts',(20.8679145757183,53.5901950776532,75.3620650643573)) ;
#9487=CARTESIAN_POINT('Ctrl Pts',(21.2722115036904,53.1525885953719,75.7039526161564)) ;
#9488=CARTESIAN_POINT('Ctrl Pts',(21.3288198886603,53.150683235797,75.5159851220233)) ;
#9489=CARTESIAN_POINT('Ctrl Pts',(21.168635977305,53.0493503316648,75.4649147748249)) ;
#9490=CARTESIAN_POINT('Ctrl Pts',(21.4290379841683,52.8821999703398,75.7484084510137)) ;
#9491=CARTESIAN_POINT('Ctrl Pts',(21.4817073897842,52.8802927777274,75.5592990080604)) ;
#9492=CARTESIAN_POINT('Ctrl Pts',(21.3204986044484,52.7789455602911,75.5115909288728)) ;
#9493=CARTESIAN_POINT('Ctrl Pts',(21.7455028833639,52.34155747258,75.8274862850819)) ;
#9494=CARTESIAN_POINT('Ctrl Pts',(21.7902223538765,52.3396495857205,75.6363372625247)) ;
#9495=CARTESIAN_POINT('Ctrl Pts',(21.6272322413106,52.2381712237465,75.5954312381129)) ;
#9496=CARTESIAN_POINT('Ctrl Pts',(21.9050535263985,52.0708923183297,75.8620748678819)) ;
#9497=CARTESIAN_POINT('Ctrl Pts',(21.9457586711354,52.0689860211318,75.6700346895836)) ;
#9498=CARTESIAN_POINT('Ctrl Pts',(21.7818685831244,51.9676510264301,75.6325282562937)) ;
#9499=CARTESIAN_POINT('Ctrl Pts',(22.2260740470942,51.5294526417416,75.921184684073)) ;
#9500=CARTESIAN_POINT('Ctrl Pts',(22.2587094058815,51.5275461441382,75.7276087174543)) ;
#9501=CARTESIAN_POINT('Ctrl Pts',(22.0934146827021,51.4261734609838,75.696996712368)) ;
#9502=CARTESIAN_POINT('Ctrl Pts',(22.3878904045578,51.2584285629873,75.9457535234147)) ;
#9503=CARTESIAN_POINT('Ctrl Pts',(22.416456657201,51.2565228090173,75.7515349229333)) ;
#9504=CARTESIAN_POINT('Ctrl Pts',(22.2505651295337,51.1551340723535,75.7243991118759)) ;
#9505=CARTESIAN_POINT('Ctrl Pts',(22.712114476026,50.7168256229722,75.9845992195019)) ;
#9506=CARTESIAN_POINT('Ctrl Pts',(22.7325252779384,50.7149201642429,75.7893564712939)) ;
#9507=CARTESIAN_POINT('Ctrl Pts',(22.5656118445195,50.6135869790189,75.769183509045)) ;
#9508=CARTESIAN_POINT('Ctrl Pts',(22.8746038558045,50.4462620313528,75.9989086646007)) ;
#9509=CARTESIAN_POINT('Ctrl Pts',(22.8909288083536,50.4443547062682,75.8032814399391)) ;
#9510=CARTESIAN_POINT('Ctrl Pts',(22.7236412533748,50.3430015532564,75.7866059993292)) ;
#9511=CARTESIAN_POINT('Ctrl Pts',(23.200335139236,49.9056099882949,76.0173280779025)) ;
#9512=CARTESIAN_POINT('Ctrl Pts',(23.2084676499439,49.9037019096726,75.8211857194506)) ;
#9513=CARTESIAN_POINT('Ctrl Pts',(23.0407104726203,49.8022062837629,75.8115271717256)) ;
#9514=CARTESIAN_POINT('Ctrl Pts',(23.3634257556432,49.6350408217839,76.0214196212264)) ;
#9515=CARTESIAN_POINT('Ctrl Pts',(23.3674505868088,49.6331344368352,75.8251542835963)) ;
#9516=CARTESIAN_POINT('Ctrl Pts',(23.1994351681766,49.5318014383597,75.8190003897153)) ;
#9517=CARTESIAN_POINT('Ctrl Pts',(23.6894762533187,49.0942250306786,76.0193813810723)) ;
#9518=CARTESIAN_POINT('Ctrl Pts',(23.6852957248443,49.092318386207,75.8231180356694)) ;
#9519=CARTESIAN_POINT('Ctrl Pts',(23.5171978570909,48.9909365753488,75.8239920330866)) ;
#9520=CARTESIAN_POINT('Ctrl Pts',(23.8526613974115,48.8238179925217,76.013242383314)) ;
#9521=CARTESIAN_POINT('Ctrl Pts',(23.8443723781408,48.8219121926012,75.8171095821339)) ;
#9522=CARTESIAN_POINT('Ctrl Pts',(23.6763279800096,48.7205331729422,75.821501992585)) ;
#9523=CARTESIAN_POINT('Ctrl Pts',(24.1782986668665,48.2823982253296,75.9907308384264)) ;
#9524=CARTESIAN_POINT('Ctrl Pts',(24.1618100373473,48.2804926625387,75.7951178126276)) ;
#9525=CARTESIAN_POINT('Ctrl Pts',(23.9940710595387,48.1791582422039,75.8065384791858)) ;
#9526=CARTESIAN_POINT('Ctrl Pts',(24.3408658244874,48.0114576298608,75.9743576213341)) ;
#9527=CARTESIAN_POINT('Ctrl Pts',(24.3202852562274,48.0095520696295,75.7791284959206)) ;
#9528=CARTESIAN_POINT('Ctrl Pts',(24.1529117568251,47.9080609643498,75.7940537064683)) ;
#9529=CARTESIAN_POINT('Ctrl Pts',(24.6648859953999,47.4697670852043,75.9313851632708)) ;
#9530=CARTESIAN_POINT('Ctrl Pts',(24.6361421055437,47.4678622559149,75.737193617338)) ;
#9531=CARTESIAN_POINT('Ctrl Pts',(24.4694621780701,47.3665093096488,75.7591266505605)) ;
#9532=CARTESIAN_POINT('Ctrl Pts',(24.8258807196733,47.1991192501834,75.9048568447549)) ;
#9533=CARTESIAN_POINT('Ctrl Pts',(24.7930818640022,47.1972127705253,75.7113096559819)) ;
#9534=CARTESIAN_POINT('Ctrl Pts',(24.6268855561176,47.0958808570305,75.7367272449909)) ;
#9535=CARTESIAN_POINT('Ctrl Pts',(25.1458531545381,46.6582159321068,75.8417831790114)) ;
#9536=CARTESIAN_POINT('Ctrl Pts',(25.1049928075486,46.6563091331506,75.6497745295534)) ;
#9537=CARTESIAN_POINT('Ctrl Pts',(24.9400382258872,46.5549171221349,75.6821115969087)) ;
#9538=CARTESIAN_POINT('Ctrl Pts',(25.30494646225,46.3878930438263,75.8052019711465)) ;
#9539=CARTESIAN_POINT('Ctrl Pts',(25.2600759105256,46.3859871917113,75.6140912947864)) ;
#9540=CARTESIAN_POINT('Ctrl Pts',(25.0958217439246,46.284617201445,75.649875303476)) ;
#9541=CARTESIAN_POINT('Ctrl Pts',(25.6202833300099,45.8470089936472,75.7222021278697)) ;
#9542=CARTESIAN_POINT('Ctrl Pts',(25.5674638607462,45.845103318913,75.5331348858038)) ;
#9543=CARTESIAN_POINT('Ctrl Pts',(25.4048302998281,45.7437666877396,75.575757312238)) ;
#9544=CARTESIAN_POINT('Ctrl Pts',(25.7766280265348,45.5765948766363,75.6757691159531)) ;
#9545=CARTESIAN_POINT('Ctrl Pts',(25.719868519592,45.5746876690806,75.4878440205586)) ;
#9546=CARTESIAN_POINT('Ctrl Pts',(25.5581897868318,45.4732994150165,75.5338518072996)) ;
#9547=CARTESIAN_POINT('Ctrl Pts',(25.931588121197,45.3060601767044,75.6243964515729)) ;
#9548=CARTESIAN_POINT('Ctrl Pts',(25.8709204598157,45.3041537286489,75.4377421295873)) ;
#9549=CARTESIAN_POINT('Ctrl Pts',(25.710296883923,45.2027271666488,75.4871056281043)) ;
#9550=CARTESIAN_POINT('Ctrl Pts',(26.0863976142602,45.1993067880441,75.5689330654432)) ;
#9551=CARTESIAN_POINT('Ctrl Pts',(26.0220932596633,45.2022941676425,75.38578662784)) ;
#9552=CARTESIAN_POINT('Ctrl Pts',(26.1774539338622,45.3026134137914,75.3267467952831)) ;
#9553=CARTESIAN_POINT('Ctrl Pts',(25.9256608515516,45.4820412744497,75.62601128439)) ;
#9554=CARTESIAN_POINT('Ctrl Pts',(25.865362711039,45.4850270679879,75.4414566098922)) ;
#9555=CARTESIAN_POINT('Ctrl Pts',(26.0220178563139,45.5853439255572,75.3858152824602)) ;
#9556=CARTESIAN_POINT('Ctrl Pts',(25.7634007076745,45.7643410734524,75.677684307806)) ;
#9557=CARTESIAN_POINT('Ctrl Pts',(25.7071510922706,45.7673274764235,75.4918604580629)) ;
#9558=CARTESIAN_POINT('Ctrl Pts',(25.8650267437967,45.8675609242127,75.4396377628776)) ;
#9559=CARTESIAN_POINT('Ctrl Pts',(25.4365228584406,46.3280183067178,75.7701628739833)) ;
#9560=CARTESIAN_POINT('Ctrl Pts',(25.3884194289408,46.3310049155781,75.5820650392191)) ;
#9561=CARTESIAN_POINT('Ctrl Pts',(25.5484108731406,46.4312549192326,75.536770822617)) ;
#9562=CARTESIAN_POINT('Ctrl Pts',(25.2716852659958,46.609335596205,75.8110255869744)) ;
#9563=CARTESIAN_POINT('Ctrl Pts',(25.227688531219,46.6123217179243,75.6219236471007)) ;
#9564=CARTESIAN_POINT('Ctrl Pts',(25.3886032840335,46.7126174787231,75.5801309568726)) ;
#9565=CARTESIAN_POINT('Ctrl Pts',(24.9401111780303,47.1717937445101,75.8818362706009)) ;
#9566=CARTESIAN_POINT('Ctrl Pts',(24.9043789784248,47.1747789756424,75.6910024575541)) ;
#9567=CARTESIAN_POINT('Ctrl Pts',(25.0669976654131,47.2750030883893,75.6562349436383)) ;
#9568=CARTESIAN_POINT('Ctrl Pts',(24.7734305499936,47.4527838881785,75.9117853151364)) ;
#9569=CARTESIAN_POINT('Ctrl Pts',(24.7418488874936,47.4557718390911,75.7202204583389)) ;
#9570=CARTESIAN_POINT('Ctrl Pts',(24.9051764209183,47.5560106521802,75.6889957400452)) ;
#9571=CARTESIAN_POINT('Ctrl Pts',(24.4382874723605,48.0142871287959,75.9608038245404)) ;
#9572=CARTESIAN_POINT('Ctrl Pts',(24.4150496664146,48.0172768213996,75.768044108176)) ;
#9573=CARTESIAN_POINT('Ctrl Pts',(24.5795009866196,48.1176560532572,75.7439548245032)) ;
#9574=CARTESIAN_POINT('Ctrl Pts',(24.269958730186,48.2952668191079,75.9798400629779)) ;
#9575=CARTESIAN_POINT('Ctrl Pts',(24.250919768841,48.2982535238078,75.7866256771499)) ;
#9576=CARTESIAN_POINT('Ctrl Pts',(24.4159420948042,48.3984774868592,75.7661011315856)) ;
#9577=CARTESIAN_POINT('Ctrl Pts',(23.9324843805748,48.8569739450404,76.0069197948193)) ;
#9578=CARTESIAN_POINT('Ctrl Pts',(23.9218485613817,48.8599612929863,75.8130594689155)) ;
#9579=CARTESIAN_POINT('Ctrl Pts',(24.0875772524104,48.9602369845976,75.799720427907)) ;
#9580=CARTESIAN_POINT('Ctrl Pts',(23.7630925057922,49.1378578224385,76.0149733475353)) ;
#9581=CARTESIAN_POINT('Ctrl Pts',(23.7566759997451,49.1408439739377,75.8209278031086)) ;
#9582=CARTESIAN_POINT('Ctrl Pts',(23.9226618863959,49.2411084827015,75.8111948341747)) ;
#9583=CARTESIAN_POINT('Ctrl Pts',(23.4241550653974,49.7002903800858,76.0200135779628)) ;
#9584=CARTESIAN_POINT('Ctrl Pts',(23.4261790755229,49.703276075074,75.8258737420784)) ;
#9585=CARTESIAN_POINT('Ctrl Pts',(23.592451809069,49.8035038746523,75.8233630227755)) ;
#9586=CARTESIAN_POINT('Ctrl Pts',(23.2545251031872,49.9815741041393,76.0170168575449)) ;
#9587=CARTESIAN_POINT('Ctrl Pts',(23.2607689883619,49.9845603796949,75.8229622257759)) ;
#9588=CARTESIAN_POINT('Ctrl Pts',(23.4269824796514,50.084920629536,75.8240701185917)) ;
#9589=CARTESIAN_POINT('Ctrl Pts',(22.9149982686695,50.5452598054651,75.9998797474338)) ;
#9590=CARTESIAN_POINT('Ctrl Pts',(22.9296979857808,50.5482445256842,75.8062861236819)) ;
#9591=CARTESIAN_POINT('Ctrl Pts',(23.0957758973726,50.6484794514056,75.8146395997979)) ;
#9592=CARTESIAN_POINT('Ctrl Pts',(22.7454660608442,50.8275371605747,75.9857636870294)) ;
#9593=CARTESIAN_POINT('Ctrl Pts',(22.7643842449477,50.8305243023702,75.7925368283109)) ;
#9594=CARTESIAN_POINT('Ctrl Pts',(22.9302473046794,50.9307473367347,75.8045130352185)) ;
#9595=CARTESIAN_POINT('Ctrl Pts',(22.4915165114997,51.2516112326304,75.9561999963104)) ;
#9596=CARTESIAN_POINT('Ctrl Pts',(22.5167536338216,51.2545984104416,75.763729312436)) ;
#9597=CARTESIAN_POINT('Ctrl Pts',(22.6820674732779,51.3548887142751,75.7811302146028)) ;
#9598=CARTESIAN_POINT('Ctrl Pts',(22.406841155564,51.3931523912311,75.9449323425022)) ;
#9599=CARTESIAN_POINT('Ctrl Pts',(22.434185480836,51.3961391935531,75.7527491069979)) ;
#9600=CARTESIAN_POINT('Ctrl Pts',(22.5992892067911,51.4964465475109,75.77195900654)) ;
#9601=CARTESIAN_POINT('Ctrl Pts',(22.2380774216862,51.6761627264457,75.919643988823)) ;
#9602=CARTESIAN_POINT('Ctrl Pts',(22.2696228165867,51.6791488679009,75.7281072912384)) ;
#9603=CARTESIAN_POINT('Ctrl Pts',(22.4342963723503,51.7794030062205,75.7509296120974)) ;
#9604=CARTESIAN_POINT('Ctrl Pts',(22.1539868343232,51.8176028378155,75.9056277281354)) ;
#9605=CARTESIAN_POINT('Ctrl Pts',(22.1876248225326,51.8205891355633,75.7144479277084)) ;
#9606=CARTESIAN_POINT('Ctrl Pts',(22.3520464638859,51.9208298261597,75.7390706210171)) ;
#9607=CARTESIAN_POINT('Ctrl Pts',(21.9025850641051,52.2417288193263,75.8594804930087)) ;
#9608=CARTESIAN_POINT('Ctrl Pts',(21.9424783701571,52.2447151365766,75.6694719008893)) ;
#9609=CARTESIAN_POINT('Ctrl Pts',(22.1060334622313,52.3449566194381,75.6994758960422)) ;
#9610=CARTESIAN_POINT('Ctrl Pts',(21.7360305487315,52.5241300049792,75.8232269920363)) ;
#9611=CARTESIAN_POINT('Ctrl Pts',(21.7800665820217,52.5271161389007,75.6341332124948)) ;
#9612=CARTESIAN_POINT('Ctrl Pts',(21.9428878891998,52.6274277787848,75.6676973569287)) ;
#9613=CARTESIAN_POINT('Ctrl Pts',(21.4057304837302,53.0891744812252,75.7399061920707)) ;
#9614=CARTESIAN_POINT('Ctrl Pts',(21.4579849498291,53.0921595377542,75.552919602523)) ;
#9615=CARTESIAN_POINT('Ctrl Pts',(21.6192326546544,53.1923844744817,75.5935737756274)) ;
#9616=CARTESIAN_POINT('Ctrl Pts',(21.2421056534695,53.3716654702888,75.6928812421765)) ;
#9617=CARTESIAN_POINT('Ctrl Pts',(21.2984281526556,53.3746531995856,75.5070791947283)) ;
#9618=CARTESIAN_POINT('Ctrl Pts',(21.4587454410097,53.4748857690477,75.5512442980755)) ;
#9619=CARTESIAN_POINT('Ctrl Pts',(20.9179077319592,53.9365848433119,75.5880960700119)) ;
#9620=CARTESIAN_POINT('Ctrl Pts',(20.9822904856432,53.9395741566644,75.4049263975121)) ;
#9621=CARTESIAN_POINT('Ctrl Pts',(21.1404564827692,54.0399343658719,75.4560318818304)) ;
#9622=CARTESIAN_POINT('Ctrl Pts',(20.7574078709364,54.2194050938411,75.5303438342495)) ;
#9623=CARTESIAN_POINT('Ctrl Pts',(20.8257847793342,54.2223916877142,75.3486320539804)) ;
#9624=CARTESIAN_POINT('Ctrl Pts',(20.9828673359832,54.322617765037,75.4032076168567)) ;
#9625=CARTESIAN_POINT('Ctrl Pts',(20.4404376642166,54.7853172885882,75.4043970887111)) ;
#9626=CARTESIAN_POINT('Ctrl Pts',(20.5166947213234,54.7883043793635,75.225847521315)) ;
#9627=CARTESIAN_POINT('Ctrl Pts',(20.6712193285801,54.8885704141613,75.2872321944973)) ;
#9628=CARTESIAN_POINT('Ctrl Pts',(20.2837973428701,55.0683374452493,75.3361184767196)) ;
#9629=CARTESIAN_POINT('Ctrl Pts',(20.3639489350762,55.07132357191,75.1592827459495)) ;
#9630=CARTESIAN_POINT('Ctrl Pts',(20.5170877424361,55.1715968138496,75.2240365555281)) ;
#9631=CARTESIAN_POINT('Ctrl Pts',(19.9759898322398,55.6338317486207,75.1897533276409)) ;
#9632=CARTESIAN_POINT('Ctrl Pts',(20.0637929682781,55.636817283455,75.0165911195765)) ;
#9633=CARTESIAN_POINT('Ctrl Pts',(20.2139803198389,55.7370429277458,75.0879860149741)) ;
#9634=CARTESIAN_POINT('Ctrl Pts',(19.8246910607917,55.9162154787288,75.1116345999751)) ;
#9635=CARTESIAN_POINT('Ctrl Pts',(19.9162531085382,55.9192018043292,74.9404246400929)) ;
#9636=CARTESIAN_POINT('Ctrl Pts',(20.0647700907842,56.0195762764982,75.0150453656116)) ;
#9637=CARTESIAN_POINT('Ctrl Pts',(19.5271637169588,56.4812254904619,74.9454381365164)) ;
#9638=CARTESIAN_POINT('Ctrl Pts',(19.6261205413857,56.4842101348273,74.7783984369201)) ;
#9639=CARTESIAN_POINT('Ctrl Pts',(19.7713027695013,56.5844490941092,74.8594729793997)) ;
#9640=CARTESIAN_POINT('Ctrl Pts',(19.3813158328695,56.7637439358551,74.8575775464296)) ;
#9641=CARTESIAN_POINT('Ctrl Pts',(19.4838949469898,56.7667309512119,74.6927382117415)) ;
#9642=CARTESIAN_POINT('Ctrl Pts',(19.6272799015428,56.8669533046052,74.7769691201447)) ;
#9643=CARTESIAN_POINT('Ctrl Pts',(19.095442866224,57.3288079962577,74.6723447445499)) ;
#9644=CARTESIAN_POINT('Ctrl Pts',(19.2051226735476,57.3317959922188,74.5121391388438)) ;
#9645=CARTESIAN_POINT('Ctrl Pts',(19.3446542775862,57.4320972450331,74.6025284739922)) ;
#9646=CARTESIAN_POINT('Ctrl Pts',(18.9553476788922,57.6115036704006,74.574907756248)) ;
#9647=CARTESIAN_POINT('Ctrl Pts',(19.0685079296873,57.6144899220291,74.4171434179548)) ;
#9648=CARTESIAN_POINT('Ctrl Pts',(19.206054842789,57.7147356136766,74.5105810395141)) ;
#9649=CARTESIAN_POINT('Ctrl Pts',(18.6818459265001,58.1775332618958,74.3710420390506)) ;
#9650=CARTESIAN_POINT('Ctrl Pts',(18.8017978488122,58.1805194049365,74.2183781834203)) ;
#9651=CARTESIAN_POINT('Ctrl Pts',(18.9351306118037,58.2807563670214,74.3177449426027)) ;
#9652=CARTESIAN_POINT('Ctrl Pts',(18.5483121501979,58.4605262973907,74.2645110032067)) ;
#9653=CARTESIAN_POINT('Ctrl Pts',(18.6715801956769,58.463511044069,74.1145080753123)) ;
#9654=CARTESIAN_POINT('Ctrl Pts',(18.8026553177914,58.563858734355,74.2167324991218)) ;
#9655=CARTESIAN_POINT('Ctrl Pts',(18.4187092424426,58.7433256931628,74.1539683873054)) ;
#9656=CARTESIAN_POINT('Ctrl Pts',(18.5451935747115,58.7463119239391,74.006735167518)) ;
#9657=CARTESIAN_POINT('Ctrl Pts',(18.6740364880035,58.846513767945,74.1118252195922)) ;
#10288=UNCERTAINTY_MEASURE_WITH_UNIT(LENGTH_MEASURE(0.001),#10335,
'DISTANCE_ACCURACY_VALUE',
'Maximum model space distance between geometric entities at asserted c
onnectivities') ;
#10297=UNCERTAINTY_MEASURE_WITH_UNIT(LENGTH_MEASURE(0.001),#10335,
'DISTANCE_ACCURACY_VALUE',
'Maximum model space distance between geometric entities at asserted c
onnectivities') ;
#10325=(
GEOMETRIC_REPRESENTATION_CONTEXT(3)
GLOBAL_UNCERTAINTY_ASSIGNED_CONTEXT((#10288))
GLOBAL_UNIT_ASSIGNED_CONTEXT((#10335,#10337,#10338))
REPRESENTATION_CONTEXT('','3D')
) ;
#10334=(
GEOMETRIC_REPRESENTATION_CONTEXT(3)
GLOBAL_UNCERTAINTY_ASSIGNED_CONTEXT((#10297))
GLOBAL_UNIT_ASSIGNED_CONTEXT((#10335,#10337,#10338))
REPRESENTATION_CONTEXT('','3D')
) ;
#10335=(
LENGTH_UNIT()
NAMED_UNIT(*)
SI_UNIT(.CENTI.,.METRE.)
) ;
#10337=(
NAMED_UNIT(*)
PLANE_ANGLE_UNIT()
SI_UNIT($,.RADIAN.)
) ;
#10338=(
NAMED_UNIT(*)
SI_UNIT($,.STERADIAN.)
SOLID_ANGLE_UNIT()
) ;
#10366=SHAPE_DEFINITION_REPRESENTATION(#10426,#10473) ;
#10426=PRODUCT_DEFINITION_SHAPE('',$,#10510) ;
#10473=SHAPE_REPRESENTATION('',(#4086),#10325) ;
#10482=PRODUCT_DEFINITION_CONTEXT('part definition',#10592,'design') ;
#10510=PRODUCT_DEFINITION('Impeller','Impeller',#10546,#10482) ;
#10546=PRODUCT_DEFINITION_FORMATION('',$,#10621) ;
#10592=APPLICATION_CONTEXT(
'Core Data for Automotive Mechanical Design Process') ;
#10593=PRODUCT_CONTEXT('part definition',#10592,'mechanical') ;
#10621=PRODUCT('Impeller','Impeller',$,(#10593)) ;
#10633=PRESENTATION_STYLE_ASSIGNMENT((#10637)) ;
#10637=SURFACE_STYLE_USAGE(.BOTH.,#10641) ;
#10641=SURFACE_SIDE_STYLE('',(#10645)) ;
#10645=SURFACE_STYLE_FILL_AREA(#10649) ;
#10649=FILL_AREA_STYLE('Opaque(232,173,35)',(#10653)) ;
#10653=FILL_AREA_STYLE_COLOUR('Opaque(232,173,35)',#10657) ;
#10657=COLOUR_RGB('Opaque(232,173,35)', 0.09019608, 0.27058824, 0.51372549) ;
ENDSEC;
END-ISO-10303-21;
